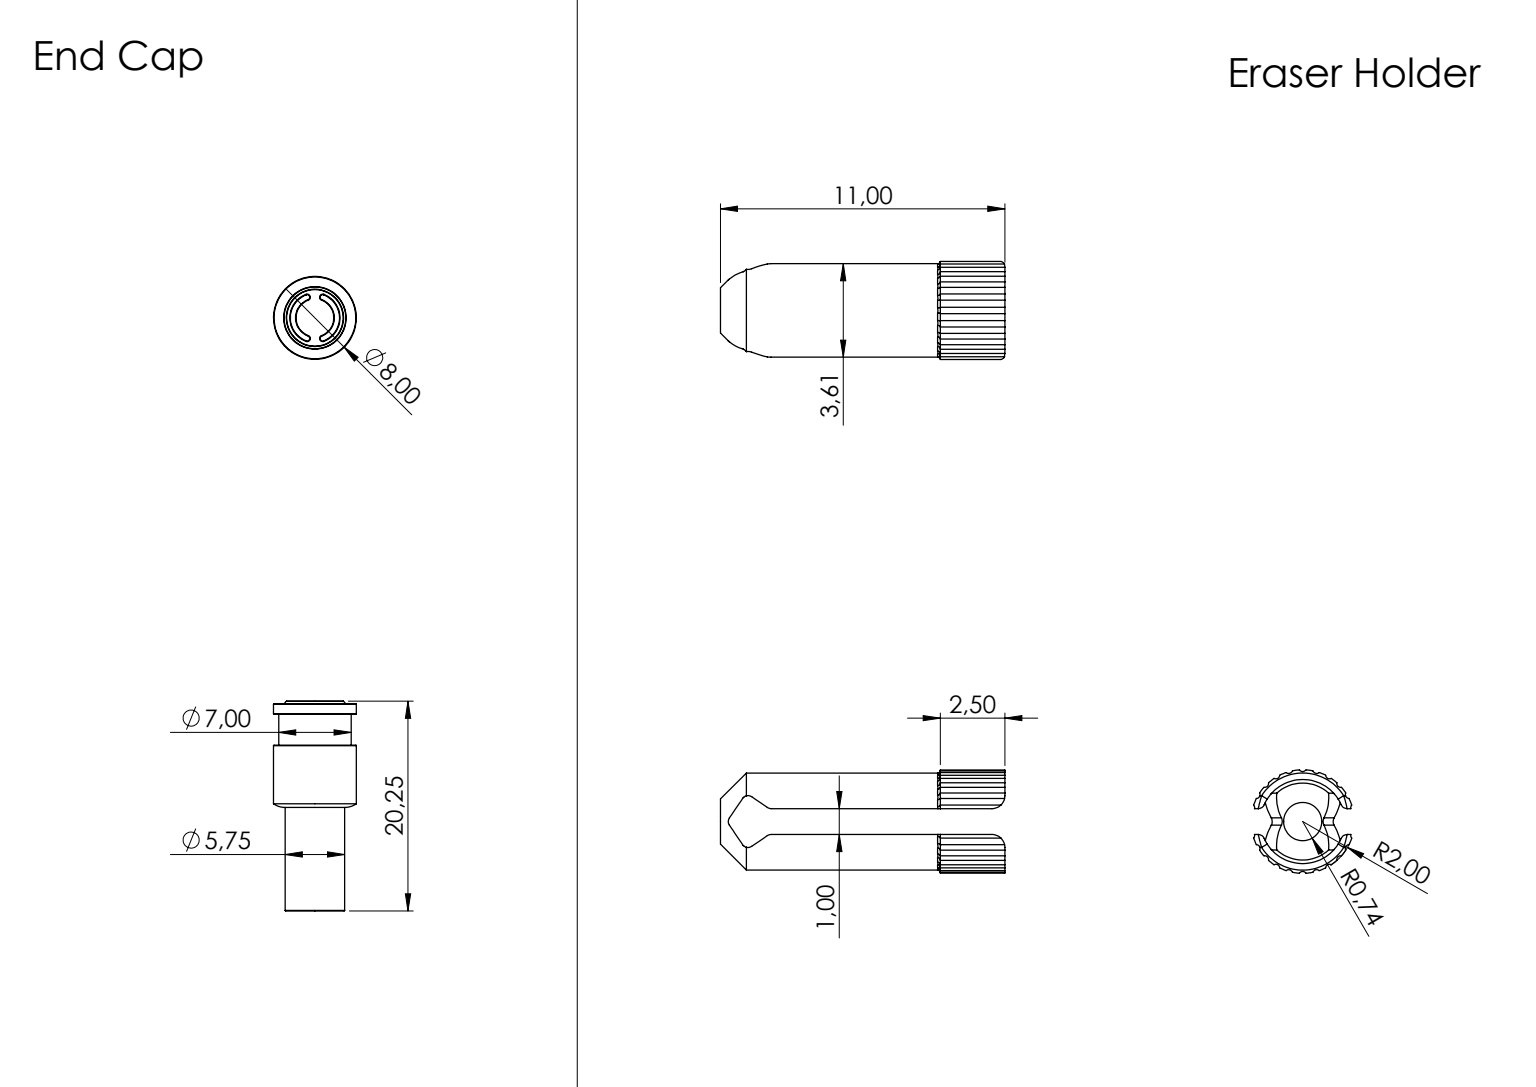
ISO-10303-21;
HEADER;
FILE_DESCRIPTION (('STEP AP214'),
    '1' );
FILE_NAME ('Eraser Holder.step',
    '2026-10-06T14:00:01',
    ( '' ),
    ( '' ),
    'SwSTEP 2.0',
    'SolidWorks 2020',
    '' );
FILE_SCHEMA (( 'AUTOMOTIVE_DESIGN' ));
ENDSEC;

DATA;
#15=CARTESIAN_POINT ( 'NONE',  ( 61.23770293223015670, -0.8897917884444476178, 1.791164585743103999 ) ) ;
#18=ORIENTED_EDGE ( 'NONE', *, *, #4179, .T. ) ;
#19=CARTESIAN_POINT ( 'NONE',  ( 58.72419296898095809, -1.822284191842195256, 0.4419487341019822102 ) ) ;
#25=ORIENTED_EDGE ( 'NONE', *, *, #30906, .F. ) ;
#36=VERTEX_POINT ( 'NONE', #5192 ) ;
#42=CARTESIAN_POINT ( 'NONE',  ( 60.81599023037216512, -0.4999999999993630651, -1.863080903343643291 ) ) ;
#52=ORIENTED_EDGE ( 'NONE', *, *, #16574, .F. ) ;
#60=DIRECTION ( 'NONE',  ( 1.000000000000000000, 1.047444401652940007E-14, -0.000000000000000000 ) ) ;
#62=EDGE_CURVE ( 'NONE', #4204, #12232, #6428, .T. ) ;
#67=VERTEX_POINT ( 'NONE', #29413 ) ;
#84=B_SPLINE_CURVE_WITH_KNOTS ( 'NONE', 3,
 ( #27085, #16988, #10017, #5408 ),
 .UNSPECIFIED., .F., .F.,
 ( 4, 4 ),
 ( 0.000000000000000000, 2.862003379465075675E-05 ),
 .UNSPECIFIED. ) ;
#90=CARTESIAN_POINT ( 'NONE',  ( 61.24891880570161362, -0.9671362613607715764, -1.669082548205986116 ) ) ;
#91=VERTEX_POINT ( 'NONE', #17714 ) ;
#93=VECTOR ( 'NONE', #18197, 1000.000000000000000 ) ;
#104=EDGE_LOOP ( 'NONE', ( #2125, #11645, #5974, #22411, #4642 ) ) ;
#118=CARTESIAN_POINT ( 'NONE',  ( 58.65817410504259044, 0.5270377936603326541, 1.799623063671935475 ) ) ;
#124=PLANE ( 'NONE',  #26575 ) ;
#126=CARTESIAN_POINT ( 'NONE',  ( 61.25000000000002132, 6.415596960124259844E-13, 3.111507638930570854E-58 ) ) ;
#136=CARTESIAN_POINT ( 'NONE',  ( 58.75000000000003553, -1.895722432252946010, 0.6373668173470157239 ) ) ;
#139=DIRECTION ( 'NONE',  ( 0.000000000000000000, 0.000000000000000000, 1.000000000000000000 ) ) ;
#145=CARTESIAN_POINT ( 'NONE',  ( 58.65000000000003411, -1.394635017527761311, -1.253243060177727131 ) ) ;
#162=CARTESIAN_POINT ( 'NONE',  ( 58.75000000000001421, 0.5933779550744251452, 1.867062706146590756 ) ) ;
#164=ORIENTED_EDGE ( 'NONE', *, *, #3455, .T. ) ;
#165=CARTESIAN_POINT ( 'NONE',  ( 58.75000018803721247, -1.882836145342761780, 0.4533061784681521322 ) ) ;
#166=LINE ( 'NONE', #7453, #15603 ) ;
#168=CARTESIAN_POINT ( 'NONE',  ( 51.64333574538936489, -0.8318165372340011743, -1.569663068107119974 ) ) ;
#173=CARTESIAN_POINT ( 'NONE',  ( 51.41326833096621129, -0.9846823677975790057, -1.426744987257088315 ) ) ;
#177=ORIENTED_EDGE ( 'NONE', *, *, #3546, .F. ) ;
#181=CARTESIAN_POINT ( 'NONE',  ( 58.74999999999980815, -1.394635017527639409, -1.253243060177863466 ) ) ;
#182=EDGE_CURVE ( 'NONE', #17885, #28405, #12945, .T. ) ;
#195=ORIENTED_EDGE ( 'NONE', *, *, #1967, .T. ) ;
#198=DIRECTION ( 'NONE',  ( 0.000000000000000000, 0.4531102586347437455, 0.8914544820235946743 ) ) ;
#203=VERTEX_POINT ( 'NONE', #8511 ) ;
#204=AXIS2_PLACEMENT_3D ( 'NONE', #12059, #22191, #17129 ) ;
#207=VERTEX_POINT ( 'NONE', #28132 ) ;
#212=B_SPLINE_CURVE_WITH_KNOTS ( 'NONE', 3,
 ( #23853, #28760, #23704, #11809, #1994, #9613, #29059, #26699, #21656, #24001, #19271, #11968, #26052 ),
 .UNSPECIFIED., .F., .F.,
 ( 4, 3, 3, 3, 4 ),
 ( 0.000000000000000000, 3.429247765843156239E-05, 6.861252194981137440E-05, 0.0001025118211733701013, 0.0001105094600589245180 ),
 .UNSPECIFIED. ) ;
#217=ADVANCED_FACE ( 'NONE', ( #691 ), #11323, .F. ) ;
#219=CIRCLE ( 'NONE', #12340, 2.000000000000000000 ) ;
#223=PLANE ( 'NONE',  #2312 ) ;
#224=CARTESIAN_POINT ( 'NONE',  ( 58.75000000000000000, 2.008165151418601191, 0.5380862305919300592 ) ) ;
#232=CARTESIAN_POINT ( 'NONE',  ( 58.66133336607628479, 1.875011749337246014, -0.03256983989501838900 ) ) ;
#233=DIRECTION ( 'NONE',  ( 1.000000000000000000, 1.047444401652940007E-14, 0.000000000000000000 ) ) ;
#238=FACE_OUTER_BOUND ( 'NONE', #13734, .T. ) ;
#243=AXIS2_PLACEMENT_3D ( 'NONE', #15272, #24917, #10208 ) ;
#245=AXIS2_PLACEMENT_3D ( 'NONE', #26689, #7358, #17036 ) ;
#249=DIRECTION ( 'NONE',  ( 1.000000000000000000, 1.047444401652940007E-14, 0.000000000000000000 ) ) ;
#262=PLANE ( 'NONE',  #2851 ) ;
#268=ORIENTED_EDGE ( 'NONE', *, *, #4535, .F. ) ;
#270=CARTESIAN_POINT ( 'NONE',  ( 51.50435016707359637, -0.9265794315402092751, -1.339215852266876672 ) ) ;
#272=VECTOR ( 'NONE', #16238, 1000.000000000000000 ) ;
#275=( BOUNDED_SURFACE ( )  B_SPLINE_SURFACE ( 3, 2, ( 
 ( #24839, #13578, #27853 ),
 ( #16132, #30851, #18355 ),
 ( #9002, #13880, #21051 ),
 ( #20886, #11544, #16291 ),
 ( #27992, #25934, #28322 ),
 ( #8822, #3767, #18511 ),
 ( #25783, #1876, #23266 ),
 ( #13729, #20588, #1550 ),
 ( #30222, #8528, #28153 ),
 ( #11213, #23111, #18831 ) ),
 .UNSPECIFIED., .F., .F., .T. ) 
 B_SPLINE_SURFACE_WITH_KNOTS ( ( 4, 2, 2, 2, 4 ),
 ( 3, 3 ),
 ( 0.0001706658715693258458, 0.0002229276920778027425, 0.0002751895125862796393, 0.0003274513330947565631, 0.0003797131536032334869 ),
 ( 0.000000000000000000, 1.000000000000000000 ),
 .UNSPECIFIED. ) 
 GEOMETRIC_REPRESENTATION_ITEM ( )  RATIONAL_B_SPLINE_SURFACE ( (
 ( 1.000000000000000000, 0.7071067811865444641, 1.000000000000000000),
 ( 1.000000000000000000, 0.7375607040701035455, 1.000000000000000000),
 ( 1.000000000000000000, 0.7730431127426561355, 1.000000000000000000),
 ( 1.000000000000000000, 0.8321012486983990764, 1.000000000000000000),
 ( 1.000000000000000000, 0.8541932017405543531, 1.000000000000000000),
 ( 1.000000000000000000, 0.8545723906055556762, 1.000000000000000000),
 ( 1.000000000000000000, 0.8327032135045047134, 1.000000000000000000),
 ( 1.000000000000000000, 0.7734559727062164658, 1.000000000000000000),
 ( 1.000000000000000000, 0.7377766653995503354, 1.000000000000000000),
 ( 1.000000000000000000, 0.7071067811865452413, 1.000000000000000000) ) ) 
 REPRESENTATION_ITEM ( '' )  SURFACE ( )  );
#276=ORIENTED_EDGE ( 'NONE', *, *, #13970, .F. ) ;
#283=DIRECTION ( 'NONE',  ( 0.000000000000000000, 0.9985773570672645816, 0.05332224631949589871 ) ) ;
#284=ADVANCED_FACE ( 'NONE', ( #30591 ), #18007, .F. ) ;
#286=CARTESIAN_POINT ( 'NONE',  ( 50.25000000000002132, 5.263408118306026973E-13, 3.111507638930570854E-58 ) ) ;
#295=CARTESIAN_POINT ( 'NONE',  ( 58.75000000000003553, -1.655311165516605509, -1.077297519404007753 ) ) ;
#297=ORIENTED_EDGE ( 'NONE', *, *, #11149, .T. ) ;
#299=AXIS2_PLACEMENT_3D ( 'NONE', #16364, #4639, #26010 ) ;
#310=CARTESIAN_POINT ( 'NONE',  ( 58.72427158855736451, -1.798991944511769470, 0.5288318043114524913 ) ) ;
#311=AXIS2_PLACEMENT_3D ( 'NONE', #27449, #5763, #15416 ) ;
#314=FACE_OUTER_BOUND ( 'NONE', #22953, .T. ) ;
#316=CARTESIAN_POINT ( 'NONE',  ( 58.74472430272383150, -0.4999999999993849364, -1.853787220596752272 ) ) ;
#321=CARTESIAN_POINT ( 'NONE',  ( 51.78416995154975666, -0.8999235898776958287, -1.360374659026170718 ) ) ;
#322=AXIS2_PLACEMENT_3D ( 'NONE', #6296, #16124, #30840 ) ;
#335=CIRCLE ( 'NONE', #10516, 1.875000000000001776 ) ;
#345=CIRCLE ( 'NONE', #29674, 0.1500000000000001887 ) ;
#346=CARTESIAN_POINT ( 'NONE',  ( 58.66133336607573057, -1.802692578418147118, 0.5167488000325648478 ) ) ;
#359=CIRCLE ( 'NONE', #3392, 1.975000000000001865 ) ;
#360=DIRECTION ( 'NONE',  ( 1.000000000000000000, 1.047444401652940007E-14, 0.000000000000000000 ) ) ;
#366=ORIENTED_EDGE ( 'NONE', *, *, #22608, .F. ) ;
#367=DIRECTION ( 'NONE',  ( 1.000000000000000000, 1.047444401652940007E-14, 0.000000000000000000 ) ) ;
#370=ADVANCED_FACE ( 'NONE', ( #29150 ), #19356, .F. ) ;
#379=AXIS2_PLACEMENT_3D ( 'NONE', #22161, #7586, #5825 ) ;
#382=ORIENTED_EDGE ( 'NONE', *, *, #29422, .T. ) ;
#383=CARTESIAN_POINT ( 'NONE',  ( 51.89360908398760586, 0.6611756245550776123, -1.497563819580874922 ) ) ;
#385=CARTESIAN_POINT ( 'NONE',  ( 58.72427158855720819, -0.9764256747734804120, -1.600821037878335185 ) ) ;
#388=CARTESIAN_POINT ( 'NONE',  ( 51.18802626461298644, 0.9696678249730820154, 1.452003249885708946 ) ) ;
#389=CIRCLE ( 'NONE', #18100, 0.1000000000000000749 ) ;
#392=CARTESIAN_POINT ( 'NONE',  ( 58.75000000000002842, -1.077297519403676906, 1.655311165517035166 ) ) ;
#394=CARTESIAN_POINT ( 'NONE',  ( 51.17290532404582137, 0.9646187004851747293, 1.462925393634774363 ) ) ;
#398=CARTESIAN_POINT ( 'NONE',  ( 61.24637336955063915, -0.9388313581414567954, -1.688008567904763835 ) ) ;
#401=ORIENTED_EDGE ( 'NONE', *, *, #30815, .F. ) ;
#406=DIRECTION ( 'NONE',  ( 1.000000000000000000, 1.047444401652940007E-14, 0.000000000000000000 ) ) ;
#408=ORIENTED_EDGE ( 'NONE', *, *, #18853, .F. ) ;
#414=CIRCLE ( 'NONE', #1347, 1.875000000000001776 ) ;
#423=CARTESIAN_POINT ( 'NONE',  ( 51.45655683570189609, 0.9591657938401617622, -1.518428463906025705 ) ) ;
#425=AXIS2_PLACEMENT_3D ( 'NONE', #10899, #22657, #18053 ) ;
#431=LINE ( 'NONE', #17079, #18420 ) ;
#436=ORIENTED_EDGE ( 'NONE', *, *, #1318, .F. ) ;
#442=CARTESIAN_POINT ( 'NONE',  ( 58.75000000000001421, 0.5380862305905714793, 2.008165151419250449 ) ) ;
#443=ADVANCED_FACE ( 'NONE', ( #24852 ), #20138, .T. ) ;
#445=DIRECTION ( 'NONE',  ( -1.000000000000000000, -1.047444401652940007E-14, -0.000000000000000000 ) ) ;
#456=CARTESIAN_POINT ( 'NONE',  ( 51.84831113588977303, -0.6920605891655385866, -1.653603923793142361 ) ) ;
#457=ORIENTED_EDGE ( 'NONE', *, *, #26462, .T. ) ;
#465=EDGE_LOOP ( 'NONE', ( #3537, #28913, #30616, #5077 ) ) ;
#466=CIRCLE ( 'NONE', #9064, 0.1499999999999998557 ) ;
#477=CARTESIAN_POINT ( 'NONE',  ( 58.75000000000002132, 6.153735859711025284E-13, 3.111507638930570854E-58 ) ) ;
#482=ORIENTED_EDGE ( 'NONE', *, *, #30906, .T. ) ;
#490=CIRCLE ( 'NONE', #22257, 2.000000000000000000 ) ;
#493=DIRECTION ( 'NONE',  ( 1.000000000000000000, 1.047444401652940007E-14, 0.000000000000000000 ) ) ;
#507=VERTEX_POINT ( 'NONE', #5861 ) ;
#511=CARTESIAN_POINT ( 'NONE',  ( 50.25000000000002842, -0.6373668173474561494, 1.895722432253304168 ) ) ;
#521=ORIENTED_EDGE ( 'NONE', *, *, #12297, .F. ) ;
#528=DIRECTION ( 'NONE',  ( 0.000000000000000000, 0.000000000000000000, 1.000000000000000000 ) ) ;
#535=CARTESIAN_POINT ( 'NONE',  ( 61.25000000000004263, -1.960427193528290424, -0.3958853607747112036 ) ) ;
#543=DIRECTION ( 'NONE',  ( 1.000000000000000000, 1.047444401652940007E-14, 0.000000000000000000 ) ) ;
#545=CARTESIAN_POINT ( 'NONE',  ( 58.72427158855708029, 1.293556822995456823, -1.357477749119827104 ) ) ;
#555=EDGE_LOOP ( 'NONE', ( #4647, #4798, #8077, #13774 ) ) ;
#574=DIRECTION ( 'NONE',  ( 0.000000000000000000, -1.154631945610163433E-14, 1.000000000000000000 ) ) ;
#575=DIRECTION ( 'NONE',  ( 1.000000000000000000, 1.047444401652940007E-14, 0.000000000000000000 ) ) ;
#585=VERTEX_POINT ( 'NONE', #11859 ) ;
#589=CARTESIAN_POINT ( 'NONE',  ( 51.23644008536124517, -1.080112125195908490, -1.214076932077872817 ) ) ;
#593=CIRCLE ( 'NONE', #14742, 0.09999999999999990841 ) ;
#595=CARTESIAN_POINT ( 'NONE',  ( 58.75000000000002132, 6.153735859711025284E-13, 3.111507638930570854E-58 ) ) ;
#599=ADVANCED_FACE ( 'NONE', ( #18369 ), #26110, .T. ) ;
#606=CARTESIAN_POINT ( 'NONE',  ( 52.06628335902946247, -0.5434431642975662280, -1.718465885608440713 ) ) ;
#620=CARTESIAN_POINT ( 'NONE',  ( 58.75000000000002132, 6.153735859711025284E-13, 3.111507638930570854E-58 ) ) ;
#624=VERTEX_POINT ( 'NONE', #28172 ) ;
#627=CYLINDRICAL_SURFACE ( 'NONE', #1476, 2.000000000000000000 ) ;
#628=ORIENTED_EDGE ( 'NONE', *, *, #25092, .T. ) ;
#631=DIRECTION ( 'NONE',  ( 0.000000000000000000, 0.000000000000000000, 1.000000000000000000 ) ) ;
#672=ORIENTED_EDGE ( 'NONE', *, *, #29291, .F. ) ;
#675=VECTOR ( 'NONE', #28976, 1000.000000000000000 ) ;
#691=FACE_OUTER_BOUND ( 'NONE', #7612, .T. ) ;
#695=CARTESIAN_POINT ( 'NONE',  ( 52.20711756518983293, 0.5000000000005468959, 1.807104036850122109 ) ) ;
#698=ORIENTED_EDGE ( 'NONE', *, *, #22851, .F. ) ;
#704=VERTEX_POINT ( 'NONE', #19468 ) ;
#716=AXIS2_PLACEMENT_3D ( 'NONE', #28481, #23120, #1884 ) ;
#719=B_SPLINE_CURVE_WITH_KNOTS ( 'NONE', 3,
 ( #22326, #2999, #17256, #24068, #2383, #12047, #21722, #16951, #26898, #14858, #7446, #7736, #15 ),
 .UNSPECIFIED., .F., .F.,
 ( 4, 3, 3, 3, 4 ),
 ( 0.000000000000000000, 4.969793434219683530E-05, 9.932084631989379544E-05, 0.0001499488332825447262, 0.0001857305951747128983 ),
 .UNSPECIFIED. ) ;
#755=CARTESIAN_POINT ( 'NONE',  ( 58.74999981404332061, 1.649595783783479375, -1.050697058760609037 ) ) ;
#756=DIRECTION ( 'NONE',  ( -0.000000000000000000, -0.000000000000000000, 1.000000000000000000 ) ) ;
#760=AXIS2_PLACEMENT_3D ( 'NONE', #23917, #2210, #11875 ) ;
#764=CARTESIAN_POINT ( 'NONE',  ( 50.25000000000001421, 0.5380862305914526633, -2.008165151417984351 ) ) ;
#771=EDGE_CURVE ( 'NONE', #11615, #8275, #12629, .T. ) ;
#773=DIRECTION ( 'NONE',  ( 0.000000000000000000, 0.000000000000000000, 1.000000000000000000 ) ) ;
#779=VERTEX_POINT ( 'NONE', #24051 ) ;
#783=VECTOR ( 'NONE', #2254, 1000.000000000000000 ) ;
#793=B_SPLINE_CURVE_WITH_KNOTS ( 'NONE', 3,
 ( #2578, #2877, #7631, #19681 ),
 .UNSPECIFIED., .F., .F.,
 ( 4, 4 ),
 ( 0.0001543670095910078732, 0.0003084486524517373977 ),
 .UNSPECIFIED. ) ;
#797=B_SPLINE_CURVE_WITH_KNOTS ( 'NONE', 3,
 ( #20697, #30322, #12903, #18305 ),
 .UNSPECIFIED., .F., .F.,
 ( 4, 4 ),
 ( 0.000000000000000000, 0.0003819718307412704175 ),
 .UNSPECIFIED. ) ;
#798=ORIENTED_EDGE ( 'NONE', *, *, #29211, .T. ) ;
#803=CIRCLE ( 'NONE', #9900, 0.1500000000000001887 ) ;
#805=DIRECTION ( 'NONE',  ( 0.000000000000000000, 1.000000000000000000, 0.000000000000000000 ) ) ;
#806=DIRECTION ( 'NONE',  ( 0.000000000000000000, 0.000000000000000000, 1.000000000000000000 ) ) ;
#810=CIRCLE ( 'NONE', #6376, 1.975000000000001865 ) ;
#822=ORIENTED_EDGE ( 'NONE', *, *, #25663, .T. ) ;
#823=CARTESIAN_POINT ( 'NONE',  ( 51.25000000000000711, 1.487500000000537836, 3.111507638930570854E-58 ) ) ;
#833=VERTEX_POINT ( 'NONE', #5999 ) ;
#835=ADVANCED_FACE ( 'NONE', ( #6144 ), #29926, .F. ) ;
#847=CIRCLE ( 'NONE', #15519, 0.1499999999999999667 ) ;
#848=CARTESIAN_POINT ( 'NONE',  ( 58.75000000000001421, 0.5811678240991637878, -1.782657835994492013 ) ) ;
#849=CYLINDRICAL_SURFACE ( 'NONE', #29409, 0.1499999999999999667 ) ;
#852=DIRECTION ( 'NONE',  ( 1.000000000000000000, 1.047444401652940007E-14, 0.000000000000000000 ) ) ;
#858=DIRECTION ( 'NONE',  ( 0.000000000000000000, 0.000000000000000000, 1.000000000000000000 ) ) ;
#861=CARTESIAN_POINT ( 'NONE',  ( 58.75000000000000711, 1.469015551797813846, -1.320082690053157037 ) ) ;
#869=CIRCLE ( 'NONE', #6936, 0.1500000000000001887 ) ;
#870=ORIENTED_EDGE ( 'NONE', *, *, #20028, .T. ) ;
#872=CIRCLE ( 'NONE', #8460, 1.975000000000001865 ) ;
#882=CARTESIAN_POINT ( 'NONE',  ( 51.59739104186226655, 1.010292945603182391, -1.272765950230260179 ) ) ;
#892=ADVANCED_FACE ( 'NONE', ( #25917 ), #30664, .F. ) ;
#906=ADVANCED_FACE ( 'NONE', ( #23399 ), #24657, .F. ) ;
#909=EDGE_CURVE ( 'NONE', #14419, #20284, #9225, .T. ) ;
#911=CARTESIAN_POINT ( 'NONE',  ( 50.56925576102500486, 0.1015751161705248512, 0.8011113709441619601 ) ) ;
#917=CARTESIAN_POINT ( 'NONE',  ( 58.75000000000001421, 0.5380862305905714793, 2.008165151419250449 ) ) ;
#919=CARTESIAN_POINT ( 'NONE',  ( 58.65000000000001990, 6.143261415694495821E-13, 3.111507638930570854E-58 ) ) ;
#923=ADVANCED_FACE ( 'NONE', ( #2011 ), #8804, .F. ) ;
#925=CARTESIAN_POINT ( 'NONE',  ( 58.65000000000001990, 6.143261415694495821E-13, 3.111507638930570854E-58 ) ) ;
#934=CARTESIAN_POINT ( 'NONE',  ( 51.64281244548085681, -0.8321733326261643304, 1.569379851958366601 ) ) ;
#935=EDGE_CURVE ( 'NONE', #17628, #18608, #7028, .T. ) ;
#939=ADVANCED_FACE ( 'NONE', ( #28303 ), #31138, .F. ) ;
#951=CARTESIAN_POINT ( 'NONE',  ( 51.12687253673781385, -0.9194130538815391551, 1.491219977510798600 ) ) ;
#954=ORIENTED_EDGE ( 'NONE', *, *, #13577, .T. ) ;
#957=MECHANICAL_DESIGN_GEOMETRIC_PRESENTATION_REPRESENTATION('',(#11070),#9033);
#967=EDGE_CURVE ( 'NONE', #12164, #18852, #27400, .T. ) ;
#978=CARTESIAN_POINT ( 'NONE',  ( 58.74999999305998699, -1.869977652031123094, -0.4744892162740728669 ) ) ;
#986=AXIS2_PLACEMENT_3D ( 'NONE', #6730, #26038, #21171 ) ;
#989=CARTESIAN_POINT ( 'NONE',  ( 58.75000000000000711, 1.039502773797200019, -1.800471618823823450 ) ) ;
#990=EDGE_LOOP ( 'NONE', ( #18643, #27738, #24622, #5621, #14527, #4921 ) ) ;
#993=CIRCLE ( 'NONE', #14134, 0.1000000000000000611 ) ;
#996=EDGE_LOOP ( 'NONE', ( #25581, #2177, #9610, #14667, #5663, #17467 ) ) ;
#997=CARTESIAN_POINT ( 'NONE',  ( 58.75000000000000711, 1.039502773796331159, 1.800471618825331355 ) ) ;
#998=CARTESIAN_POINT ( 'NONE',  ( 51.36308620441097617, 1.097739233406260118, -1.198394850649635357 ) ) ;
#1013=FACE_OUTER_BOUND ( 'NONE', #20174, .T. ) ;
#1014=CARTESIAN_POINT ( 'NONE',  ( 50.25000000000000000, 1.800471618824854181, -1.039502773795712987 ) ) ;
#1015=DIRECTION ( 'NONE',  ( 1.000000000000000000, 1.047444401652940007E-14, 0.000000000000000000 ) ) ;
#1016=CARTESIAN_POINT ( 'NONE',  ( 51.25000000000001421, 5.368152558471320595E-13, 3.111507638930570854E-58 ) ) ;
#1018=DIRECTION ( 'NONE',  ( -0.5633368246414943714, -0.8262273428075581627, 0.000000000000000000 ) ) ;
#1024=AXIS2_PLACEMENT_3D ( 'NONE', #23682, #18298, #6253 ) ;
#1030=CARTESIAN_POINT ( 'NONE',  ( 61.00000000000002132, 6.389410850082937196E-13, 3.111507638930570854E-58 ) ) ;
#1037=VERTEX_POINT ( 'NONE', #24332 ) ;
#1048=AXIS2_PLACEMENT_3D ( 'NONE', #10585, #8052, #2989 ) ;
#1050=DIRECTION ( 'NONE',  ( 1.000000000000000000, 1.047444401652940007E-14, 0.000000000000000000 ) ) ;
#1054=CARTESIAN_POINT ( 'NONE',  ( 51.25000000000001421, 5.368152558471320595E-13, 3.111507638930570854E-58 ) ) ;
#1058=CARTESIAN_POINT ( 'NONE',  ( 58.65000000000000568, 1.571497941946485177, 1.022750809562084306 ) ) ;
#1061=FACE_OUTER_BOUND ( 'NONE', #19043, .T. ) ;
#1062=ORIENTED_EDGE ( 'NONE', *, *, #27891, .F. ) ;
#1063=CARTESIAN_POINT ( 'NONE',  ( 58.75000000000000711, 1.932246131438033920, -0.4087173687832938995 ) ) ;
#1066=DIRECTION ( 'NONE',  ( -1.018631342913014973E-14, 1.000000000000000000, 0.000000000000000000 ) ) ;
#1067=DIRECTION ( 'NONE',  ( 0.000000000000000000, 0.000000000000000000, 1.000000000000000000 ) ) ;
#1072=CARTESIAN_POINT ( 'NONE',  ( 51.31572262954152563, 0.7526089581382734428, -1.996089927833914146 ) ) ;
#1075=DIRECTION ( 'NONE',  ( -0.8262273428075537218, 0.5633368246415009217, 0.000000000000000000 ) ) ;
#1079=FACE_OUTER_BOUND ( 'NONE', #31118, .T. ) ;
#1081=CARTESIAN_POINT ( 'NONE',  ( 51.84831113588978724, -0.6920605891655307040, 1.653603923793091068 ) ) ;
#1083=VERTEX_POINT ( 'NONE', #20221 ) ;
#1091=CARTESIAN_POINT ( 'NONE',  ( 58.75000000000002132, -0.4999999999991334154, 1.863080903344709549 ) ) ;
#1107=CARTESIAN_POINT ( 'NONE',  ( 58.74160516400056053, 1.017053542743361794, 1.575205926126844513 ) ) ;
#1114=ADVANCED_FACE ( 'NONE', ( #10373 ), #27630, .F. ) ;
#1121=DIRECTION ( 'NONE',  ( 1.000000000000000000, 1.047444401652940007E-14, 0.000000000000000000 ) ) ;
#1124=CARTESIAN_POINT ( 'NONE',  ( 58.75000000000003553, -1.760622601995984304, -0.8948927608036236769 ) ) ;
#1135=ORIENTED_EDGE ( 'NONE', *, *, #4031, .F. ) ;
#1138=ORIENTED_EDGE ( 'NONE', *, *, #28214, .F. ) ;
#1143=CARTESIAN_POINT ( 'NONE',  ( 58.64999999999999858, 1.671477153795419390, -0.8495817349390374362 ) ) ;
#1144=EDGE_LOOP ( 'NONE', ( #6591, #9871, #26617, #31163 ) ) ;
#1152=CARTESIAN_POINT ( 'NONE',  ( 61.20598745287978915, 0.7563774268569909420, 1.657497327209963345 ) ) ;
#1154=AXIS2_PLACEMENT_3D ( 'NONE', #9213, #7572, #17089 ) ;
#1164=ORIENTED_EDGE ( 'NONE', *, *, #8587, .T. ) ;
#1165=CARTESIAN_POINT ( 'NONE',  ( 51.98855675296391610, 0.7791495708613138671, -1.432971607104406520 ) ) ;
#1192=FACE_OUTER_BOUND ( 'NONE', #13084, .T. ) ;
#1196=DIRECTION ( 'NONE',  ( 1.000000000000000000, 1.047444401652940007E-14, 0.000000000000000000 ) ) ;
#1200=EDGE_LOOP ( 'NONE', ( #2742, #18519, #13836, #1367 ) ) ;
#1201=ADVANCED_FACE ( 'NONE', ( #11638 ), #13817, .T. ) ;
#1211=DIRECTION ( 'NONE',  ( 0.000000000000000000, 0.000000000000000000, -1.000000000000000000 ) ) ;
#1216=CARTESIAN_POINT ( 'NONE',  ( 58.73371041428912065, 1.662559130999850865, -0.8671977075788435130 ) ) ;
#1249=( BOUNDED_CURVE ( )  B_SPLINE_CURVE ( 3, ( #3855, #13504, #1165, #10822 ),
 .UNSPECIFIED., .F., .T. ) 
 B_SPLINE_CURVE_WITH_KNOTS ( ( 4, 4 ),
 ( 4.041453792691655167, 4.300872134317202722 ),
 .UNSPECIFIED. ) 
 CURVE ( )  GEOMETRIC_REPRESENTATION_ITEM ( )  RATIONAL_B_SPLINE_CURVE ( ( 1.000000000000000000, 0.9943997021150918769, 0.9943997021150918769, 1.000000000000000000 ) ) 
 REPRESENTATION_ITEM ( '' )  );
#1256=VERTEX_POINT ( 'NONE', #25406 ) ;
#1266=CARTESIAN_POINT ( 'NONE',  ( 58.64999999999999147, 1.827485639843792864, -0.4207625006677218060 ) ) ;
#1268=AXIS2_PLACEMENT_3D ( 'NONE', #6662, #6195, #11578 ) ;
#1269=ORIENTED_EDGE ( 'NONE', *, *, #8234, .T. ) ;
#1273=DIRECTION ( 'NONE',  ( 0.000000000000000000, 0.000000000000000000, 1.000000000000000000 ) ) ;
#1276=CARTESIAN_POINT ( 'NONE',  ( 61.25000000000000711, 1.499837071477986505, 1.323060376182421782 ) ) ;
#1288=CARTESIAN_POINT ( 'NONE',  ( 51.23644008536124517, -1.080112125195908490, -1.214076932077872817 ) ) ;
#1298=AXIS2_PLACEMENT_3D ( 'NONE', #4590, #28822, #21869 ) ;
#1300=CARTESIAN_POINT ( 'NONE',  ( 58.75000002382379449, 0.5510104498278126650, -1.849358057801673505 ) ) ;
#1301=CARTESIAN_POINT ( 'NONE',  ( 58.64999999999999147, 1.589751505945893095, 0.9947034709630272475 ) ) ;
#1313=CIRCLE ( 'NONE', #15983, 0.1000000000000000611 ) ;
#1316=ORIENTED_EDGE ( 'NONE', *, *, #1533, .F. ) ;
#1318=EDGE_CURVE ( 'NONE', #3662, #19841, #3554, .T. ) ;
#1320=FACE_OUTER_BOUND ( 'NONE', #25481, .T. ) ;
#1332=ORIENTED_EDGE ( 'NONE', *, *, #26822, .F. ) ;
#1333=AXIS2_PLACEMENT_3D ( 'NONE', #25103, #29529, #2954 ) ;
#1335=DIRECTION ( 'NONE',  ( 0.000000000000000000, 0.000000000000000000, 1.000000000000000000 ) ) ;
#1336=VERTEX_POINT ( 'NONE', #15758 ) ;
#1337=CARTESIAN_POINT ( 'NONE',  ( 61.09423418603945777, 0.6373668173466511266, 1.895722432253563516 ) ) ;
#1341=CARTESIAN_POINT ( 'NONE',  ( 51.89360908398611372, -0.6611756245528535025, -1.497563819582787614 ) ) ;
#1347=AXIS2_PLACEMENT_3D ( 'NONE', #24122, #26652, #2730 ) ;
#1349=CARTESIAN_POINT ( 'NONE',  ( 61.25000000000004263, -1.996089927834276301, 0.1250000000000018041 ) ) ;
#1352=CARTESIAN_POINT ( 'NONE',  ( 58.65000090395038512, -0.5493607500713694192, 1.793027323413614038 ) ) ;
#1356=AXIS2_PLACEMENT_3D ( 'NONE', #5359, #7596, #14714 ) ;
#1358=DIRECTION ( 'NONE',  ( 0.000000000000000000, 0.000000000000000000, -1.000000000000000000 ) ) ;
#1362=ORIENTED_EDGE ( 'NONE', *, *, #12297, .T. ) ;
#1364=EDGE_LOOP ( 'NONE', ( #23271, #3401, #8925, #4713 ) ) ;
#1367=ORIENTED_EDGE ( 'NONE', *, *, #7484, .F. ) ;
#1370=CARTESIAN_POINT ( 'NONE',  ( 60.87284881435256523, -0.5000000998561487942, 1.554802432719775362 ) ) ;
#1372=CIRCLE ( 'NONE', #30683, 0.1500000000000001887 ) ;
#1382=VERTEX_POINT ( 'NONE', #16713 ) ;
#1384=CARTESIAN_POINT ( 'NONE',  ( 58.75000000000000000, 1.871971993775707555, -0.6020210199447628696 ) ) ;
#1394=AXIS2_PLACEMENT_3D ( 'NONE', #286, #17550, #5511 ) ;
#1395=CIRCLE ( 'NONE', #10003, 0.1500000000000001887 ) ;
#1397=CARTESIAN_POINT ( 'NONE',  ( 61.09423418603945777, 0.6373668173466511266, 1.895722432253563516 ) ) ;
#1399=CARTESIAN_POINT ( 'NONE',  ( 58.66118217212479635, -1.874997884618849753, 0.01689491344058241529 ) ) ;
#1401=ORIENTED_EDGE ( 'NONE', *, *, #26434, .T. ) ;
#1405=CARTESIAN_POINT ( 'NONE',  ( 51.64837794009022076, -0.8283786772106969121, 1.688958810662479104 ) ) ;
#1407=CARTESIAN_POINT ( 'NONE',  ( 58.65000000000001990, 6.143261415694495821E-13, 3.111507638930570854E-58 ) ) ;
#1421=ORIENTED_EDGE ( 'NONE', *, *, #10213, .T. ) ;
#1431=CARTESIAN_POINT ( 'NONE',  ( 58.65000000000001990, 6.143261415694495821E-13, 3.111507638930570854E-58 ) ) ;
#1433=ORIENTED_EDGE ( 'NONE', *, *, #16160, .F. ) ;
#1435=CARTESIAN_POINT ( 'NONE',  ( 61.25000000000003553, -0.9999999999993586242, -1.586072192556190252 ) ) ;
#1436=( BOUNDED_SURFACE ( )  B_SPLINE_SURFACE ( 3, 2, ( 
 ( #15821, #3492, #3779 ),
 ( #13130, #1107, #22819 ),
 ( #21701, #26269, #23426 ),
 ( #18997, #4575, #30704 ),
 ( #12024, #14223, #21384 ),
 ( #26421, #16926, #31172 ),
 ( #9660, #23749, #4717 ),
 ( #14374, #23897, #30863 ),
 ( #21230, #14067, #31008 ),
 ( #19167, #7258, #2189 ) ),
 .UNSPECIFIED., .F., .F., .F. ) 
 B_SPLINE_SURFACE_WITH_KNOTS ( ( 4, 2, 2, 2, 4 ),
 ( 3, 3 ),
 ( 0.0001706658715694773631, 0.0002229276920777904640, 0.0002751895125861035648, 0.0003274513330944167199, 0.0003797131536027298208 ),
 ( 0.000000000000000000, 1.000000000000000000 ),
 .UNSPECIFIED. ) 
 GEOMETRIC_REPRESENTATION_ITEM ( )  RATIONAL_B_SPLINE_SURFACE ( (
 ( 1.000000000000000000, 0.7071067811865445751, 1.000000000000000000),
 ( 1.000000000000000000, 0.7375607040698810568, 1.000000000000000000),
 ( 1.000000000000000000, 0.7730431127426297122, 1.000000000000000000),
 ( 1.000000000000000000, 0.8321012486974134204, 1.000000000000000000),
 ( 1.000000000000000000, 0.8541932017392805943, 1.000000000000000000),
 ( 1.000000000000000000, 0.8545723906046818197, 1.000000000000000000),
 ( 1.000000000000000000, 0.8327032135036619431, 1.000000000000000000),
 ( 1.000000000000000000, 0.7734559727059460155, 1.000000000000000000),
 ( 1.000000000000000000, 0.7377766653993722556, 1.000000000000000000),
 ( 1.000000000000000000, 0.7071067811865451302, 1.000000000000000000) ) ) 
 REPRESENTATION_ITEM ( '' )  SURFACE ( )  );
#1443=CARTESIAN_POINT ( 'NONE',  ( 51.12687253673781385, -0.9194130538815391551, -1.491219977510798600 ) ) ;
#1448=ORIENTED_EDGE ( 'NONE', *, *, #2643, .F. ) ;
#1468=CIRCLE ( 'NONE', #23234, 1.975000000000001865 ) ;
#1472=CARTESIAN_POINT ( 'NONE',  ( 58.75000000000003553, -1.760622601995690983, -0.8948927608037045012 ) ) ;
#1476=AXIS2_PLACEMENT_3D ( 'NONE', #477, #10141, #11927 ) ;
#1478=VERTEX_POINT ( 'NONE', #4584 ) ;
#1480=DIRECTION ( 'NONE',  ( 0.000000000000000000, 0.000000000000000000, 1.000000000000000000 ) ) ;
#1484=CARTESIAN_POINT ( 'NONE',  ( 51.25000000000001421, 0.9938153758931693726, 1.589954715908409755 ) ) ;
#1487=CARTESIAN_POINT ( 'NONE',  ( 58.75000000000002132, 6.153735859711025284E-13, 3.111507638930570854E-58 ) ) ;
#1503=DIRECTION ( 'NONE',  ( 1.000000000000000000, 1.047444401652940007E-14, 0.000000000000000000 ) ) ;
#1505=EDGE_CURVE ( 'NONE', #16552, #4296, #28743, .T. ) ;
#1509=DIRECTION ( 'NONE',  ( 1.000000000000000000, 1.047444401652940007E-14, 0.000000000000000000 ) ) ;
#1523=CARTESIAN_POINT ( 'NONE',  ( 60.75000000000003553, -0.6499999999993626432, 1.489337100860685270 ) ) ;
#1525=ORIENTED_EDGE ( 'NONE', *, *, #13910, .F. ) ;
#1531=FACE_OUTER_BOUND ( 'NONE', #4571, .T. ) ;
#1532=CYLINDRICAL_SURFACE ( 'NONE', #17592, 0.2500000000000000000 ) ;
#1533=EDGE_CURVE ( 'NONE', #10001, #12097, #20968, .T. ) ;
#1537=CARTESIAN_POINT ( 'NONE',  ( 58.74999981404330640, 1.865327579934561664, -0.5879486190987924799 ) ) ;
#1542=PLANE ( 'NONE',  #8402 ) ;
#1550=CARTESIAN_POINT ( 'NONE',  ( 58.65266784251152643, 1.589569034372934730, 0.9945725797258593293 ) ) ;
#1551=ORIENTED_EDGE ( 'NONE', *, *, #3019, .F. ) ;
#1574=CARTESIAN_POINT ( 'NONE',  ( 61.23913277633455721, 0.8963220027434347648, -1.755758457445524279 ) ) ;
#1575=CARTESIAN_POINT ( 'NONE',  ( 61.25000000000004263, -2.008165151418346728, -0.5380862305909229759 ) ) ;
#1578=DIRECTION ( 'NONE',  ( 0.000000000000000000, 0.000000000000000000, 1.000000000000000000 ) ) ;
#1582=CARTESIAN_POINT ( 'NONE',  ( 50.25000000000004263, -1.960427193528665679, 0.3958853607747486181 ) ) ;
#1586=CARTESIAN_POINT ( 'NONE',  ( 58.65838214097832548, 1.819565423307722973, 0.4528606663879586880 ) ) ;
#1594=DIRECTION ( 'NONE',  ( 0.000000000000000000, 0.000000000000000000, 1.000000000000000000 ) ) ;
#1598=ORIENTED_EDGE ( 'NONE', *, *, #27228, .F. ) ;
#1603=ORIENTED_EDGE ( 'NONE', *, *, #30308, .T. ) ;
#1609=DIRECTION ( 'NONE',  ( 0.000000000000000000, 0.000000000000000000, 1.000000000000000000 ) ) ;
#1620=ORIENTED_EDGE ( 'NONE', *, *, #27872, .T. ) ;
#1625=ORIENTED_EDGE ( 'NONE', *, *, #27794, .F. ) ;
#1629=ORIENTED_EDGE ( 'NONE', *, *, #2077, .F. ) ;
#1633=CARTESIAN_POINT ( 'NONE',  ( 51.31943556899493331, 1.088761256244167086, -1.206353010735628395 ) ) ;
#1640=EDGE_LOOP ( 'NONE', ( #23576, #7511, #21638, #13636 ) ) ;
#1649=CARTESIAN_POINT ( 'NONE',  ( 58.73307976133193620, -0.5681412931372339381, 1.786904874453541181 ) ) ;
#1652=EDGE_CURVE ( 'NONE', #18954, #20483, #19935, .T. ) ;
#1656=DIRECTION ( 'NONE',  ( 1.000000000000000000, 1.047444401652940007E-14, 0.000000000000000000 ) ) ;
#1657=AXIS2_PLACEMENT_3D ( 'NONE', #30446, #11286, #18439 ) ;
#1660=ORIENTED_EDGE ( 'NONE', *, *, #10869, .F. ) ;
#1662=DIRECTION ( 'NONE',  ( 1.000000000000000000, 1.047444401652940007E-14, 0.000000000000000000 ) ) ;
#1663=EDGE_LOOP ( 'NONE', ( #16263, #15937, #26989, #11465 ) ) ;
#1667=CARTESIAN_POINT ( 'NONE',  ( 61.16418558922029547, -0.6863720863828340901, 1.477277441814885073 ) ) ;
#1671=ORIENTED_EDGE ( 'NONE', *, *, #20492, .F. ) ;
#1681=CARTESIAN_POINT ( 'NONE',  ( 51.21569492700663062, -0.9844681138054331981, -1.555342057744142359 ) ) ;
#1682=FACE_OUTER_BOUND ( 'NONE', #29942, .T. ) ;
#1685=CIRCLE ( 'NONE', #9284, 0.09999999999999997780 ) ;
#1686=DIRECTION ( 'NONE',  ( 0.000000000000000000, 0.000000000000000000, 1.000000000000000000 ) ) ;
#1701=CARTESIAN_POINT ( 'NONE',  ( 58.75000000000004263, -1.394635017527501075, 1.253243060178017121 ) ) ;
#1718=ORIENTED_EDGE ( 'NONE', *, *, #12779, .F. ) ;
#1722=DIRECTION ( 'NONE',  ( 0.000000000000000000, 0.000000000000000000, 1.000000000000000000 ) ) ;
#1725=ADVANCED_FACE ( 'NONE', ( #25449 ), #4036, .T. ) ;
#1726=EDGE_CURVE ( 'NONE', #25442, #19414, #7799, .T. ) ;
#1737=CARTESIAN_POINT ( 'NONE',  ( 58.74999981196283017, 1.865248186430322752, 0.5877861523419425360 ) ) ;
#1751=CYLINDRICAL_SURFACE ( 'NONE', #7892, 0.5000000000000000000 ) ;
#1763=FACE_OUTER_BOUND ( 'NONE', #1200, .T. ) ;
#1765=CARTESIAN_POINT ( 'NONE',  ( 60.88446240048056524, 0.5000000000006363798, 1.718465885608440491 ) ) ;
#1767=CARTESIAN_POINT ( 'NONE',  ( 51.25000000000001421, 5.368152558471320595E-13, 3.111507638930570854E-58 ) ) ;
#1773=CARTESIAN_POINT ( 'NONE',  ( 58.75000000694009827, -1.658042653848017300, -0.9860766835992956780 ) ) ;
#1781=ORIENTED_EDGE ( 'NONE', *, *, #7380, .T. ) ;
#1786=AXIS2_PLACEMENT_3D ( 'NONE', #8044, #17551, #27356 ) ;
#1792=CARTESIAN_POINT ( 'NONE',  ( 58.75000000000003553, -1.655311165516861083, 1.077297519403202175 ) ) ;
#1794=ORIENTED_EDGE ( 'NONE', *, *, #13176, .T. ) ;
#1795=CARTESIAN_POINT ( 'NONE',  ( 52.20711756518983293, 0.5000000000005468959, -1.996089927833914146 ) ) ;
#1801=ORIENTED_EDGE ( 'NONE', *, *, #3505, .F. ) ;
#1805=( BOUNDED_CURVE ( )  B_SPLINE_CURVE ( 3, ( #14575, #3006, #7288, #19798 ),
 .UNSPECIFIED., .F., .T. ) 
 B_SPLINE_CURVE_WITH_KNOTS ( ( 4, 4 ),
 ( 1.033802687944702203, 1.276740478505648868 ),
 .UNSPECIFIED. ) 
 CURVE ( )  GEOMETRIC_REPRESENTATION_ITEM ( )  RATIONAL_B_SPLINE_CURVE ( ( 1.000000000000000000, 0.9950878134350369386, 0.9950878134350369386, 1.000000000000000000 ) ) 
 REPRESENTATION_ITEM ( '' )  );
#1806=DIRECTION ( 'NONE',  ( 0.000000000000000000, 0.000000000000000000, 1.000000000000000000 ) ) ;
#1815=CARTESIAN_POINT ( 'NONE',  ( 58.75000000000003553, -1.323060376181095732, -1.499837071478052453 ) ) ;
#1816=CARTESIAN_POINT ( 'NONE',  ( 58.66118217212468267, -0.9228675180754075669, 1.632243256842505819 ) ) ;
#1818=AXIS2_PLACEMENT_3D ( 'NONE', #29013, #4951, #3037 ) ;
#1822=CIRCLE ( 'NONE', #12942, 0.1500000000000001887 ) ;
#1826=CIRCLE ( 'NONE', #7431, 0.1499999999999999667 ) ;
#1841=EDGE_LOOP ( 'NONE', ( #628, #26422, #5505, #21184 ) ) ;
#1847=EDGE_CURVE ( 'NONE', #27521, #23889, #26879, .T. ) ;
#1849=CARTESIAN_POINT ( 'NONE',  ( 58.72200624034154259, 1.816790722508793365, -0.4641018782086855921 ) ) ;
#1858=EDGE_CURVE ( 'NONE', #19651, #21772, #2734, .T. ) ;
#1875=EDGE_CURVE ( 'NONE', #10792, #18525, #6890, .T. ) ;
#1876=CARTESIAN_POINT ( 'NONE',  ( 58.72419296898070940, 1.601054456121395964, 0.9760445624818194776 ) ) ;
#1877=CIRCLE ( 'NONE', #6952, 0.1499999999999999667 ) ;
#1881=CARTESIAN_POINT ( 'NONE',  ( 58.74999981196286569, -1.441661833134154636, 1.321459237641457563 ) ) ;
#1882=VERTEX_POINT ( 'NONE', #15903 ) ;
#1883=ORIENTED_EDGE ( 'NONE', *, *, #21252, .T. ) ;
#1884=DIRECTION ( 'NONE',  ( 0.000000000000000000, 0.000000000000000000, 1.000000000000000000 ) ) ;
#1889=CIRCLE ( 'NONE', #379, 1.875000000000001776 ) ;
#1895=DIRECTION ( 'NONE',  ( 1.000000000000000000, 1.047444401652940007E-14, 0.000000000000000000 ) ) ;
#1897=EDGE_CURVE ( 'NONE', #17885, #10721, #16797, .T. ) ;
#1900=VERTEX_POINT ( 'NONE', #31101 ) ;
#1901=AXIS2_PLACEMENT_3D ( 'NONE', #24169, #2478, #12132 ) ;
#1906=DIRECTION ( 'NONE',  ( 1.000000000000000000, 1.047444401652940007E-14, 0.000000000000000000 ) ) ;
#1908=ADVANCED_FACE ( 'NONE', ( #12113 ), #20053, .F. ) ;
#1910=CARTESIAN_POINT ( 'NONE',  ( 58.75000000000002132, 6.153735859711025284E-13, 3.111507638930570854E-58 ) ) ;
#1915=CARTESIAN_POINT ( 'NONE',  ( 51.25000000000002842, -1.099999999999462963, -1.996089927833914146 ) ) ;
#1917=VECTOR ( 'NONE', #16680, 1000.000000000000000 ) ;
#1920=DIRECTION ( 'NONE',  ( -0.000000000000000000, -0.000000000000000000, -1.000000000000000000 ) ) ;
#1922=ORIENTED_EDGE ( 'NONE', *, *, #24349, .F. ) ;
#1926=AXIS2_PLACEMENT_3D ( 'NONE', #4634, #4487, #24276 ) ;
#1931=CARTESIAN_POINT ( 'NONE',  ( 58.75000000000000000, 1.972190280208565571, -0.1053114364790996016 ) ) ;
#1932=ORIENTED_EDGE ( 'NONE', *, *, #14326, .F. ) ;
#1937=EDGE_CURVE ( 'NONE', #28767, #12009, #26394, .T. ) ;
#1939=VERTEX_POINT ( 'NONE', #14316 ) ;
#1943=CARTESIAN_POINT ( 'NONE',  ( 58.75000000000003553, -1.800471618824714071, 1.039502773796719959 ) ) ;
#1952=CARTESIAN_POINT ( 'NONE',  ( 58.65000038048068376, -1.663933463835848059, -0.8644232797864647155 ) ) ;
#1958=FACE_OUTER_BOUND ( 'NONE', #27770, .T. ) ;
#1961=CARTESIAN_POINT ( 'NONE',  ( 60.75000000000001421, 0.6500000000006350698, -1.489337100860685048 ) ) ;
#1965=DIRECTION ( 'NONE',  ( 0.000000000000000000, 0.000000000000000000, 1.000000000000000000 ) ) ;
#1967=EDGE_CURVE ( 'NONE', #31291, #24125, #14030, .T. ) ;
#1968=CARTESIAN_POINT ( 'NONE',  ( 58.65266784251147669, -1.656109637134997703, 0.8793208749736606267 ) ) ;
#1974=CARTESIAN_POINT ( 'NONE',  ( 58.65000000000004121, -1.872332544500605378, 0.09997921184723741750 ) ) ;
#1985=ADVANCED_FACE ( 'NONE', ( #25225 ), #849, .F. ) ;
#1992=CARTESIAN_POINT ( 'NONE',  ( 51.25000000000001421, 5.368159983410797313E-13, 3.111507638930570854E-58 ) ) ;
#1994=CARTESIAN_POINT ( 'NONE',  ( 58.72153194576635826, 0.5000000000006150636, -1.827449685318863093 ) ) ;
#1998=DIRECTION ( 'NONE',  ( 1.000000000000000000, 0.000000000000000000, -0.000000000000000000 ) ) ;
#2011=FACE_OUTER_BOUND ( 'NONE', #28396, .T. ) ;
#2021=CARTESIAN_POINT ( 'NONE',  ( 58.75000000000000711, 1.932246131437593162, 0.4087173687853762338 ) ) ;
#2023=CARTESIAN_POINT ( 'NONE',  ( 61.23770293222972327, 0.8897917884438596436, 1.791164585743606041 ) ) ;
#2033=CARTESIAN_POINT ( 'NONE',  ( 58.74999999305997989, -1.345908541131179081, 1.382203543031325088 ) ) ;
#2034=VERTEX_POINT ( 'NONE', #8131 ) ;
#2035=EDGE_LOOP ( 'NONE', ( #12776, #23464, #28372, #21264 ) ) ;
#2038=EDGE_CURVE ( 'NONE', #2740, #15300, #22545, .T. ) ;
#2040=DIRECTION ( 'NONE',  ( 0.000000000000000000, 0.000000000000000000, 1.000000000000000000 ) ) ;
#2045=CARTESIAN_POINT ( 'NONE',  ( 61.25000000000001421, 1.000000000000641709, 1.546164609606623053 ) ) ;
#2047=CARTESIAN_POINT ( 'NONE',  ( 58.75000000000002132, 6.153735859711025284E-13, 3.111507638930570854E-58 ) ) ;
#2062=EDGE_CURVE ( 'NONE', #20216, #21772, #20343, .T. ) ;
#2067=CARTESIAN_POINT ( 'NONE',  ( 58.75000000000004263, -1.922112613533886405, 0.4146634982040790507 ) ) ;
#2075=ORIENTED_EDGE ( 'NONE', *, *, #28271, .T. ) ;
#2077=EDGE_CURVE ( 'NONE', #507, #20216, #12900, .T. ) ;
#2078=CARTESIAN_POINT ( 'NONE',  ( 58.68279620299848176, 0.5000000000006146195, 1.809045707182517004 ) ) ;
#2081=CARTESIAN_POINT ( 'NONE',  ( 58.75000018595667939, 1.936190688449842767, -0.04992417795777597672 ) ) ;
#2085=EDGE_LOOP ( 'NONE', ( #4934, #25212, #8117, #15158, #24252, #16329 ) ) ;
#2090=CARTESIAN_POINT ( 'NONE',  ( 51.49472959044967268, -1.070956530527746420, -1.224612562803250038 ) ) ;
#2092=CARTESIAN_POINT ( 'NONE',  ( 61.00000000000002132, 6.389410850082937196E-13, 3.111507638930570854E-58 ) ) ;
#2093=AXIS2_PLACEMENT_3D ( 'NONE', #6612, #10880, #6146 ) ;
#2115=EDGE_CURVE ( 'NONE', #19132, #7871, #593, .T. ) ;
#2117=ORIENTED_EDGE ( 'NONE', *, *, #14849, .F. ) ;
#2125=ORIENTED_EDGE ( 'NONE', *, *, #2514, .T. ) ;
#2126=VERTEX_POINT ( 'NONE', #535 ) ;
#2127=( BOUNDED_SURFACE ( )  B_SPLINE_SURFACE ( 3, 2, ( 
 ( #30225, #8531, #18217 ),
 ( #6167, #25465, #2181 ),
 ( #2348, #9172, #19159 ),
 ( #16770, #12014, #4411 ),
 ( #21696, #31161, #7415 ),
 ( #21222, #28798, #31320 ),
 ( #18835, #7110, #4243 ),
 ( #9496, #14540, #11546 ),
 ( #26414, #9787, #11847 ),
 ( #19455, #28639, #14060 ) ),
 .UNSPECIFIED., .F., .F., .F. ) 
 B_SPLINE_SURFACE_WITH_KNOTS ( ( 4, 2, 2, 2, 4 ),
 ( 3, 3 ),
 ( 0.0001706658715691171911, 0.0002229276920778207674, 0.0002751895125865243437, 0.0003274513330952279200, 0.0003797131536039315505 ),
 ( 0.000000000000000000, 1.000000000000000000 ),
 .UNSPECIFIED. ) 
 GEOMETRIC_REPRESENTATION_ITEM ( )  RATIONAL_B_SPLINE_SURFACE ( (
 ( 1.000000000000000000, 0.7071067811865445751, 1.000000000000000000),
 ( 1.000000000000000000, 0.7375607040702577555, 1.000000000000000000),
 ( 1.000000000000000000, 0.7730431127429812088, 1.000000000000000000),
 ( 1.000000000000000000, 0.8321012486994131541, 1.000000000000000000),
 ( 1.000000000000000000, 0.8541932017417729339, 1.000000000000000000),
 ( 1.000000000000000000, 0.8545723906072647535, 1.000000000000000000),
 ( 1.000000000000000000, 0.8327032135058914930, 1.000000000000000000),
 ( 1.000000000000000000, 0.7734559727064781454, 1.000000000000000000),
 ( 1.000000000000000000, 0.7377766653997793744, 1.000000000000000000),
 ( 1.000000000000000000, 0.7071067811865466846, 1.000000000000000000) ) ) 
 REPRESENTATION_ITEM ( '' )  SURFACE ( )  );
#2130=CARTESIAN_POINT ( 'NONE',  ( 58.75000000000002842, -0.8948927608030053937, -1.760622601996600922 ) ) ;
#2134=DIRECTION ( 'NONE',  ( -0.000000000000000000, -0.000000000000000000, -1.000000000000000000 ) ) ;
#2138=CARTESIAN_POINT ( 'NONE',  ( 51.47729133425610115, 0.9526829978902818796, 1.321356857234310178 ) ) ;
#2139=ADVANCED_FACE ( 'NONE', ( #29657 ), #17646, .F. ) ;
#2142=ADVANCED_FACE ( 'NONE', ( #18740 ), #25522, .F. ) ;
#2150=CARTESIAN_POINT ( 'NONE',  ( 58.75000000000002842, -1.039502773796102897, -1.800471618824325493 ) ) ;
#2156=DIRECTION ( 'NONE',  ( 1.000000000000000000, 1.047444401652940007E-14, 0.000000000000000000 ) ) ;
#2164=CARTESIAN_POINT ( 'NONE',  ( 51.14630318392394770, 0.9364487020639118420, -1.503522130792751987 ) ) ;
#2170=CARTESIAN_POINT ( 'NONE',  ( 51.31572262954153985, -0.7526089581371979698, -1.996089927833914146 ) ) ;
#2177=ORIENTED_EDGE ( 'NONE', *, *, #6013, .T. ) ;
#2181=CARTESIAN_POINT ( 'NONE',  ( 58.65000038048047060, 0.8644232797865400997, -1.663933463836744231 ) ) ;
#2182=CARTESIAN_POINT ( 'NONE',  ( 58.72200624034191208, -1.341335979946730816, 1.310319377727102497 ) ) ;
#2184=EDGE_LOOP ( 'NONE', ( #27777, #22817, #4422, #9131, #26467 ) ) ;
#2188=CARTESIAN_POINT ( 'NONE',  ( 58.65815574817776223, -0.5272471384221183444, 1.799565140951959963 ) ) ;
#2189=CARTESIAN_POINT ( 'NONE',  ( 58.65000000000000568, 0.8495817349399593654, 1.671477153794648896 ) ) ;
#2204=CARTESIAN_POINT ( 'NONE',  ( 58.75000000000000000, 2.079005547593415937, 1.004182178118534636E-12 ) ) ;
#2210=DIRECTION ( 'NONE',  ( 1.000000000000000000, 1.047444401652940007E-14, 0.000000000000000000 ) ) ;
#2212=EDGE_CURVE ( 'NONE', #29156, #28572, #6857, .T. ) ;
#2214=DIRECTION ( 'NONE',  ( -0.000000000000000000, -0.000000000000000000, -1.000000000000000000 ) ) ;
#2218=CARTESIAN_POINT ( 'NONE',  ( 51.25000000000002842, -1.099999999999462963, 1.196087371390569087 ) ) ;
#2223=ORIENTED_EDGE ( 'NONE', *, *, #30510, .T. ) ;
#2224=CARTESIAN_POINT ( 'NONE',  ( 51.35647303904148231, -1.001029238032807633, -1.398203054920482025 ) ) ;
#2225=EDGE_CURVE ( 'NONE', #29589, #67, #17282, .T. ) ;
#2228=CARTESIAN_POINT ( 'NONE',  ( 58.67159525762672700, 0.5000000000007230883, 1.807104036850089468 ) ) ;
#2230=LINE ( 'NONE', #11895, #29634 ) ;
#2231=EDGE_LOOP ( 'NONE', ( #12494, #26433, #20885, #23045, #6777, #24843 ) ) ;
#2236=ORIENTED_EDGE ( 'NONE', *, *, #11052, .T. ) ;
#2249=CIRCLE ( 'NONE', #12863, 1.625000000000000222 ) ;
#2254=DIRECTION ( 'NONE',  ( 1.000000000000000000, 1.047444401652940007E-14, 0.000000000000000000 ) ) ;
#2264=CARTESIAN_POINT ( 'NONE',  ( 58.65000000000001279, 0.6121634413844184719, -1.877732920580865272 ) ) ;
#2274=ORIENTED_EDGE ( 'NONE', *, *, #29608, .F. ) ;
#2276=( BOUNDED_SURFACE ( )  B_SPLINE_SURFACE ( 3, 2, ( 
 ( #1792, #16224, #18611 ),
 ( #30610, #11469, #13519 ),
 ( #6712, #30307, #21312 ),
 ( #18920, #16374, #8617 ),
 ( #18293, #13983, #13347 ),
 ( #8757, #23040, #4026 ),
 ( #8924, #16067, #28409 ),
 ( #25719, #28561, #1968 ),
 ( #27933, #11633, #21152 ),
 ( #28254, #30941, #6564 ) ),
 .UNSPECIFIED., .F., .F., .F. ) 
 B_SPLINE_SURFACE_WITH_KNOTS ( ( 4, 2, 2, 2, 4 ),
 ( 3, 3 ),
 ( 0.0001706658715701343896, 0.0002229276920781098699, 0.0002751895125860853502, 0.0003274513330940608848, 0.0003797131536020363651 ),
 ( 0.000000000000000000, 1.000000000000000000 ),
 .UNSPECIFIED. ) 
 GEOMETRIC_REPRESENTATION_ITEM ( )  RATIONAL_B_SPLINE_SURFACE ( (
 ( 1.000000000000000000, 0.7071067811873458231, 1.000000000000000000),
 ( 1.000000000000000000, 0.7375607040708066497, 1.000000000000000000),
 ( 1.000000000000000000, 0.7730431127427257465, 1.000000000000000000),
 ( 1.000000000000000000, 0.8321012486970551514, 1.000000000000000000),
 ( 1.000000000000000000, 0.8541932017381971276, 1.000000000000000000),
 ( 1.000000000000000000, 0.8545723906028362959, 1.000000000000000000),
 ( 1.000000000000000000, 0.8327032135022484072, 1.000000000000000000),
 ( 1.000000000000000000, 0.7734559727053097467, 1.000000000000000000),
 ( 1.000000000000000000, 0.7377766653992025025, 1.000000000000000000),
 ( 1.000000000000000000, 0.7071067811865759944, 1.000000000000000000) ) ) 
 REPRESENTATION_ITEM ( '' )  SURFACE ( )  );
#2277=CARTESIAN_POINT ( 'NONE',  ( 51.23644008536124517, -1.080112125195908046, 1.214076932077873039 ) ) ;
#2279=AXIS2_PLACEMENT_3D ( 'NONE', #9892, #19568, #29213 ) ;
#2285=CIRCLE ( 'NONE', #15922, 0.1000000000000001027 ) ;
#2289=PLANE ( 'NONE',  #13484 ) ;
#2293=EDGE_CURVE ( 'NONE', #23458, #29895, #18212, .T. ) ;
#2295=CARTESIAN_POINT ( 'NONE',  ( 51.02976068049071756, 1.019450805965458340, 1.268081568884036114 ) ) ;
#2297=DIRECTION ( 'NONE',  ( 1.000000000000000000, 1.047444401652940007E-14, 0.000000000000000000 ) ) ;
#2299=CIRCLE ( 'NONE', #12395, 0.1500000000000001887 ) ;
#2308=ORIENTED_EDGE ( 'NONE', *, *, #28100, .T. ) ;
#2311=ORIENTED_EDGE ( 'NONE', *, *, #21252, .F. ) ;
#2312=AXIS2_PLACEMENT_3D ( 'NONE', #26682, #22092, #22247 ) ;
#2316=CARTESIAN_POINT ( 'NONE',  ( 58.65000000000004121, -1.590093208332549413, 0.9941784314378853127 ) ) ;
#2342=CARTESIAN_POINT ( 'NONE',  ( 51.25000000000001421, 5.368152558471320595E-13, 3.111507638930570854E-58 ) ) ;
#2344=CIRCLE ( 'NONE', #20057, 1.487500000000000933 ) ;
#2348=CARTESIAN_POINT ( 'NONE',  ( 58.74999981404332772, 0.9032433253516619631, -1.734728236459875728 ) ) ;
#2349=CARTESIAN_POINT ( 'NONE',  ( 58.75000000000002132, 6.153735859711025284E-13, 3.111507638930570854E-58 ) ) ;
#2352=DIRECTION ( 'NONE',  ( 0.000000000000000000, 0.000000000000000000, 1.000000000000000000 ) ) ;
#2355=CARTESIAN_POINT ( 'NONE',  ( 58.75000000000004263, -2.079005547593188119, 1.932245437381540134E-15 ) ) ;
#2359=CARTESIAN_POINT ( 'NONE',  ( 61.25000000000001421, 1.000000000000641709, 1.655766640118845112 ) ) ;
#2364=EDGE_CURVE ( 'NONE', #28412, #17938, #22756, .T. ) ;
#2365=CIRCLE ( 'NONE', #17529, 1.875000000000001776 ) ;
#2366=CARTESIAN_POINT ( 'NONE',  ( 58.64999999999999858, 1.655311165516931471, 1.077297519405395310 ) ) ;
#2370=EDGE_LOOP ( 'NONE', ( #6560, #30304, #10944, #27026 ) ) ;
#2371=DIRECTION ( 'NONE',  ( 0.000000000000000000, 0.000000000000000000, 1.000000000000000000 ) ) ;
#2379=EDGE_CURVE ( 'NONE', #27051, #15300, #11016, .T. ) ;
#2380=VECTOR ( 'NONE', #19019, 1000.000000000000000 ) ;
#2383=CARTESIAN_POINT ( 'NONE',  ( 61.24672990992804245, -0.9412912739128637130, 1.685898893893857053 ) ) ;
#2387=VERTEX_POINT ( 'NONE', #4770 ) ;
#2389=VECTOR ( 'NONE', #3649, 1000.000000000000000 ) ;
#2391=CARTESIAN_POINT ( 'NONE',  ( 51.45655683570191741, -0.9591657938390835136, -1.468576096419531574 ) ) ;
#2393=CARTESIAN_POINT ( 'NONE',  ( 52.20711756518982583, 0.7500000000005468959, 1.718465885608440269 ) ) ;
#2397=ORIENTED_EDGE ( 'NONE', *, *, #22347, .T. ) ;
#2401=ORIENTED_EDGE ( 'NONE', *, *, #21227, .T. ) ;
#2407=AXIS2_PLACEMENT_3D ( 'NONE', #17777, #15847, #13010 ) ;
#2410=CIRCLE ( 'NONE', #20121, 1.875000000000001776 ) ;
#2412=VECTOR ( 'NONE', #11803, 1000.000000000000000 ) ;
#2417=DIRECTION ( 'NONE',  ( 1.000000000000000000, 1.047444401652940007E-14, 0.000000000000000000 ) ) ;
#2419=CARTESIAN_POINT ( 'NONE',  ( 58.65000000000000568, 1.077297519403822568, 1.655311165517741490 ) ) ;
#2426=CARTESIAN_POINT ( 'NONE',  ( 61.25000000000004263, -1.895722432251839562, -0.6373668173467583742 ) ) ;
#2436=DIRECTION ( 'NONE',  ( 0.000000000000000000, 0.000000000000000000, 1.000000000000000000 ) ) ;
#2437=ORIENTED_EDGE ( 'NONE', *, *, #25376, .F. ) ;
#2444=CARTESIAN_POINT ( 'NONE',  ( 58.65000000000003411, -1.394635017527501297, 1.253243060178016455 ) ) ;
#2447=ORIENTED_EDGE ( 'NONE', *, *, #29611, .F. ) ;
#2450=CARTESIAN_POINT ( 'NONE',  ( 51.59739104186229497, -1.010292945602101256, 1.272765950230260623 ) ) ;
#2453=ORIENTED_EDGE ( 'NONE', *, *, #23414, .T. ) ;
#2454=AXIS2_PLACEMENT_3D ( 'NONE', #10410, #19925, #8195 ) ;
#2455=CARTESIAN_POINT ( 'NONE',  ( 52.15659655364832048, -0.4999999999994547695, -1.807104036850121886 ) ) ;
#2456=CARTESIAN_POINT ( 'NONE',  ( 52.06628335902946247, -0.5434431642975677823, 1.718465885608439603 ) ) ;
#2458=DIRECTION ( 'NONE',  ( 0.000000000000000000, 0.000000000000000000, 1.000000000000000000 ) ) ;
#2462=CARTESIAN_POINT ( 'NONE',  ( 58.73379417893118415, -0.8670685180651961366, 1.662624490945991740 ) ) ;
#2466=DIRECTION ( 'NONE',  ( 0.000000000000000000, 0.000000000000000000, 1.000000000000000000 ) ) ;
#2471=ORIENTED_EDGE ( 'NONE', *, *, #9703, .T. ) ;
#2474=EDGE_LOOP ( 'NONE', ( #6328, #2570, #20144, #14080, #18366, #17961 ) ) ;
#2475=( BOUNDED_SURFACE ( )  B_SPLINE_SURFACE ( 3, 2, ( 
 ( #15199, #19807, #14145 ),
 ( #29440, #26341, #11626 ),
 ( #29592, #7752, #10289 ),
 ( #24536, #4644, #17418 ) ),
 .UNSPECIFIED., .F., .F., .F. ) 
 B_SPLINE_SURFACE_WITH_KNOTS ( ( 4, 4 ),
 ( 3, 3 ),
 ( 4.041453792691653391, 4.300872134317200945 ),
 ( 0.000000000000000000, 1.000000000000000000 ),
 .UNSPECIFIED. ) 
 GEOMETRIC_REPRESENTATION_ITEM ( )  RATIONAL_B_SPLINE_SURFACE ( (
 ( 1.000000000000000000, 0.8699658093904929501, 1.000000000000000000),
 ( 1.000000000000000000, 0.8538860448759273414, 1.000000000000000000),
 ( 1.000000000000000000, 0.8356979842195431107, 1.000000000000000000),
 ( 1.000000000000000000, 0.8156258140602941076, 1.000000000000000000) ) ) 
 REPRESENTATION_ITEM ( '' )  SURFACE ( )  );
#2476=CARTESIAN_POINT ( 'NONE',  ( 61.25000000000003553, -1.106298139389941149, 1.666164585742037296 ) ) ;
#2478=DIRECTION ( 'NONE',  ( 1.000000000000000000, 1.047444401652940007E-14, -0.000000000000000000 ) ) ;
#2483=ORIENTED_EDGE ( 'NONE', *, *, #13665, .F. ) ;
#2502=ORIENTED_EDGE ( 'NONE', *, *, #8643, .T. ) ;
#2503=ADVANCED_FACE ( 'NONE', ( #20149 ), #19971, .F. ) ;
#2508=EDGE_CURVE ( 'NONE', #21159, #28946, #14385, .T. ) ;
#2513=ORIENTED_EDGE ( 'NONE', *, *, #29211, .F. ) ;
#2514=EDGE_CURVE ( 'NONE', #1336, #2034, #12622, .T. ) ;
#2526=VERTEX_POINT ( 'NONE', #13752 ) ;
#2528=CARTESIAN_POINT ( 'NONE',  ( 61.24012582333622845, 0.9011229182324727027, 1.742583661752045820 ) ) ;
#2529=LINE ( 'NONE', #2045, #8954 ) ;
#2532=B_SPLINE_CURVE_WITH_KNOTS ( 'NONE', 3,
 ( #14574, #19486, #19194, #16656, #24238, #17121 ),
 .UNSPECIFIED., .F., .F.,
 ( 4, 2, 4 ),
 ( 0.000000000000000000, 0.0001000270069610660921, 0.0002000540139221321841 ),
 .UNSPECIFIED. ) ;
#2533=DIRECTION ( 'NONE',  ( -7.145967004358956819E-15, 0.5454670984331110306, -0.8381322357044637128 ) ) ;
#2544=EDGE_CURVE ( 'NONE', #19199, #2126, #16698, .T. ) ;
#2551=CARTESIAN_POINT ( 'NONE',  ( 58.65000000000004121, -1.782657835994441387, 0.5811678240968194409 ) ) ;
#2557=ORIENTED_EDGE ( 'NONE', *, *, #18563, .T. ) ;
#2559=ORIENTED_EDGE ( 'NONE', *, *, #30590, .F. ) ;
#2570=ORIENTED_EDGE ( 'NONE', *, *, #9386, .T. ) ;
#2571=ORIENTED_EDGE ( 'NONE', *, *, #23479, .F. ) ;
#2574=CARTESIAN_POINT ( 'NONE',  ( 58.75000000000003553, -1.800471618824714071, 1.039502773796719959 ) ) ;
#2578=CARTESIAN_POINT ( 'NONE',  ( 50.55258015808398397, 5.293720379222080095E-13, -1.177580158083963546 ) ) ;
#2583=CARTESIAN_POINT ( 'NONE',  ( 61.25000000000001421, 1.106298139389969348, 1.666164585743605375 ) ) ;
#2585=ORIENTED_EDGE ( 'NONE', *, *, #9944, .T. ) ;
#2586=CARTESIAN_POINT ( 'NONE',  ( 58.65000000000003411, -1.394635017527761311, -1.253243060177727131 ) ) ;
#2593=CARTESIAN_POINT ( 'NONE',  ( 51.41639946534622396, 0.9865458190826668083, 1.594793944595433111 ) ) ;
#2603=VERTEX_POINT ( 'NONE', #20614 ) ;
#2604=CARTESIAN_POINT ( 'NONE',  ( 61.21683709729278888, -0.7974544867251196489, -1.837034727152028424 ) ) ;
#2605=CARTESIAN_POINT ( 'NONE',  ( 50.25000000000004263, -1.800471618824301734, -1.039502773796582069 ) ) ;
#2608=CIRCLE ( 'NONE', #6060, 0.1499999999999999667 ) ;
#2616=CARTESIAN_POINT ( 'NONE',  ( 51.36283714269074352, 1.001673184508090397, 1.284520656909115877 ) ) ;
#2618=EDGE_CURVE ( 'NONE', #24348, #28516, #29867, .T. ) ;
#2622=ORIENTED_EDGE ( 'NONE', *, *, #20452, .F. ) ;
#2638=CARTESIAN_POINT ( 'NONE',  ( 51.13996726386385916, -0.9386186536664237190, 1.439073407537155180 ) ) ;
#2639=DIRECTION ( 'NONE',  ( 1.000000000000000000, 1.047444401652940007E-14, 0.000000000000000000 ) ) ;
#2643=EDGE_CURVE ( 'NONE', #19132, #30566, #10273, .T. ) ;
#2649=ADVANCED_FACE ( 'NONE', ( #10922 ), #8550, .F. ) ;
#2656=DIRECTION ( 'NONE',  ( 1.000000000000000000, 1.047444401652940007E-14, 0.000000000000000000 ) ) ;
#2657=CARTESIAN_POINT ( 'NONE',  ( 51.55144386500332132, -1.037443573994098811, -1.251214392908860829 ) ) ;
#2686=DIRECTION ( 'NONE',  ( -0.000000000000000000, -0.000000000000000000, -1.000000000000000000 ) ) ;
#2693=CARTESIAN_POINT ( 'NONE',  ( 58.73379417893125520, -1.788763080991752963, 0.5625430232375976392 ) ) ;
#2697=DIRECTION ( 'NONE',  ( -1.000000000000000000, -1.047444401652940007E-14, -0.000000000000000000 ) ) ;
#2707=ORIENTED_EDGE ( 'NONE', *, *, #15872, .F. ) ;
#2725=CARTESIAN_POINT ( 'NONE',  ( 52.13000000000003098, -0.4999999999994542144, -1.718465885608440269 ) ) ;
#2730=DIRECTION ( 'NONE',  ( 0.000000000000000000, 0.000000000000000000, 1.000000000000000000 ) ) ;
#2731=CARTESIAN_POINT ( 'NONE',  ( 58.75000000000000711, 1.877732920581273390, 0.6121634413844396772 ) ) ;
#2734=B_SPLINE_CURVE_WITH_KNOTS ( 'NONE', 3,
 ( #23364, #11303, #16555, #25884, #23509, #25562 ),
 .UNSPECIFIED., .F., .F.,
 ( 4, 2, 4 ),
 ( 0.000000000000000000, 0.0003974125641964907241, 0.0007948251283929814483 ),
 .UNSPECIFIED. ) ;
#2739=ORIENTED_EDGE ( 'NONE', *, *, #19326, .F. ) ;
#2740=VERTEX_POINT ( 'NONE', #17519 ) ;
#2741=CARTESIAN_POINT ( 'NONE',  ( 58.66054497608038076, -0.4999999999994944599, -1.807104036850091688 ) ) ;
#2742=ORIENTED_EDGE ( 'NONE', *, *, #13315, .T. ) ;
#2751=ORIENTED_EDGE ( 'NONE', *, *, #7123, .T. ) ;
#2754=CARTESIAN_POINT ( 'NONE',  ( 58.74999981196286569, -0.9033020670124441986, -1.734557215428337296 ) ) ;
#2758=CIRCLE ( 'NONE', #20475, 1.875000000000001776 ) ;
#2768=DIRECTION ( 'NONE',  ( 0.000000000000000000, 0.000000000000000000, 1.000000000000000000 ) ) ;
#2769=DIRECTION ( 'NONE',  ( 1.000000000000000000, 1.047444401652940007E-14, 0.000000000000000000 ) ) ;
#2775=ORIENTED_EDGE ( 'NONE', *, *, #3509, .F. ) ;
#2777=ORIENTED_EDGE ( 'NONE', *, *, #2818, .F. ) ;
#2782=EDGE_CURVE ( 'NONE', #22168, #5779, #5526, .T. ) ;
#2784=AXIS2_PLACEMENT_3D ( 'NONE', #23788, #21417, #631 ) ;
#2787=LINE ( 'NONE', #423, #11966 ) ;
#2793=VERTEX_POINT ( 'NONE', #21245 ) ;
#2800=ORIENTED_EDGE ( 'NONE', *, *, #26083, .T. ) ;
#2804=CARTESIAN_POINT ( 'NONE',  ( 58.65000000000000568, 0.8794134543724719810, 1.656314228059073912 ) ) ;
#2809=CARTESIAN_POINT ( 'NONE',  ( 58.75000000000000000, 1.972190280208565571, -0.1053114364790996849 ) ) ;
#2818=EDGE_CURVE ( 'NONE', #14302, #28844, #1468, .T. ) ;
#2819=CARTESIAN_POINT ( 'NONE',  ( 50.25000000000004263, -1.996089927834391764, 0.1250000000000018041 ) ) ;
#2823=EDGE_CURVE ( 'NONE', #30150, #12308, #9108, .T. ) ;
#2824=VERTEX_POINT ( 'NONE', #30166 ) ;
#2825=AXIS2_PLACEMENT_3D ( 'NONE', #21286, #4301, #7017 ) ;
#2826=CIRCLE ( 'NONE', #7384, 0.1500000000000001887 ) ;
#2832=FACE_OUTER_BOUND ( 'NONE', #17196, .T. ) ;
#2833=CIRCLE ( 'NONE', #3341, 2.000000000000000000 ) ;
#2839=CIRCLE ( 'NONE', #20569, 0.1500000000000001887 ) ;
#2840=ORIENTED_EDGE ( 'NONE', *, *, #7061, .T. ) ;
#2842=CARTESIAN_POINT ( 'NONE',  ( 61.00000000000001421, 1.000000000000639044, 1.586072192556190252 ) ) ;
#2849=ORIENTED_EDGE ( 'NONE', *, *, #10793, .T. ) ;
#2851=AXIS2_PLACEMENT_3D ( 'NONE', #29246, #7559, #17219 ) ;
#2857=CARTESIAN_POINT ( 'NONE',  ( 60.75000000000001421, 0.7500000000006363798, -1.718465885608440047 ) ) ;
#2863=AXIS2_PLACEMENT_3D ( 'NONE', #26528, #4836, #7540 ) ;
#2875=CYLINDRICAL_SURFACE ( 'NONE', #30172, 2.000000000000000000 ) ;
#2877=CARTESIAN_POINT ( 'NONE',  ( 50.55258015808398397, -0.05176326469654482509, -1.177580158083963324 ) ) ;
#2880=DIRECTION ( 'NONE',  ( 1.000000000000000000, 1.047444401652940007E-14, 0.000000000000000000 ) ) ;
#2892=AXIS2_PLACEMENT_3D ( 'NONE', #5034, #24660, #17090 ) ;
#2894=CONICAL_SURFACE ( 'NONE', #25675, 1.487500000000000933, 0.7853981633974481680 ) ;
#2899=ORIENTED_EDGE ( 'NONE', *, *, #16827, .F. ) ;
#2910=B_SPLINE_CURVE_WITH_KNOTS ( 'NONE', 3,
 ( #24331, #2638, #20054, #12280, #14809, #17211 ),
 .UNSPECIFIED., .F., .F.,
 ( 4, 2, 4 ),
 ( 0.000000000000000000, 0.0001701207528151775234, 0.0003402415056303550469 ),
 .UNSPECIFIED. ) ;
#2915=FACE_OUTER_BOUND ( 'NONE', #2370, .T. ) ;
#2920=CIRCLE ( 'NONE', #28712, 1.975000000000001865 ) ;
#2923=DIRECTION ( 'NONE',  ( 1.000000000000000000, 1.047444401652940007E-14, 0.000000000000000000 ) ) ;
#2924=CARTESIAN_POINT ( 'NONE',  ( 58.66595318830262329, -0.4999999999993857136, 1.807217177072697245 ) ) ;
#2931=VERTEX_POINT ( 'NONE', #1349 ) ;
#2933=EDGE_CURVE ( 'NONE', #22181, #14808, #797, .T. ) ;
#2934=DIRECTION ( 'NONE',  ( 1.000000000000000000, 1.047444401652940007E-14, 0.000000000000000000 ) ) ;
#2942=ORIENTED_EDGE ( 'NONE', *, *, #3426, .F. ) ;
#2954=DIRECTION ( 'NONE',  ( 0.000000000000000000, 0.000000000000000000, 1.000000000000000000 ) ) ;
#2955=DIRECTION ( 'NONE',  ( 5.167928589571388008E-15, -0.4531102586341528293, -0.8914544820238951006 ) ) ;
#2961=CARTESIAN_POINT ( 'NONE',  ( 51.19148447764912646, -0.9872860527319672341, 1.295557643792433433 ) ) ;
#2962=ORIENTED_EDGE ( 'NONE', *, *, #25304, .T. ) ;
#2964=CARTESIAN_POINT ( 'NONE',  ( 51.59739104186229497, -1.010292945602101256, -1.272765950230260623 ) ) ;
#2971=DIRECTION ( 'NONE',  ( 1.000000000000000000, 1.047444401652940007E-14, 0.000000000000000000 ) ) ;
#2977=B_SPLINE_CURVE_WITH_KNOTS ( 'NONE', 3,
 ( #12007, #7245, #4867, #12160, #21842, #19447 ),
 .UNSPECIFIED., .F., .F.,
 ( 4, 2, 4 ),
 ( 0.000000000000000000, 0.0001000270069610858788, 0.0002000540139221717575 ),
 .UNSPECIFIED. ) ;
#2978=CARTESIAN_POINT ( 'NONE',  ( 60.88861521483879358, -0.6775725165974680886, -1.477731239195208879 ) ) ;
#2989=DIRECTION ( 'NONE',  ( 0.000000000000000000, 0.000000000000000000, 1.000000000000000000 ) ) ;
#2996=CARTESIAN_POINT ( 'NONE',  ( 52.20711756518982583, 0.7500000000005468959, -1.718465885608440269 ) ) ;
#2999=CARTESIAN_POINT ( 'NONE',  ( 61.25000000000003553, -0.9840188032644283656, 1.660129320693359167 ) ) ;
#3003=EDGE_CURVE ( 'NONE', #833, #28572, #20711, .T. ) ;
#3006=CARTESIAN_POINT ( 'NONE',  ( 51.64837794009021366, -0.8283786772106966900, -1.688958810662479104 ) ) ;
#3019=EDGE_CURVE ( 'NONE', #20216, #10008, #6581, .T. ) ;
#3023=AXIS2_PLACEMENT_3D ( 'NONE', #1575, #1906, #30541 ) ;
#3030=AXIS2_PLACEMENT_3D ( 'NONE', #29194, #4499, #7509 ) ;
#3034=CARTESIAN_POINT ( 'NONE',  ( 51.17957687186119387, 0.9671124184268959922, -1.523623459118158552 ) ) ;
#3037=DIRECTION ( 'NONE',  ( 0.000000000000000000, 0.000000000000000000, 1.000000000000000000 ) ) ;
#3048=VERTEX_POINT ( 'NONE', #28268 ) ;
#3053=ORIENTED_EDGE ( 'NONE', *, *, #30454, .F. ) ;
#3070=CARTESIAN_POINT ( 'NONE',  ( 51.16540481435728793, 0.9540520100826064276, 1.477289350867987405 ) ) ;
#3073=FACE_OUTER_BOUND ( 'NONE', #29067, .T. ) ;
#3075=CARTESIAN_POINT ( 'NONE',  ( 51.34441612831281532, 1.002608958138276440, 1.395204572094387085 ) ) ;
#3077=CARTESIAN_POINT ( 'NONE',  ( 58.72419296898062413, 1.357170036000971081, -1.293880926823457456 ) ) ;
#3080=CARTESIAN_POINT ( 'NONE',  ( 51.45655683570191741, -0.9591657938390835136, 1.468576096419531574 ) ) ;
#3088=ORIENTED_EDGE ( 'NONE', *, *, #25651, .T. ) ;
#3090=ORIENTED_EDGE ( 'NONE', *, *, #19574, .T. ) ;
#3091=CARTESIAN_POINT ( 'NONE',  ( 51.44193764627932808, 0.9752197701250188144, -1.304631266258923006 ) ) ;
#3105=FACE_OUTER_BOUND ( 'NONE', #9254, .T. ) ;
#3112=B_SPLINE_CURVE_WITH_KNOTS ( 'NONE', 3,
 ( #19978, #15222, #3034, #22054 ),
 .UNSPECIFIED., .F., .F.,
 ( 4, 4 ),
 ( 2.168404344971008868E-19, 0.0001476506082772737762 ),
 .UNSPECIFIED. ) ;
#3122=CARTESIAN_POINT ( 'NONE',  ( 51.25000000000001421, 5.368152558471320595E-13, 3.111507638930570854E-58 ) ) ;
#3124=CARTESIAN_POINT ( 'NONE',  ( 58.65000000000000568, 1.394635017528131904, 1.253243060178682144 ) ) ;
#3126=ORIENTED_EDGE ( 'NONE', *, *, #29024, .F. ) ;
#3143=DIRECTION ( 'NONE',  ( 1.000000000000000000, 0.000000000000000000, -0.000000000000000000 ) ) ;
#3153=EDGE_CURVE ( 'NONE', #28946, #22153, #13621, .T. ) ;
#3154=PLANE ( 'NONE',  #15838 ) ;
#3155=ORIENTED_EDGE ( 'NONE', *, *, #26129, .T. ) ;
#3157=FACE_OUTER_BOUND ( 'NONE', #26227, .T. ) ;
#3158=DIRECTION ( 'NONE',  ( 0.000000000000000000, 0.000000000000000000, 1.000000000000000000 ) ) ;
#3159=CARTESIAN_POINT ( 'NONE',  ( 58.75000000000002132, -0.4999999999991823207, -1.863080903343696137 ) ) ;
#3164=ORIENTED_EDGE ( 'NONE', *, *, #4179, .F. ) ;
#3174=EDGE_CURVE ( 'NONE', #16870, #31166, #2344, .T. ) ;
#3183=CYLINDRICAL_SURFACE ( 'NONE', #23527, 0.1500000000000001887 ) ;
#3184=VECTOR ( 'NONE', #14103, 1000.000000000000000 ) ;
#3187=DIRECTION ( 'NONE',  ( -1.000000000000000000, -1.047444401652940007E-14, -0.000000000000000000 ) ) ;
#3193=DIRECTION ( 'NONE',  ( 1.000000000000000000, 1.047444401652940007E-14, 0.000000000000000000 ) ) ;
#3202=ORIENTED_EDGE ( 'NONE', *, *, #25541, .T. ) ;
#3205=( NAMED_UNIT ( * ) PLANE_ANGLE_UNIT ( ) SI_UNIT ( $, .RADIAN. ) );
#3216=EDGE_CURVE ( 'NONE', #23636, #23889, #18934, .T. ) ;
#3219=EDGE_CURVE ( 'NONE', #6099, #11926, #15951, .T. ) ;
#3220=CARTESIAN_POINT ( 'NONE',  ( 58.75000000000001421, 0.6121634413844194711, -1.877732920580865050 ) ) ;
#3225=DIRECTION ( 'NONE',  ( 0.000000000000000000, 0.000000000000000000, 1.000000000000000000 ) ) ;
#3233=ORIENTED_EDGE ( 'NONE', *, *, #28271, .F. ) ;
#3247=CARTESIAN_POINT ( 'NONE',  ( 51.38214458811555829, 1.084857585946179315, -1.209959298770756808 ) ) ;
#3251=CARTESIAN_POINT ( 'NONE',  ( 50.75360625943719839, 0.3719558471750604722, -1.344678919698701014 ) ) ;
#3252=CARTESIAN_POINT ( 'NONE',  ( 51.31572262954153985, -0.7526089581371979698, -1.996089927833914146 ) ) ;
#3253=VECTOR ( 'NONE', #9511, 1000.000000000000000 ) ;
#3258=FACE_OUTER_BOUND ( 'NONE', #23705, .T. ) ;
#3260=CARTESIAN_POINT ( 'NONE',  ( 58.64999999999999147, 1.793030239489902478, 0.5493518053835514392 ) ) ;
#3262=CARTESIAN_POINT ( 'NONE',  ( 58.75000000000000711, 0.8948927608033926395, 1.760622601997029912 ) ) ;
#3263=DIRECTION ( 'NONE',  ( 0.000000000000000000, 0.000000000000000000, 1.000000000000000000 ) ) ;
#3283=CARTESIAN_POINT ( 'NONE',  ( 60.75000000000002132, -0.4999999999993638977, -1.718465885608440047 ) ) ;
#3284=ADVANCED_FACE ( 'NONE', ( #9371 ), #19229, .F. ) ;
#3285=DIRECTION ( 'NONE',  ( 0.000000000000000000, 0.000000000000000000, 1.000000000000000000 ) ) ;
#3286=ORIENTED_EDGE ( 'NONE', *, *, #1652, .T. ) ;
#3290=ADVANCED_FACE ( 'NONE', ( #7008 ), #1751, .T. ) ;
#3293=CARTESIAN_POINT ( 'NONE',  ( 50.59602332238209499, -0.1408342061598474859, 1.212874140286674285 ) ) ;
#3314=CARTESIAN_POINT ( 'NONE',  ( 58.74160516400043264, -1.258299259018153204, 1.390091577293904423 ) ) ;
#3320=EDGE_CURVE ( 'NONE', #1882, #9827, #2230, .T. ) ;
#3321=CIRCLE ( 'NONE', #4304, 0.1499999999999999667 ) ;
#3325=CARTESIAN_POINT ( 'NONE',  ( 51.25000000000001421, 1.100000000000537215, -1.196087371390568643 ) ) ;
#3326=CARTESIAN_POINT ( 'NONE',  ( 52.20711756518982583, 0.7500000000005468959, -1.996089927833914146 ) ) ;
#3341=AXIS2_PLACEMENT_3D ( 'NONE', #22217, #9855, #5248 ) ;
#3342=CIRCLE ( 'NONE', #15485, 0.1500000000000001887 ) ;
#3346=CARTESIAN_POINT ( 'NONE',  ( 58.66118217212486741, -1.815481606354510724, -0.4689659288411509031 ) ) ;
#3348=CARTESIAN_POINT ( 'NONE',  ( 58.75000000000002132, 6.153735859711025284E-13, 3.111507638930570854E-58 ) ) ;
#3351=CARTESIAN_POINT ( 'NONE',  ( 50.50000000000002132, 5.291762632692320630E-13, 3.111507638930570854E-58 ) ) ;
#3353=EDGE_LOOP ( 'NONE', ( #29832, #4972, #15380, #12265 ) ) ;
#3355=AXIS2_PLACEMENT_3D ( 'NONE', #15910, #20841, #25418 ) ;
#3359=ORIENTED_EDGE ( 'NONE', *, *, #29768, .T. ) ;
#3362=EDGE_CURVE ( 'NONE', #11262, #1256, #1313, .T. ) ;
#3379=AXIS2_PLACEMENT_3D ( 'NONE', #21214, #25929, #6046 ) ;
#3381=ORIENTED_EDGE ( 'NONE', *, *, #30108, .T. ) ;
#3385=CIRCLE ( 'NONE', #26136, 0.2500000000000000000 ) ;
#3386=CARTESIAN_POINT ( 'NONE',  ( 58.66122331388464772, 0.5173534011644945751, -1.802520131073004128 ) ) ;
#3392=AXIS2_PLACEMENT_3D ( 'NONE', #1487, #24248, #4922 ) ;
#3394=AXIS2_PLACEMENT_3D ( 'NONE', #26527, #30818, #28442 ) ;
#3398=CARTESIAN_POINT ( 'NONE',  ( 58.64999999999999858, 1.394635017529600951, -1.253243060177047452 ) ) ;
#3401=ORIENTED_EDGE ( 'NONE', *, *, #5205, .T. ) ;
#3403=DIRECTION ( 'NONE',  ( 0.000000000000000000, -0.8381322357052107819, 0.5454670984319629490 ) ) ;
#3409=VECTOR ( 'NONE', #11236, 1000.000000000000000 ) ;
#3426=EDGE_CURVE ( 'NONE', #17938, #27064, #28745, .T. ) ;
#3439=EDGE_LOOP ( 'NONE', ( #9222, #4212, #12728, #14863 ) ) ;
#3445=EDGE_CURVE ( 'NONE', #29950, #14808, #22443, .T. ) ;
#3455=EDGE_CURVE ( 'NONE', #12058, #12009, #19040, .T. ) ;
#3456=ORIENTED_EDGE ( 'NONE', *, *, #21208, .T. ) ;
#3464=CARTESIAN_POINT ( 'NONE',  ( 58.75000000000000711, 1.652371589363942794, -1.066009655021259883 ) ) ;
#3466=CARTESIAN_POINT ( 'NONE',  ( 51.78364358464227024, -0.9002346248696042608, 1.360127766454835685 ) ) ;
#3468=ORIENTED_EDGE ( 'NONE', *, *, #15966, .T. ) ;
#3475=CARTESIAN_POINT ( 'NONE',  ( 58.72204580543430552, -1.874996463825583826, 0.02257357450724356909 ) ) ;
#3482=CARTESIAN_POINT ( 'NONE',  ( 61.25000000000002132, 6.415596960124259844E-13, 3.111507638930570854E-58 ) ) ;
#3486=DIRECTION ( 'NONE',  ( 0.000000000000000000, 0.000000000000000000, 1.000000000000000000 ) ) ;
#3487=( GEOMETRIC_REPRESENTATION_CONTEXT ( 3 ) GLOBAL_UNCERTAINTY_ASSIGNED_CONTEXT ( ( #19948 ) ) GLOBAL_UNIT_ASSIGNED_CONTEXT ( ( #5741, #3205, #13168 ) ) REPRESENTATION_CONTEXT ( 'NONE', 'WORKASPACE' ) );
#3492=CARTESIAN_POINT ( 'NONE',  ( 58.75000000000000711, 1.022750809560622143, 1.571497941947222365 ) ) ;
#3505=EDGE_CURVE ( 'NONE', #3662, #19199, #24031, .T. ) ;
#3507=CIRCLE ( 'NONE', #16677, 0.09999999999999983902 ) ;
#3509=EDGE_CURVE ( 'NONE', #20749, #22845, #219, .T. ) ;
#3512=CARTESIAN_POINT ( 'NONE',  ( 58.75000000000002132, -0.4999999999991823207, -1.863080903343696137 ) ) ;
#3523=EDGE_CURVE ( 'NONE', #27109, #7871, #8782, .T. ) ;
#3524=( BOUNDED_CURVE ( )  B_SPLINE_CURVE ( 3, ( #10140, #17268, #321, #9689 ),
 .UNSPECIFIED., .F., .T. ) 
 B_SPLINE_CURVE_WITH_KNOTS ( ( 4, 4 ),
 ( 1.982313172862383510, 2.241731514487931065 ),
 .UNSPECIFIED. ) 
 CURVE ( )  GEOMETRIC_REPRESENTATION_ITEM ( )  RATIONAL_B_SPLINE_CURVE ( ( 1.000000000000000000, 0.9943997021150918769, 0.9943997021150918769, 1.000000000000000000 ) ) 
 REPRESENTATION_ITEM ( '' )  );
#3527=DIRECTION ( 'NONE',  ( 0.000000000000000000, 0.000000000000000000, 1.000000000000000000 ) ) ;
#3537=ORIENTED_EDGE ( 'NONE', *, *, #6553, .T. ) ;
#3546=EDGE_CURVE ( 'NONE', #3048, #28401, #4252, .T. ) ;
#3552=CARTESIAN_POINT ( 'NONE',  ( 58.75000000000000711, 1.394635017529601617, -1.253243060177046564 ) ) ;
#3553=LINE ( 'NONE', #30130, #21611 ) ;
#3554=CIRCLE ( 'NONE', #1024, 2.000000000000000000 ) ;
#3561=EDGE_CURVE ( 'NONE', #4172, #28052, #431, .T. ) ;
#3563=LINE ( 'NONE', #19876, #12364 ) ;
#3569=CARTESIAN_POINT ( 'NONE',  ( 58.64999999999999858, 1.877732920581272058, 0.6121634413844395661 ) ) ;
#3570=ORIENTED_EDGE ( 'NONE', *, *, #10028, .T. ) ;
#3573=CARTESIAN_POINT ( 'NONE',  ( 60.81468257897371643, 0.5000000000006363798, 1.863080903344385586 ) ) ;
#3579=CARTESIAN_POINT ( 'NONE',  ( 58.65000038048046349, 1.383507098107668476, 1.265626441016067805 ) ) ;
#3584=DIRECTION ( 'NONE',  ( 1.000000000000000000, 1.047444401652940007E-14, -0.000000000000000000 ) ) ;
#3593=ORIENTED_EDGE ( 'NONE', *, *, #14187, .T. ) ;
#3595=CYLINDRICAL_SURFACE ( 'NONE', #8231, 0.1500000000000001887 ) ;
#3598=VERTEX_POINT ( 'NONE', #24198 ) ;
#3605=EDGE_LOOP ( 'NONE', ( #28850, #1164, #16168, #20608, #16024, #7000, #4024, #15605, #10838, #27110, #3468, #15958, #18199, #1781, #6627, #26607, #3570, #20339, #27784, #23267, #6999, #2962, #26412, #22336, #26949, #4513, #20403, #28216, #3090, #10562 ) ) ;
#3608=CARTESIAN_POINT ( 'NONE',  ( 58.75000000000000711, 1.655311165517640459, -1.077297519404307957 ) ) ;
#3611=CARTESIAN_POINT ( 'NONE',  ( 51.89360908398616345, -0.6611756245529596399, 1.497563819582714340 ) ) ;
#3622=CARTESIAN_POINT ( 'NONE',  ( 58.74160516400041843, -1.872695119588361212, 0.09319124196129820181 ) ) ;
#3624=ORIENTED_EDGE ( 'NONE', *, *, #18111, .F. ) ;
#3630=ORIENTED_EDGE ( 'NONE', *, *, #23122, .F. ) ;
#3634=LINE ( 'NONE', #18223, #6547 ) ;
#3638=EDGE_CURVE ( 'NONE', #4925, #7153, #27006, .T. ) ;
#3645=DIRECTION ( 'NONE',  ( 1.000000000000000000, 1.047444401652940007E-14, 0.000000000000000000 ) ) ;
#3647=EDGE_CURVE ( 'NONE', #8649, #19299, #20456, .T. ) ;
#3649=DIRECTION ( 'NONE',  ( 1.000000000000000000, 1.047444401652940007E-14, 0.000000000000000000 ) ) ;
#3650=CARTESIAN_POINT ( 'NONE',  ( 58.65000000000004121, -1.834410884275005094, -0.3880228184670952429 ) ) ;
#3652=LINE ( 'NONE', #10480, #21571 ) ;
#3659=CARTESIAN_POINT ( 'NONE',  ( 58.74160516400053211, 1.833004249033624022, 0.3946733352257345007 ) ) ;
#3661=CARTESIAN_POINT ( 'NONE',  ( 61.25000000000003553, -0.9999999999993586242, -1.586072192556190252 ) ) ;
#3662=VERTEX_POINT ( 'NONE', #25703 ) ;
#3665=ORIENTED_EDGE ( 'NONE', *, *, #21632, .T. ) ;
#3668=ADVANCED_FACE ( 'NONE', ( #23025 ), #6795, .F. ) ;
#3675=ORIENTED_EDGE ( 'NONE', *, *, #11181, .F. ) ;
#3676=EDGE_CURVE ( 'NONE', #29895, #7647, #26502, .T. ) ;
#3679=CARTESIAN_POINT ( 'NONE',  ( 58.66120520918180858, 0.4851952615770047106, -1.811135157337470991 ) ) ;
#3681=AXIS2_PLACEMENT_3D ( 'NONE', #11928, #26491, #30935 ) ;
#3685=DIRECTION ( 'NONE',  ( 0.000000000000000000, 0.000000000000000000, 1.000000000000000000 ) ) ;
#3688=CARTESIAN_POINT ( 'NONE',  ( 51.12687253673779253, 0.9194130538826106314, 1.491219977510798156 ) ) ;
#3689=DIRECTION ( 'NONE',  ( 1.000000000000000000, 1.047444401652940007E-14, 0.000000000000000000 ) ) ;
#3690=CARTESIAN_POINT ( 'NONE',  ( 58.65838214097816206, -1.640356269755633534, -0.9083679987359125629 ) ) ;
#3691=DIRECTION ( 'NONE',  ( 0.000000000000000000, 0.000000000000000000, 1.000000000000000000 ) ) ;
#3695=CARTESIAN_POINT ( 'NONE',  ( 58.65000000000003411, -1.022750809560422747, 1.571497941946552457 ) ) ;
#3698=AXIS2_PLACEMENT_3D ( 'NONE', #5324, #17852, #27489 ) ;
#3699=CARTESIAN_POINT ( 'NONE',  ( 61.22030551133023835, 0.7785732690203674977, -1.430137637026578146 ) ) ;
#3702=ORIENTED_EDGE ( 'NONE', *, *, #28456, .F. ) ;
#3708=DIRECTION ( 'NONE',  ( 1.000000000000000000, 1.047444401652940007E-14, 0.000000000000000000 ) ) ;
#3717=CARTESIAN_POINT ( 'NONE',  ( 58.72200624034169891, 1.310319377727330536, 1.341335979947728241 ) ) ;
#3721=CARTESIAN_POINT ( 'NONE',  ( 51.13989201884552926, -0.9305404255924549783, 1.499649012356545130 ) ) ;
#3727=DIRECTION ( 'NONE',  ( 0.000000000000000000, 0.000000000000000000, 1.000000000000000000 ) ) ;
#3732=ORIENTED_EDGE ( 'NONE', *, *, #2379, .T. ) ;
#3737=ORIENTED_EDGE ( 'NONE', *, *, #10619, .F. ) ;
#3750=CARTESIAN_POINT ( 'NONE',  ( 58.75000000000000000, 1.571497941947157972, -1.022750809561051133 ) ) ;
#3762=EDGE_CURVE ( 'NONE', #23733, #27840, #7293, .T. ) ;
#3763=DIRECTION ( 'NONE',  ( 1.000000000000000000, 1.047444401652940007E-14, 0.000000000000000000 ) ) ;
#3765=DIRECTION ( 'NONE',  ( 0.000000000000000000, 0.000000000000000000, 1.000000000000000000 ) ) ;
#3767=CARTESIAN_POINT ( 'NONE',  ( 58.72200624034164207, 1.612834625125591614, 0.9564954546397232971 ) ) ;
#3769=CARTESIAN_POINT ( 'NONE',  ( 51.45655683570191741, -0.9591657938390834026, 1.611094652690528095 ) ) ;
#3771=PLANE ( 'NONE',  #6068 ) ;
#3773=ORIENTED_EDGE ( 'NONE', *, *, #24286, .T. ) ;
#3779=CARTESIAN_POINT ( 'NONE',  ( 58.65000000000000568, 1.022750809560621699, 1.571497941947222587 ) ) ;
#3787=DIRECTION ( 'NONE',  ( 1.000000000000000000, 1.047444401652940007E-14, 0.000000000000000000 ) ) ;
#3802=CARTESIAN_POINT ( 'NONE',  ( 61.25000000000002132, 6.415596960124259844E-13, 3.111507638930570854E-58 ) ) ;
#3815=CARTESIAN_POINT ( 'NONE',  ( 50.25000000000000000, 1.499837071478580919, -1.323060376180706710 ) ) ;
#3816=CIRCLE ( 'NONE', #21546, 0.1500000000000001887 ) ;
#3821=ORIENTED_EDGE ( 'NONE', *, *, #13783, .F. ) ;
#3829=ORIENTED_EDGE ( 'NONE', *, *, #25537, .F. ) ;
#3834=CARTESIAN_POINT ( 'NONE',  ( 58.65000090395037802, 0.5493607500728427961, -1.793027323413543650 ) ) ;
#3837=CARTESIAN_POINT ( 'NONE',  ( 51.25000000000002842, -1.487499999999465361, 1.821662113731690703E-16 ) ) ;
#3849=CARTESIAN_POINT ( 'NONE',  ( 58.73371041428932671, -1.582294810366662308, -1.006219588948326304 ) ) ;
#3852=EDGE_CURVE ( 'NONE', #207, #15867, #9041, .T. ) ;
#3855=CARTESIAN_POINT ( 'NONE',  ( 51.59739104186227365, 1.010292945603182169, -1.272765950230260401 ) ) ;
#3858=CIRCLE ( 'NONE', #311, 0.1500000000000001887 ) ;
#3870=CARTESIAN_POINT ( 'NONE',  ( 51.13585994975460380, 0.9262448312174480503, -1.518514878530177192 ) ) ;
#3875=EDGE_LOOP ( 'NONE', ( #1794, #15851, #2274, #3593 ) ) ;
#3877=CARTESIAN_POINT ( 'NONE',  ( 50.25000000000004263, -1.960427193528405887, -0.3958853607747112036 ) ) ;
#3882=CARTESIAN_POINT ( 'NONE',  ( 58.75000000000001421, 1.253243060177670509, 1.394635017528978560 ) ) ;
#3885=VECTOR ( 'NONE', #2214, 1000.000000000000000 ) ;
#3886=DIRECTION ( 'NONE',  ( 0.000000000000000000, 0.000000000000000000, 1.000000000000000000 ) ) ;
#3894=CARTESIAN_POINT ( 'NONE',  ( 50.25000000000002842, -1.106298139390672564, 1.666164585743104443 ) ) ;
#3906=ORIENTED_EDGE ( 'NONE', *, *, #18111, .T. ) ;
#3909=CIRCLE ( 'NONE', #18569, 0.1500000000000000777 ) ;
#3912=AXIS2_PLACEMENT_3D ( 'NONE', #16435, #13878, #18982 ) ;
#3913=ORIENTED_EDGE ( 'NONE', *, *, #9715, .F. ) ;
#3915=DIRECTION ( 'NONE',  ( 1.000000000000000000, 1.047444401652940007E-14, 0.000000000000000000 ) ) ;
#3919=DIRECTION ( 'NONE',  ( 0.5633368246415176861, -0.8262273428075422865, 0.000000000000000000 ) ) ;
#3922=CARTESIAN_POINT ( 'NONE',  ( 52.20711756518982583, 0.7500000000005468959, -1.718465885608440269 ) ) ;
#3923=AXIS2_PLACEMENT_3D ( 'NONE', #2419, #9709, #7317 ) ;
#3933=CARTESIAN_POINT ( 'NONE',  ( 51.24099374247644789, 1.086790822299315895, 1.208135181987621598 ) ) ;
#3936=ORIENTED_EDGE ( 'NONE', *, *, #5923, .F. ) ;
#3942=ORIENTED_EDGE ( 'NONE', *, *, #19332, .F. ) ;
#3944=EDGE_CURVE ( 'NONE', #22261, #10512, #26962, .T. ) ;
#3958=CARTESIAN_POINT ( 'NONE',  ( 50.25000000000004263, -2.079005547593277381, 1.932245437381540134E-15 ) ) ;
#3962=CARTESIAN_POINT ( 'NONE',  ( 58.65000045311414567, -1.787855644601539451, -0.5652242121843152889 ) ) ;
#3968=DIRECTION ( 'NONE',  ( 0.000000000000000000, 0.000000000000000000, 1.000000000000000000 ) ) ;
#3970=( BOUNDED_SURFACE ( )  B_SPLINE_SURFACE ( 3, 2, ( 
 ( #8463, #18141, #27780 ),
 ( #25395, #3699, #23031 ),
 ( #10995, #25542, #13512 ),
 ( #16854, #7503, #4322 ),
 ( #21306, #19239, #28555 ),
 ( #1961, #9578, #26661 ) ),
 .UNSPECIFIED., .F., .F., .F. ) 
 B_SPLINE_SURFACE_WITH_KNOTS ( ( 4, 2, 4 ),
 ( 3, 3 ),
 ( 5.963111948670274387E-19, 0.0002090583013612447186, 0.0004181166027224888409 ),
 ( 0.000000000000000000, 1.000000000000000000 ),
 .UNSPECIFIED. ) 
 GEOMETRIC_REPRESENTATION_ITEM ( )  RATIONAL_B_SPLINE_SURFACE ( (
 ( 1.000000000000000000, 0.7071067811865358044, 1.000000000000000000),
 ( 1.000000000000000000, 0.7521684882082442236, 1.000000000000000000),
 ( 1.000000000000000000, 0.7851308282770599334, 1.000000000000000000),
 ( 1.000000000000000000, 0.8276934144745562438, 1.000000000000000000),
 ( 1.000000000000000000, 0.8364441017664440148, 1.000000000000000000),
 ( 1.000000000000000000, 0.8366600265340728981, 1.000000000000000000) ) ) 
 REPRESENTATION_ITEM ( '' )  SURFACE ( )  );
#3973=CARTESIAN_POINT ( 'NONE',  ( 58.65263613458532888, 1.827305695291647547, 0.4205413283056451679 ) ) ;
#3980=ORIENTED_EDGE ( 'NONE', *, *, #10979, .T. ) ;
#4002=DIRECTION ( 'NONE',  ( 1.000000000000000000, 1.047444401652940007E-14, 0.000000000000000000 ) ) ;
#4008=CARTESIAN_POINT ( 'NONE',  ( 58.65000000000004121, -1.671477153793431647, -0.8495817349405304642 ) ) ;
#4024=ORIENTED_EDGE ( 'NONE', *, *, #30577, .T. ) ;
#4025=AXIS2_PLACEMENT_3D ( 'NONE', #13563, #15794, #28134 ) ;
#4026=CARTESIAN_POINT ( 'NONE',  ( 58.66122797211809825, -1.632010475557796214, 0.9232791089888466862 ) ) ;
#4027=PLANE ( 'NONE',  #23546 ) ;
#4031=EDGE_CURVE ( 'NONE', #22261, #28405, #29006, .T. ) ;
#4033=ORIENTED_EDGE ( 'NONE', *, *, #4819, .T. ) ;
#4036=( BOUNDED_SURFACE ( )  B_SPLINE_SURFACE ( 3, 2, ( 
 ( #6147, #15488, #25146 ),
 ( #12944, #3611, #1081 ),
 ( #3466, #30207, #934 ),
 ( #22638, #10731, #10586 ) ),
 .UNSPECIFIED., .F., .F., .F. ) 
 B_SPLINE_SURFACE_WITH_KNOTS ( ( 4, 4 ),
 ( 3, 3 ),
 ( 1.982313172862383066, 2.241731514487931065 ),
 ( 0.000000000000000000, 1.000000000000000000 ),
 .UNSPECIFIED. ) 
 GEOMETRIC_REPRESENTATION_ITEM ( )  RATIONAL_B_SPLINE_SURFACE ( (
 ( 1.000000000000000000, 0.8156258140602881124, 1.000000000000000000),
 ( 1.000000000000000000, 0.8356979842195455532, 1.000000000000000000),
 ( 1.000000000000000000, 0.8538860448759181265, 1.000000000000000000),
 ( 1.000000000000000000, 0.8699658093904938383, 1.000000000000000000) ) ) 
 REPRESENTATION_ITEM ( '' )  SURFACE ( )  );
#4037=CARTESIAN_POINT ( 'NONE',  ( 51.45655683570191741, -0.9591657938390827365, -1.468576096419532018 ) ) ;
#4052=CARTESIAN_POINT ( 'NONE',  ( 51.39880079787599243, -0.9985449105385801882, 1.587650281084739712 ) ) ;
#4055=FACE_OUTER_BOUND ( 'NONE', #31072, .T. ) ;
#4061=ORIENTED_EDGE ( 'NONE', *, *, #28959, .T. ) ;
#4062=ORIENTED_EDGE ( 'NONE', *, *, #9263, .T. ) ;
#4069=CARTESIAN_POINT ( 'NONE',  ( 58.75000000000002132, 6.153735859711025284E-13, 3.111507638930570854E-58 ) ) ;
#4070=ORIENTED_EDGE ( 'NONE', *, *, #8587, .F. ) ;
#4073=CARTESIAN_POINT ( 'NONE',  ( 58.65000045311409593, 1.830940512617971194, -0.4044292957139257183 ) ) ;
#4083=CARTESIAN_POINT ( 'NONE',  ( 61.00000000000001421, 1.000000000000639044, -1.586072192556190474 ) ) ;
#4084=AXIS2_PLACEMENT_3D ( 'NONE', #24707, #26781, #4926 ) ;
#4089=VERTEX_POINT ( 'NONE', #13293 ) ;
#4094=DIRECTION ( 'NONE',  ( 0.000000000000000000, 0.9783524716138816135, -0.2069455031814148027 ) ) ;
#4095=CARTESIAN_POINT ( 'NONE',  ( 58.65263613458535019, -1.277852321299179916, 1.372222488448882727 ) ) ;
#4106=EDGE_CURVE ( 'NONE', #26655, #23063, #26472, .T. ) ;
#4112=CARTESIAN_POINT ( 'NONE',  ( 61.23770293222991512, 0.8897917884447287262, -1.791164585742097914 ) ) ;
#4126=DIRECTION ( 'NONE',  ( 0.000000000000000000, 0.000000000000000000, 1.000000000000000000 ) ) ;
#4131=EDGE_CURVE ( 'NONE', #30566, #16027, #1685, .T. ) ;
#4134=CARTESIAN_POINT ( 'NONE',  ( 52.06628335902946247, -0.5434431642975677823, -1.996089927833914146 ) ) ;
#4138=DIRECTION ( 'NONE',  ( 2.616380615828677096E-15, -0.2069455031823360380, -0.9783524716136868804 ) ) ;
#4151=FACE_OUTER_BOUND ( 'NONE', #15246, .T. ) ;
#4165=CARTESIAN_POINT ( 'NONE',  ( 51.45655683570191741, -0.9591657938390835136, -1.468576096419531574 ) ) ;
#4169=ORIENTED_EDGE ( 'NONE', *, *, #22608, .T. ) ;
#4171=FACE_OUTER_BOUND ( 'NONE', #19072, .T. ) ;
#4172=VERTEX_POINT ( 'NONE', #27415 ) ;
#4173=CARTESIAN_POINT ( 'NONE',  ( 51.13858604272871133, 1.070913481529462086, -1.222302725805713308 ) ) ;
#4179=EDGE_CURVE ( 'NONE', #7044, #17335, #18893, .T. ) ;
#4193=CARTESIAN_POINT ( 'NONE',  ( 58.74999999305997278, -0.9423072185570646742, 1.683452862813170636 ) ) ;
#4195=DIRECTION ( 'NONE',  ( 0.000000000000000000, 0.000000000000000000, 1.000000000000000000 ) ) ;
#4201=EDGE_LOOP ( 'NONE', ( #3773, #1603, #18562, #21804 ) ) ;
#4204=VERTEX_POINT ( 'NONE', #28201 ) ;
#4210=ORIENTED_EDGE ( 'NONE', *, *, #23209, .T. ) ;
#4212=ORIENTED_EDGE ( 'NONE', *, *, #29857, .F. ) ;
#4214=ORIENTED_EDGE ( 'NONE', *, *, #17708, .T. ) ;
#4221=CARTESIAN_POINT ( 'NONE',  ( 58.75000018803716273, 1.882836145343370404, -0.4533061784665026739 ) ) ;
#4224=VECTOR ( 'NONE', #16333, 1000.000000000000000 ) ;
#4227=CARTESIAN_POINT ( 'NONE',  ( 50.59602332238209499, 0.1408342061609074158, -1.212874140286673841 ) ) ;
#4237=EDGE_CURVE ( 'NONE', #10792, #4826, #31036, .T. ) ;
#4240=ORIENTED_EDGE ( 'NONE', *, *, #31187, .F. ) ;
#4243=CARTESIAN_POINT ( 'NONE',  ( 58.65844932252372246, 0.9660788770032745498, -1.607045716458365581 ) ) ;
#4247=DIRECTION ( 'NONE',  ( 2.475188721679744024E-12, -0.7438053426811914726, -0.6683962987621305807 ) ) ;
#4248=DIRECTION ( 'NONE',  ( 0.000000000000000000, 0.000000000000000000, 1.000000000000000000 ) ) ;
#4249=CARTESIAN_POINT ( 'NONE',  ( 61.05455829109366306, 0.5997039666881081033, -1.862468256791881327 ) ) ;
#4252=CIRCLE ( 'NONE', #14870, 0.1500000000000001887 ) ;
#4265=DIRECTION ( 'NONE',  ( 0.000000000000000000, -1.000000000000000000, 0.000000000000000000 ) ) ;
#4268=CARTESIAN_POINT ( 'NONE',  ( 58.73371041428929118, -1.788808215311387118, -0.5624054559931295216 ) ) ;
#4273=VERTEX_POINT ( 'NONE', #4599 ) ;
#4280=AXIS2_PLACEMENT_3D ( 'NONE', #9088, #28402, #28073 ) ;
#4289=CARTESIAN_POINT ( 'NONE',  ( 60.75000000000001421, 1.000000000000636380, -1.996089927833914146 ) ) ;
#4296=VERTEX_POINT ( 'NONE', #2218 ) ;
#4301=DIRECTION ( 'NONE',  ( 1.000000000000000000, 1.047444401652940007E-14, 0.000000000000000000 ) ) ;
#4304=AXIS2_PLACEMENT_3D ( 'NONE', #12089, #10484, #10314 ) ;
#4312=CARTESIAN_POINT ( 'NONE',  ( 58.72427158855725793, -1.646019958200114486, -0.8981388483283767599 ) ) ;
#4316=ORIENTED_EDGE ( 'NONE', *, *, #29166, .T. ) ;
#4322=CARTESIAN_POINT ( 'NONE',  ( 61.02708519082499095, 0.5631634571416959112, -1.705199831323242821 ) ) ;
#4324=ORIENTED_EDGE ( 'NONE', *, *, #23356, .T. ) ;
#4330=CARTESIAN_POINT ( 'NONE',  ( 51.31802667458094902, 1.005866567097610575, -1.281163073955430720 ) ) ;
#4338=VERTEX_POINT ( 'NONE', #20924 ) ;
#4346=LINE ( 'NONE', #28577, #272 ) ;
#4347=CARTESIAN_POINT ( 'NONE',  ( 58.65000000000002700, -0.6121634413827002907, 1.877732920581024700 ) ) ;
#4348=DIRECTION ( 'NONE',  ( -1.000000000000000000, -1.047444401652940007E-14, -0.000000000000000000 ) ) ;
#4350=CARTESIAN_POINT ( 'NONE',  ( 58.75000000000002132, -0.5933363752205416120, 1.867039175319914923 ) ) ;
#4351=CARTESIAN_POINT ( 'NONE',  ( 58.65000000000002700, -0.8495817349410276220, 1.671477153793481163 ) ) ;
#4359=EDGE_CURVE ( 'NONE', #22738, #8786, #4638, .T. ) ;
#4361=CIRCLE ( 'NONE', #25107, 0.1500000000000002720 ) ;
#4362=AXIS2_PLACEMENT_3D ( 'NONE', #4779, #9073, #14440 ) ;
#4365=AXIS2_PLACEMENT_3D ( 'NONE', #15295, #30004, #18307 ) ;
#4375=EDGE_CURVE ( 'NONE', #5258, #36, #1805, .T. ) ;
#4383=DIRECTION ( 'NONE',  ( 0.000000000000000000, 0.000000000000000000, 1.000000000000000000 ) ) ;
#4387=DIRECTION ( 'NONE',  ( 1.000000000000000000, 1.047444401652940007E-14, 0.000000000000000000 ) ) ;
#4389=CIRCLE ( 'NONE', #22596, 1.875000000000001776 ) ;
#4393=TOROIDAL_SURFACE ( 'NONE', #29169, 1.975000000000001865, 0.1000000000000000056 ) ;
#4397=EDGE_CURVE ( 'NONE', #7031, #22738, #16121, .T. ) ;
#4402=EDGE_CURVE ( 'NONE', #27109, #8262, #166, .T. ) ;
#4404=CIRCLE ( 'NONE', #2892, 0.1500000000000001887 ) ;
#4406=DIRECTION ( 'NONE',  ( 1.000000000000000000, 1.047444401652940007E-14, 0.000000000000000000 ) ) ;
#4411=CARTESIAN_POINT ( 'NONE',  ( 58.65838214097848891, 0.9083679987363961761, -1.640356269756322094 ) ) ;
#4419=SPHERICAL_SURFACE ( 'NONE', #25150, 0.2500000000000000000 ) ;
#4422=ORIENTED_EDGE ( 'NONE', *, *, #1967, .F. ) ;
#4429=EDGE_CURVE ( 'NONE', #14364, #23034, #5489, .T. ) ;
#4433=AXIS2_PLACEMENT_3D ( 'NONE', #7560, #29530, #9929 ) ;
#4452=VERTEX_POINT ( 'NONE', #24386 ) ;
#4455=VECTOR ( 'NONE', #27653, 1000.000000000000000 ) ;
#4457=CARTESIAN_POINT ( 'NONE',  ( 58.72219294808260770, 0.5000000000006150636, 1.828782891498946350 ) ) ;
#4458=ORIENTED_EDGE ( 'NONE', *, *, #20222, .F. ) ;
#4465=B_SPLINE_CURVE_WITH_KNOTS ( 'NONE', 3,
 ( #18842, #4249, #13893, #11554 ),
 .UNSPECIFIED., .F., .F.,
 ( 4, 4 ),
 ( 0.000000000000000000, 0.0001886355468578361809 ),
 .UNSPECIFIED. ) ;
#4487=DIRECTION ( 'NONE',  ( 1.000000000000000000, 1.047444401652940007E-14, 0.000000000000000000 ) ) ;
#4488=CARTESIAN_POINT ( 'NONE',  ( 58.75000000000002132, 6.153735859711025284E-13, 3.111507638930570854E-58 ) ) ;
#4490=DIRECTION ( 'NONE',  ( -9.958586508671106819E-15, 0.9507508458640636650, -0.3099561728515299319 ) ) ;
#4499=DIRECTION ( 'NONE',  ( -9.994490842163784987E-15, 0.7438053426821212843, -0.6683962987610958528 ) ) ;
#4500=CIRCLE ( 'NONE', #16123, 0.2499999999999986955 ) ;
#4502=ORIENTED_EDGE ( 'NONE', *, *, #15891, .T. ) ;
#4507=ORIENTED_EDGE ( 'NONE', *, *, #19286, .T. ) ;
#4508=ADVANCED_FACE ( 'NONE', ( #314 ), #24693, .F. ) ;
#4509=CARTESIAN_POINT ( 'NONE',  ( 50.25000000000000711, 1.106298139390723190, -1.666164585742097914 ) ) ;
#4513=ORIENTED_EDGE ( 'NONE', *, *, #7852, .T. ) ;
#4516=DIRECTION ( 'NONE',  ( 0.000000000000000000, 0.000000000000000000, 1.000000000000000000 ) ) ;
#4520=CARTESIAN_POINT ( 'NONE',  ( 58.65000000000005542, -1.827356000909702294, -0.4213753797513699051 ) ) ;
#4521=CARTESIAN_POINT ( 'NONE',  ( 58.75000000000002132, -0.4999999999991334154, 1.863080903344709549 ) ) ;
#4525=CARTESIAN_POINT ( 'NONE',  ( 61.25000000000002132, 6.415596960124259844E-13, 3.111507638930570854E-58 ) ) ;
#4528=ORIENTED_EDGE ( 'NONE', *, *, #3455, .F. ) ;
#4535=EDGE_CURVE ( 'NONE', #4273, #4826, #11537, .T. ) ;
#4541=CARTESIAN_POINT ( 'NONE',  ( 61.25000000000004263, -1.470078920827193825, -1.320078920827526758 ) ) ;
#4543=VERTEX_POINT ( 'NONE', #23114 ) ;
#4546=AXIS2_PLACEMENT_3D ( 'NONE', #31003, #9324, #18989 ) ;
#4558=AXIS2_PLACEMENT_3D ( 'NONE', #3252, #29850, #17676 ) ;
#4569=CARTESIAN_POINT ( 'NONE',  ( 58.65000000000003411, -1.394635017527501297, 1.253243060178016899 ) ) ;
#4571=EDGE_LOOP ( 'NONE', ( #27306, #2557, #12420 ) ) ;
#4572=AXIS2_PLACEMENT_3D ( 'NONE', #20687, #5956, #20524 ) ;
#4574=CARTESIAN_POINT ( 'NONE',  ( 58.65000000000002700, -0.5811678240974692544, 1.782657835994643447 ) ) ;
#4575=CARTESIAN_POINT ( 'NONE',  ( 58.72427158855730767, 0.9764256747737051212, 1.600821037878903619 ) ) ;
#4581=EDGE_CURVE ( 'NONE', #7044, #8649, #8072, .T. ) ;
#4584=CARTESIAN_POINT ( 'NONE',  ( 61.25000000000003553, -1.323060376180724029, -1.499837071477706729 ) ) ;
#4585=ADVANCED_FACE ( 'NONE', ( #3157 ), #12078, .F. ) ;
#4586=VERTEX_POINT ( 'NONE', #951 ) ;
#4590=CARTESIAN_POINT ( 'NONE',  ( 61.25000000000002132, 6.415596960124259844E-13, 3.111507638930570854E-58 ) ) ;
#4592=CARTESIAN_POINT ( 'NONE',  ( 51.23644008536122385, 1.080112125196981854, 1.214076932077872817 ) ) ;
#4596=CARTESIAN_POINT ( 'NONE',  ( 60.81561938753820584, -0.6499999999993623101, 1.489337100860648633 ) ) ;
#4599=CARTESIAN_POINT ( 'NONE',  ( 52.06628335902946247, -0.5434431642975682264, 1.794517909405659806 ) ) ;
#4610=CARTESIAN_POINT ( 'NONE',  ( 58.74840439586692753, 0.5000000000006153966, 1.859896009349663037 ) ) ;
#4614=CARTESIAN_POINT ( 'NONE',  ( 58.75000000000002132, -0.5380862305903428844, -2.008165151418244143 ) ) ;
#4617=EDGE_CURVE ( 'NONE', #28052, #22181, #26217, .T. ) ;
#4618=ORIENTED_EDGE ( 'NONE', *, *, #29522, .T. ) ;
#4632=CARTESIAN_POINT ( 'NONE',  ( 58.66133336607604321, -1.348863877412392664, -1.302803168107730114 ) ) ;
#4633=CARTESIAN_POINT ( 'NONE',  ( 60.81472790383496374, -0.4999999999993504640, 1.863080903340958328 ) ) ;
#4634=CARTESIAN_POINT ( 'NONE',  ( 61.25000000000004263, -1.800471618824186493, -1.039502773796582069 ) ) ;
#4638=B_SPLINE_CURVE_WITH_KNOTS ( 'NONE', 3,
 ( #17409, #26770, #4745, #17123, #29432, #21879 ),
 .UNSPECIFIED., .F., .F.,
 ( 4, 2, 4 ),
 ( 0.000000000000000000, 0.0001939776071359005987, 0.0003879552142718011975 ),
 .UNSPECIFIED. ) ;
#4639=DIRECTION ( 'NONE',  ( 1.000000000000000000, 1.047444401652940007E-14, 0.000000000000000000 ) ) ;
#4642=ORIENTED_EDGE ( 'NONE', *, *, #5312, .F. ) ;
#4643=ADVANCED_FACE ( 'NONE', ( #18674 ), #26260, .T. ) ;
#4644=CARTESIAN_POINT ( 'NONE',  ( 52.10126625705170511, 0.5195911883743922210, 1.546252172343136388 ) ) ;
#4647=ORIENTED_EDGE ( 'NONE', *, *, #1847, .T. ) ;
#4648=VERTEX_POINT ( 'NONE', #28156 ) ;
#4653=VECTOR ( 'NONE', #28419, 1000.000000000000000 ) ;
#4657=CYLINDRICAL_SURFACE ( 'NONE', #19757, 0.1499999999999999667 ) ;
#4663=CARTESIAN_POINT ( 'NONE',  ( 58.65000045311413146, -0.8645309767535818146, -1.663878723407328897 ) ) ;
#4671=DIRECTION ( 'NONE',  ( 0.000000000000000000, 0.000000000000000000, 1.000000000000000000 ) ) ;
#4672=ORIENTED_EDGE ( 'NONE', *, *, #10728, .F. ) ;
#4676=( BOUNDED_CURVE ( )  B_SPLINE_CURVE ( 3, ( #3688, #20662, #25529, #10671 ),
 .UNSPECIFIED., .F., .T. ) 
 B_SPLINE_CURVE_WITH_KNOTS ( ( 4, 4 ),
 ( 1.817784745758538767, 2.232964403949253107 ),
 .UNSPECIFIED. ) 
 CURVE ( )  GEOMETRIC_REPRESENTATION_ITEM ( )  RATIONAL_B_SPLINE_CURVE ( ( 1.000000000000000000, 0.9856869983806465507, 0.9856869983806465507, 1.000000000000000000 ) ) 
 REPRESENTATION_ITEM ( '' )  );
#4687=VERTEX_POINT ( 'NONE', #15959 ) ;
#4690=B_SPLINE_CURVE_WITH_KNOTS ( 'NONE', 3,
 ( #27638, #3260, #27172, #12598, #7842, #21713 ),
 .UNSPECIFIED., .F., .F.,
 ( 4, 2, 4 ),
 ( 0.000000000000000000, 0.0001000270069607746585, 0.0002000540139215493170 ),
 .UNSPECIFIED. ) ;
#4699=AXIS2_PLACEMENT_3D ( 'NONE', #7963, #367, #27273 ) ;
#4705=DIRECTION ( 'NONE',  ( 0.000000000000000000, 0.000000000000000000, 1.000000000000000000 ) ) ;
#4713=ORIENTED_EDGE ( 'NONE', *, *, #62, .F. ) ;
#4714=CARTESIAN_POINT ( 'NONE',  ( 51.01608411450973080, -0.7569233679470204201, 1.030722644926826748 ) ) ;
#4716=CARTESIAN_POINT ( 'NONE',  ( 58.64999999999991331, -0.8948927608045756932, 1.760622601995819325 ) ) ;
#4717=CARTESIAN_POINT ( 'NONE',  ( 58.65844932252329613, 0.9087029769946789459, 1.640171707773312004 ) ) ;
#4735=DIRECTION ( 'NONE',  ( 0.5633368246414943714, 0.8262273428075581627, 0.000000000000000000 ) ) ;
#4736=AXIS2_PLACEMENT_3D ( 'NONE', #28115, #25898, #13840 ) ;
#4742=FACE_OUTER_BOUND ( 'NONE', #29851, .T. ) ;
#4745=CARTESIAN_POINT ( 'NONE',  ( 60.97363240180332156, 0.7541976959284683035, 1.440084173506624321 ) ) ;
#4751=AXIS2_PLACEMENT_3D ( 'NONE', #29252, #9485, #26407 ) ;
#4753=CARTESIAN_POINT ( 'NONE',  ( 61.25000000000001421, 1.000000000000641709, -1.655766640117574795 ) ) ;
#4766=AXIS2_PLACEMENT_3D ( 'NONE', #20893, #30523, #13736 ) ;
#4770=CARTESIAN_POINT ( 'NONE',  ( 58.75000000000000711, 1.760622601997809955, -0.8948927608024527247 ) ) ;
#4779=CARTESIAN_POINT ( 'NONE',  ( 58.75000000000002132, 6.153735859711025284E-13, 3.111507638930570854E-58 ) ) ;
#4780=CARTESIAN_POINT ( 'NONE',  ( 58.75000000000002842, -1.039502773796102897, -1.800471618824325493 ) ) ;
#4784=CARTESIAN_POINT ( 'NONE',  ( 60.75000000000001421, 0.5000000000006363798, -1.863080903343375061 ) ) ;
#4790=DIRECTION ( 'NONE',  ( 0.000000000000000000, -0.7438053426816512159, -0.6683962987616188789 ) ) ;
#4791=EDGE_CURVE ( 'NONE', #585, #8786, #7151, .T. ) ;
#4792=ORIENTED_EDGE ( 'NONE', *, *, #20393, .T. ) ;
#4798=ORIENTED_EDGE ( 'NONE', *, *, #3216, .F. ) ;
#4807=AXIS2_PLACEMENT_3D ( 'NONE', #9235, #23954, #20953 ) ;
#4810=B_SPLINE_CURVE_WITH_KNOTS ( 'NONE', 3,
 ( #14608, #17156, #24274, #4632, #14902, #2586 ),
 .UNSPECIFIED., .F., .F.,
 ( 4, 2, 4 ),
 ( 0.000000000000000000, 0.0001000270069604664605, 0.0002000540139209329210 ),
 .UNSPECIFIED. ) ;
#4814=CARTESIAN_POINT ( 'NONE',  ( 50.59602332238209499, 0.1408342061609076379, -0.8215393206232032286 ) ) ;
#4817=EDGE_CURVE ( 'NONE', #11068, #29981, #8929, .T. ) ;
#4819=EDGE_CURVE ( 'NONE', #17369, #4543, #28891, .T. ) ;
#4826=VERTEX_POINT ( 'NONE', #17540 ) ;
#4829=AXIS2_PLACEMENT_3D ( 'NONE', #28719, #26482, #21604 ) ;
#4836=DIRECTION ( 'NONE',  ( 1.000000000000000000, 1.047444401652940007E-14, 0.000000000000000000 ) ) ;
#4837=ORIENTED_EDGE ( 'NONE', *, *, #9226, .F. ) ;
#4838=CIRCLE ( 'NONE', #16483, 0.2500000000000000000 ) ;
#4841=VERTEX_POINT ( 'NONE', #1063 ) ;
#4842=CIRCLE ( 'NONE', #5836, 0.2500000000000000000 ) ;
#4852=CARTESIAN_POINT ( 'NONE',  ( 58.75000000000003553, -1.791164585742486937, -0.8897917884440847969 ) ) ;
#4853=ADVANCED_FACE ( 'NONE', ( #20396 ), #23325, .F. ) ;
#4854=CIRCLE ( 'NONE', #10903, 0.1500000000000001887 ) ;
#4865=ORIENTED_EDGE ( 'NONE', *, *, #26519, .F. ) ;
#4866=DIRECTION ( 'NONE',  ( 0.000000000000000000, 0.000000000000000000, 1.000000000000000000 ) ) ;
#4867=CARTESIAN_POINT ( 'NONE',  ( 58.66107449606997193, 1.349793924523127187, -1.301839550767805331 ) ) ;
#4876=LINE ( 'NONE', #14541, #9630 ) ;
#4882=CARTESIAN_POINT ( 'NONE',  ( 58.75000000000002132, 6.153735859711025284E-13, 3.111507638930570854E-58 ) ) ;
#4888=AXIS2_PLACEMENT_3D ( 'NONE', #9852, #26644, #14752 ) ;
#4892=TOROIDAL_SURFACE ( 'NONE', #14524, 1.975000000000001865, 0.1000000000000000056 ) ;
#4894=ORIENTED_EDGE ( 'NONE', *, *, #13577, .F. ) ;
#4896=DIRECTION ( 'NONE',  ( 1.000000000000000000, 1.047444401652940007E-14, 0.000000000000000000 ) ) ;
#4900=CIRCLE ( 'NONE', #27665, 1.975000000000001865 ) ;
#4911=ADVANCED_FACE ( 'NONE', ( #238 ), #19273, .F. ) ;
#4912=CARTESIAN_POINT ( 'NONE',  ( 58.72200624034184102, -1.816790722507359179, 0.4641018782093048189 ) ) ;
#4916=CARTESIAN_POINT ( 'NONE',  ( 58.68279620299891519, -0.4999999999993856026, -1.809045707182514118 ) ) ;
#4921=ORIENTED_EDGE ( 'NONE', *, *, #909, .F. ) ;
#4922=DIRECTION ( 'NONE',  ( 0.000000000000000000, 0.000000000000000000, 1.000000000000000000 ) ) ;
#4925=VERTEX_POINT ( 'NONE', #2476 ) ;
#4926=DIRECTION ( 'NONE',  ( 0.000000000000000000, 0.000000000000000000, 1.000000000000000000 ) ) ;
#4930=DIRECTION ( 'NONE',  ( 0.000000000000000000, 0.000000000000000000, 1.000000000000000000 ) ) ;
#4931=VERTEX_POINT ( 'NONE', #31286 ) ;
#4934=ORIENTED_EDGE ( 'NONE', *, *, #8258, .F. ) ;
#4944=CARTESIAN_POINT ( 'NONE',  ( 61.23770293222972327, 0.8897917884438596436, 1.791164585743606041 ) ) ;
#4951=DIRECTION ( 'NONE',  ( 1.000000000000000000, 1.047444401652940007E-14, 0.000000000000000000 ) ) ;
#4969=ORIENTED_EDGE ( 'NONE', *, *, #26248, .F. ) ;
#4972=ORIENTED_EDGE ( 'NONE', *, *, #5136, .F. ) ;
#4975=B_SPLINE_CURVE_WITH_KNOTS ( 'NONE', 3,
 ( #21127, #2090, #30759, #30914 ),
 .UNSPECIFIED., .F., .F.,
 ( 4, 4 ),
 ( 0.000000000000000000, 0.0003819718307412712306 ),
 .UNSPECIFIED. ) ;
#4983=CARTESIAN_POINT ( 'NONE',  ( 50.56925576102500486, -0.1015751161694646437, -0.8011113709441625153 ) ) ;
#4988=LINE ( 'NONE', #14643, #5804 ) ;
#4995=ORIENTED_EDGE ( 'NONE', *, *, #29706, .T. ) ;
#4999=CARTESIAN_POINT ( 'NONE',  ( 58.75000000000002842, -0.8897917884436052915, -1.791164585742600179 ) ) ;
#5002=VERTEX_POINT ( 'NONE', #25242 ) ;
#5015=EDGE_CURVE ( 'NONE', #1037, #27051, #3563, .T. ) ;
#5018=FACE_OUTER_BOUND ( 'NONE', #19394, .T. ) ;
#5030=AXIS2_PLACEMENT_3D ( 'NONE', #11374, #4247, #11552 ) ;
#5034=CARTESIAN_POINT ( 'NONE',  ( 58.75000000000000711, 1.470078920827434965, 1.470078920828533420 ) ) ;
#5037=ADVANCED_FACE ( 'NONE', ( #29680 ), #15116, .F. ) ;
#5040=EDGE_CURVE ( 'NONE', #21318, #17938, #2249, .T. ) ;
#5044=DIRECTION ( 'NONE',  ( 2.477824476393711885E-12, -0.8914544820231923294, -0.4531102586355355011 ) ) ;
#5047=EDGE_LOOP ( 'NONE', ( #2585, #2401, #15070, #27283, #20892, #13162, #26022, #2447, #9939, #12246, #25982, #22277, #30857, #28564, #21150, #18575, #25722, #1671, #16223, #177, #14264, #25322 ) ) ;
#5049=CARTESIAN_POINT ( 'NONE',  ( 61.23770293223015670, -0.8897917884444476178, 1.791164585743103999 ) ) ;
#5050=CARTESIAN_POINT ( 'NONE',  ( 52.20711756518983293, 0.5000000000005468959, -1.807104036850122109 ) ) ;
#5062=AXIS2_PLACEMENT_3D ( 'NONE', #29065, #2769, #24320 ) ;
#5067=CYLINDRICAL_SURFACE ( 'NONE', #25621, 1.875000000000001776 ) ;
#5069=ORIENTED_EDGE ( 'NONE', *, *, #8145, .F. ) ;
#5076=LINE ( 'NONE', #9685, #9520 ) ;
#5077=ORIENTED_EDGE ( 'NONE', *, *, #2293, .F. ) ;
#5078=ORIENTED_EDGE ( 'NONE', *, *, #16650, .F. ) ;
#5082=CARTESIAN_POINT ( 'NONE',  ( 58.75000000000002842, -1.039502773796971091, 1.800471618824829756 ) ) ;
#5088=CARTESIAN_POINT ( 'NONE',  ( 58.65000000000003411, -1.253243060177393620, -1.394635017528123688 ) ) ;
#5095=DIRECTION ( 'NONE',  ( 8.860386339788722010E-15, -0.8459051693633015123, 0.5333333333333332149 ) ) ;
#5098=DIRECTION ( 'NONE',  ( 1.000000000000000000, 1.047444401652940007E-14, 0.000000000000000000 ) ) ;
#5102=CARTESIAN_POINT ( 'NONE',  ( 50.25000000000000000, 1.960427193528456069, 0.3958853607757182314 ) ) ;
#5106=CARTESIAN_POINT ( 'NONE',  ( 58.75000000000003553, -1.960427193528576639, 0.3958853607747486181 ) ) ;
#5113=CARTESIAN_POINT ( 'NONE',  ( 61.25000000000003553, -0.9999999999993586242, 1.586072192556190252 ) ) ;
#5120=ORIENTED_EDGE ( 'NONE', *, *, #8315, .F. ) ;
#5130=CARTESIAN_POINT ( 'NONE',  ( 51.45655683570189609, 0.9591657938401632055, -1.468576096419530463 ) ) ;
#5132=DIRECTION ( 'NONE',  ( 1.000000000000000000, 1.047444401652940007E-14, 0.000000000000000000 ) ) ;
#5136=EDGE_CURVE ( 'NONE', #28516, #16439, #10691, .T. ) ;
#5137=CARTESIAN_POINT ( 'NONE',  ( 51.11922224408084503, 0.9310536428531250852, 1.338077479438640971 ) ) ;
#5142=B_SPLINE_CURVE_WITH_KNOTS ( 'NONE', 3,
 ( #26375, #6741, #14331, #16401 ),
 .UNSPECIFIED., .F., .F.,
 ( 4, 4 ),
 ( 0.000000000000000000, 2.862003379465107863E-05 ),
 .UNSPECIFIED. ) ;
#5156=ORIENTED_EDGE ( 'NONE', *, *, #27593, .T. ) ;
#5159=CARTESIAN_POINT ( 'NONE',  ( 50.93312545610842790, 0.6352506689595297518, -1.438808137080895611 ) ) ;
#5161=EDGE_CURVE ( 'NONE', #14419, #21148, #10855, .T. ) ;
#5164=AXIS2_PLACEMENT_3D ( 'NONE', #11989, #2639, #19432 ) ;
#5170=( BOUNDED_SURFACE ( )  B_SPLINE_SURFACE ( 3, 2, ( 
 ( #27659, #27493, #15924 ),
 ( #13552, #18010, #17856 ),
 ( #27823, #1667, #25585 ),
 ( #30185, #23074, #5987 ),
 ( #23384, #1370, #23235 ),
 ( #1523, #11326, #20398 ) ),
 .UNSPECIFIED., .F., .F., .T. ) 
 B_SPLINE_SURFACE_WITH_KNOTS ( ( 4, 2, 4 ),
 ( 3, 3 ),
 ( 9.486769009248163798E-19, 0.0002090583013612445288, 0.0004181166027224881361 ),
 ( 0.000000000000000000, 1.000000000000000000 ),
 .UNSPECIFIED. ) 
 GEOMETRIC_REPRESENTATION_ITEM ( )  RATIONAL_B_SPLINE_SURFACE ( (
 ( 1.000000000000000000, 0.7071067811865492381, 1.000000000000000000),
 ( 1.000000000000000000, 0.7521684882082728674, 1.000000000000000000),
 ( 1.000000000000000000, 0.7851308282770136371, 1.000000000000000000),
 ( 1.000000000000000000, 0.8276934144745947686, 1.000000000000000000),
 ( 1.000000000000000000, 0.8364441017664203670, 1.000000000000000000),
 ( 1.000000000000000000, 0.8366600265340731202, 1.000000000000000000) ) ) 
 REPRESENTATION_ITEM ( '' )  SURFACE ( )  );
#5184=DIRECTION ( 'NONE',  ( 1.000000000000000000, 1.047444401652940007E-14, 0.000000000000000000 ) ) ;
#5188=DIRECTION ( 'NONE',  ( 0.000000000000000000, 0.4531102586345838179, -0.8914544820236760536 ) ) ;
#5192=CARTESIAN_POINT ( 'NONE',  ( 52.06628335902946247, -0.5434431642975682264, -1.794517909405659806 ) ) ;
#5198=CARTESIAN_POINT ( 'NONE',  ( 52.20711756518984714, -0.7499999999994533262, -1.996089927833914146 ) ) ;
#5199=CIRCLE ( 'NONE', #3681, 0.1500000000000001887 ) ;
#5205=EDGE_CURVE ( 'NONE', #25278, #10205, #22491, .T. ) ;
#5209=EDGE_CURVE ( 'NONE', #2740, #27829, #2608, .T. ) ;
#5211=CARTESIAN_POINT ( 'NONE',  ( 58.75000006180458456, 0.5511536957114213653, 1.849318015439010532 ) ) ;
#5213=ORIENTED_EDGE ( 'NONE', *, *, #771, .F. ) ;
#5214=CARTESIAN_POINT ( 'NONE',  ( 58.65266784251144827, -1.827264058874260133, 0.4207260278637539597 ) ) ;
#5219=DIRECTION ( 'NONE',  ( -2.167639087557276846E-15, 0.2069455031824688485, -0.9783524716136586807 ) ) ;
#5221=AXIS2_PLACEMENT_3D ( 'NONE', #13155, #8254, #1273 ) ;
#5222=ORIENTED_EDGE ( 'NONE', *, *, #29707, .F. ) ;
#5223=ORIENTED_EDGE ( 'NONE', *, *, #20813, .F. ) ;
#5225=DIRECTION ( 'NONE',  ( 1.093889549751081128E-14, -0.9507508458637282667, -0.3099561728525587756 ) ) ;
#5239=CIRCLE ( 'NONE', #8209, 1.487500000000000933 ) ;
#5246=DIRECTION ( 'NONE',  ( 0.000000000000000000, 0.000000000000000000, 1.000000000000000000 ) ) ;
#5247=DIRECTION ( 'NONE',  ( 0.000000000000000000, 0.000000000000000000, 1.000000000000000000 ) ) ;
#5248=DIRECTION ( 'NONE',  ( 0.000000000000000000, 0.000000000000000000, 1.000000000000000000 ) ) ;
#5254=DIRECTION ( 'NONE',  ( 0.8023336663629093701, 0.5470456816110859100, -0.2387503090077881251 ) ) ;
#5258=VERTEX_POINT ( 'NONE', #22339 ) ;
#5259=CIRCLE ( 'NONE', #22970, 0.1000000000000000611 ) ;
#5260=CARTESIAN_POINT ( 'NONE',  ( 51.31572262954149011, 1.002608958138273554, -1.395204572094392637 ) ) ;
#5263=CARTESIAN_POINT ( 'NONE',  ( 58.65000000000002700, -0.5539202450379242526, -1.791540873397694966 ) ) ;
#5264=B_SPLINE_CURVE_WITH_KNOTS ( 'NONE', 3,
 ( #26635, #1765, #9069, #18743, #6689, #28535 ),
 .UNSPECIFIED., .F., .F.,
 ( 4, 2, 4 ),
 ( 0.000000000000000000, 0.0003982002662752217367, 0.0007964005325504434733 ),
 .UNSPECIFIED. ) ;
#5268=ORIENTED_EDGE ( 'NONE', *, *, #3523, .T. ) ;
#5271=AXIS2_PLACEMENT_3D ( 'NONE', #7854, #15146, #20076 ) ;
#5276=CARTESIAN_POINT ( 'NONE',  ( 58.75000000000002842, -1.077297519403688009, -1.655311165516759608 ) ) ;
#5281=DIRECTION ( 'NONE',  ( 0.000000000000000000, 0.000000000000000000, 1.000000000000000000 ) ) ;
#5285=AXIS2_PLACEMENT_3D ( 'NONE', #20934, #6355, #18564 ) ;
#5287=ORIENTED_EDGE ( 'NONE', *, *, #11983, .T. ) ;
#5288=ADVANCED_FACE ( 'NONE', ( #26914 ), #627, .T. ) ;
#5292=CARTESIAN_POINT ( 'NONE',  ( 60.75000000000003553, -0.9999999999993638422, -1.996089927833914146 ) ) ;
#5293=DIRECTION ( 'NONE',  ( 0.000000000000000000, 0.000000000000000000, 1.000000000000000000 ) ) ;
#5309=ADVANCED_FACE ( 'NONE', ( #22030 ), #2475, .T. ) ;
#5311=FACE_OUTER_BOUND ( 'NONE', #23467, .T. ) ;
#5312=EDGE_CURVE ( 'NONE', #1336, #2824, #993, .T. ) ;
#5316=CARTESIAN_POINT ( 'NONE',  ( 51.34893360928146677, -1.002183861492330630, 1.396106892655424980 ) ) ;
#5319=CARTESIAN_POINT ( 'NONE',  ( 61.09423418604154676, -0.6373668173473425735, 1.895722432253304168 ) ) ;
#5321=TOROIDAL_SURFACE ( 'NONE', #9391, 1.875000000000000222, 0.2500000000000000000 ) ;
#5324=CARTESIAN_POINT ( 'NONE',  ( 58.64999999999992752, -1.877732920580853948, 0.6121634413819996290 ) ) ;
#5337=ORIENTED_EDGE ( 'NONE', *, *, #3505, .T. ) ;
#5350=CIRCLE ( 'NONE', #15460, 0.2500000000000000000 ) ;
#5353=( BOUNDED_CURVE ( )  B_SPLINE_CURVE ( 3, ( #23769, #8699, #28502, #16467 ),
 .UNSPECIFIED., .F., .T. ) 
 B_SPLINE_CURVE_WITH_KNOTS ( ( 4, 4 ),
 ( 1.982313172862383732, 2.241731514487931065 ),
 .UNSPECIFIED. ) 
 CURVE ( )  GEOMETRIC_REPRESENTATION_ITEM ( )  RATIONAL_B_SPLINE_CURVE ( ( 1.000000000000000000, 0.9943997021150919879, 0.9943997021150919879, 1.000000000000000000 ) ) 
 REPRESENTATION_ITEM ( '' )  );
#5359=CARTESIAN_POINT ( 'NONE',  ( 58.65000000000003411, -1.320082690053553387, -1.469015551796290397 ) ) ;
#5360=AXIS2_PLACEMENT_3D ( 'NONE', #28470, #3763, #6772 ) ;
#5361=DIRECTION ( 'NONE',  ( 1.000000000000000000, 1.047444401652940007E-14, 0.000000000000000000 ) ) ;
#5380=AXIS2_PLACEMENT_3D ( 'NONE', #27947, #23054, #8773 ) ;
#5383=EDGE_LOOP ( 'NONE', ( #25715, #24167, #6740, #26466 ) ) ;
#5389=EDGE_LOOP ( 'NONE', ( #9825, #30740, #7516, #9625, #22269 ) ) ;
#5391=CARTESIAN_POINT ( 'NONE',  ( 58.75000000000003553, -1.320165430233233295, -1.457266603153496876 ) ) ;
#5393=EDGE_CURVE ( 'NONE', #28012, #6477, #3634, .T. ) ;
#5395=AXIS2_PLACEMENT_3D ( 'NONE', #14719, #19794, #17404 ) ;
#5396=ORIENTED_EDGE ( 'NONE', *, *, #23794, .T. ) ;
#5408=CARTESIAN_POINT ( 'NONE',  ( 51.14630318392407560, -0.9364487020629673752, -1.503522130792586564 ) ) ;
#5423=CARTESIAN_POINT ( 'NONE',  ( 60.88479802533564111, -0.4999999999993592348, 1.718465885608769117 ) ) ;
#5447=CARTESIAN_POINT ( 'NONE',  ( 51.98914612709257455, 0.7788013043310292316, -1.433123603079363484 ) ) ;
#5449=DIRECTION ( 'NONE',  ( 1.000000000000000000, 1.047444401652940007E-14, 0.000000000000000000 ) ) ;
#5450=CIRCLE ( 'NONE', #7464, 0.09999999999999979738 ) ;
#5451=DIRECTION ( 'NONE',  ( 1.000000000000000000, 1.047444401652940007E-14, 0.000000000000000000 ) ) ;
#5455=AXIS2_PLACEMENT_3D ( 'NONE', #25705, #30928, #17849 ) ;
#5457=DIRECTION ( 'NONE',  ( 1.000000000000000000, 1.047444401652940007E-14, 0.000000000000000000 ) ) ;
#5464=ORIENTED_EDGE ( 'NONE', *, *, #23542, .F. ) ;
#5474=ORIENTED_EDGE ( 'NONE', *, *, #25732, .F. ) ;
#5475=ADVANCED_FACE ( 'NONE', ( #17893 ), #27529, .T. ) ;
#5476=CARTESIAN_POINT ( 'NONE',  ( 58.75000000000002132, 6.153735859711025284E-13, 3.111507638930570854E-58 ) ) ;
#5477=ORIENTED_EDGE ( 'NONE', *, *, #30308, .F. ) ;
#5487=CYLINDRICAL_SURFACE ( 'NONE', #14977, 0.5000000000000000000 ) ;
#5489=CIRCLE ( 'NONE', #12554, 0.1499999999999999667 ) ;
#5492=CARTESIAN_POINT ( 'NONE',  ( 51.08379317338048509, -0.8723108729827115937, 1.374656996893404148 ) ) ;
#5503=CARTESIAN_POINT ( 'NONE',  ( 58.66133336607590820, 0.9657121834149602346, 1.607522887372458076 ) ) ;
#5505=ORIENTED_EDGE ( 'NONE', *, *, #3362, .F. ) ;
#5511=DIRECTION ( 'NONE',  ( 0.000000000000000000, 0.000000000000000000, 1.000000000000000000 ) ) ;
#5515=CARTESIAN_POINT ( 'NONE',  ( 58.72200624034153549, 1.634766674885311133, -0.9185080301418440119 ) ) ;
#5524=EDGE_CURVE ( 'NONE', #29235, #10512, #19723, .T. ) ;
#5526=CIRCLE ( 'NONE', #24249, 0.1500000000000001887 ) ;
#5532=DIRECTION ( 'NONE',  ( 0.000000000000000000, 0.9985773570673159849, -0.05332224631853133001 ) ) ;
#5540=CARTESIAN_POINT ( 'NONE',  ( 60.75000000000002842, -0.7499999999993639532, -1.718465885608440269 ) ) ;
#5544=CARTESIAN_POINT ( 'NONE',  ( 51.17957687186121518, -0.9671124184258252932, 1.523623459118159440 ) ) ;
#5547=DIRECTION ( 'NONE',  ( 0.000000000000000000, 0.000000000000000000, 1.000000000000000000 ) ) ;
#5554=CARTESIAN_POINT ( 'NONE',  ( 58.75000000000002132, 6.153735859711025284E-13, 3.111507638930570854E-58 ) ) ;
#5556=CARTESIAN_POINT ( 'NONE',  ( 58.75000000694009827, -1.346330794793457519, -1.381609951798280500 ) ) ;
#5568=DIRECTION ( 'NONE',  ( 0.000000000000000000, 0.000000000000000000, 1.000000000000000000 ) ) ;
#5570=DIRECTION ( 'NONE',  ( 0.000000000000000000, -0.5454670984325209471, -0.8381322357048476279 ) ) ;
#5572=CYLINDRICAL_SURFACE ( 'NONE', #24612, 0.1500000000000001887 ) ;
#5579=EDGE_CURVE ( 'NONE', #4338, #29960, #23424, .T. ) ;
#5584=ORIENTED_EDGE ( 'NONE', *, *, #23141, .F. ) ;
#5594=VERTEX_POINT ( 'NONE', #23895 ) ;
#5595=( NAMED_UNIT ( * ) PLANE_ANGLE_UNIT ( ) SI_UNIT ( $, .RADIAN. ) );
#5599=EDGE_LOOP ( 'NONE', ( #21634, #20050, #23505, #9460 ) ) ;
#5604=CARTESIAN_POINT ( 'NONE',  ( 52.10126625705171222, 0.5195911883743921100, -1.546252172343136611 ) ) ;
#5605=CARTESIAN_POINT ( 'NONE',  ( 60.75000000000001421, 0.6500000000006364020, 1.489337100860647967 ) ) ;
#5606=DIRECTION ( 'NONE',  ( 1.000000000000000000, 1.047444401652940007E-14, 0.000000000000000000 ) ) ;
#5608=CARTESIAN_POINT ( 'NONE',  ( 51.27853981583098886, 1.002608958138269113, 1.395204572094398854 ) ) ;
#5609=CARTESIAN_POINT ( 'NONE',  ( 58.75000000000001421, 0.5380862305915415922, -2.008165151417984351 ) ) ;
#5610=FACE_OUTER_BOUND ( 'NONE', #21742, .T. ) ;
#5617=EDGE_CURVE ( 'NONE', #7928, #31291, #9967, .T. ) ;
#5621=ORIENTED_EDGE ( 'NONE', *, *, #21170, .F. ) ;
#5624=DIRECTION ( 'NONE',  ( 1.387778780781445676E-14, -1.000000000000000000, 0.000000000000000000 ) ) ;
#5627=EDGE_LOOP ( 'NONE', ( #14550, #13842, #4792, #28700 ) ) ;
#5630=CARTESIAN_POINT ( 'NONE',  ( 51.43355796162960303, 0.9748468443439985975, -1.443681521171340520 ) ) ;
#5645=CIRCLE ( 'NONE', #29914, 0.2500000000000000000 ) ;
#5653=EDGE_LOOP ( 'NONE', ( #30909, #22533, #28717, #3942 ) ) ;
#5654=CARTESIAN_POINT ( 'NONE',  ( 52.20711756518984714, -0.6499999999994533484, 1.489337100860647967 ) ) ;
#5657=DIRECTION ( 'NONE',  ( 1.000000000000000000, 1.047444401652940007E-14, 0.000000000000000000 ) ) ;
#5663=ORIENTED_EDGE ( 'NONE', *, *, #15418, .F. ) ;
#5669=CARTESIAN_POINT ( 'NONE',  ( 58.65000038048046349, 1.580579251836441435, -1.008797009996411642 ) ) ;
#5685=EDGE_LOOP ( 'NONE', ( #25079, #457, #23739, #268 ) ) ;
#5687=ORIENTED_EDGE ( 'NONE', *, *, #21865, .F. ) ;
#5691=CARTESIAN_POINT ( 'NONE',  ( 58.65000000000003411, -1.253243060178391932, 1.394635017527226628 ) ) ;
#5692=ORIENTED_EDGE ( 'NONE', *, *, #9215, .T. ) ;
#5693=ORIENTED_EDGE ( 'NONE', *, *, #17110, .F. ) ;
#5697=EDGE_LOOP ( 'NONE', ( #17193, #25746, #19664, #3732 ) ) ;
#5700=( BOUNDED_CURVE ( )  B_SPLINE_CURVE ( 3, ( #24137, #28884, #7343, #14306 ),
 .UNSPECIFIED., .F., .T. ) 
 B_SPLINE_CURVE_WITH_KNOTS ( ( 4, 4 ),
 ( 1.454199501120267524, 2.189070931013918031 ),
 .UNSPECIFIED. ) 
 CURVE ( )  GEOMETRIC_REPRESENTATION_ITEM ( )  RATIONAL_B_SPLINE_CURVE ( ( 1.000000000000000000, 0.9555010429016485007, 0.9555010429016485007, 1.000000000000000000 ) ) 
 REPRESENTATION_ITEM ( '' )  );
#5702=CIRCLE ( 'NONE', #21407, 2.000000000000000000 ) ;
#5707=ORIENTED_EDGE ( 'NONE', *, *, #21609, .T. ) ;
#5723=EDGE_LOOP ( 'NONE', ( #17170, #9498, #24346, #6791 ) ) ;
#5729=ORIENTED_EDGE ( 'NONE', *, *, #2818, .T. ) ;
#5730=CARTESIAN_POINT ( 'NONE',  ( 61.01502350126983742, -0.5557829358550897547, 1.706838207573794453 ) ) ;
#5737=VERTEX_POINT ( 'NONE', #29408 ) ;
#5740=ORIENTED_EDGE ( 'NONE', *, *, #22553, .F. ) ;
#5741=( LENGTH_UNIT ( ) NAMED_UNIT ( * ) SI_UNIT ( .MILLI., .METRE. ) );
#5742=CARTESIAN_POINT ( 'NONE',  ( 51.37201957452462153, 0.9974676312069150619, -1.404527551348820680 ) ) ;
#5753=DIRECTION ( 'NONE',  ( 0.000000000000000000, 0.000000000000000000, 1.000000000000000000 ) ) ;
#5763=DIRECTION ( 'NONE',  ( 1.000000000000000000, 1.047444401652940007E-14, 0.000000000000000000 ) ) ;
#5764=CARTESIAN_POINT ( 'NONE',  ( 58.74154451056411830, 1.390058629629814968, -1.258335925859399351 ) ) ;
#5767=ORIENTED_EDGE ( 'NONE', *, *, #30368, .F. ) ;
#5770=ORIENTED_EDGE ( 'NONE', *, *, #3647, .T. ) ;
#5779=VERTEX_POINT ( 'NONE', #2809 ) ;
#5782=DIRECTION ( 'NONE',  ( 0.000000000000000000, 0.000000000000000000, 1.000000000000000000 ) ) ;
#5788=EDGE_CURVE ( 'NONE', #24125, #16052, #26328, .T. ) ;
#5800=DIRECTION ( 'NONE',  ( 0.5633368246415176861, -0.8262273428075422865, 0.000000000000000000 ) ) ;
#5801=CARTESIAN_POINT ( 'NONE',  ( 51.17290532404553716, -0.9646187004837835088, 1.462925393634369353 ) ) ;
#5802=ORIENTED_EDGE ( 'NONE', *, *, #29021, .T. ) ;
#5804=VECTOR ( 'NONE', #26833, 1000.000000000000000 ) ;
#5805=CARTESIAN_POINT ( 'NONE',  ( 51.36283714269054457, -1.001673184507024805, -1.284520656909109659 ) ) ;
#5807=ORIENTED_EDGE ( 'NONE', *, *, #29744, .T. ) ;
#5808=FACE_OUTER_BOUND ( 'NONE', #5697, .T. ) ;
#5810=CARTESIAN_POINT ( 'NONE',  ( 51.59739104186229497, -1.010292945602101256, 1.272765950230260623 ) ) ;
#5811=VECTOR ( 'NONE', #18645, 1000.000000000000000 ) ;
#5815=EDGE_LOOP ( 'NONE', ( #28935, #24975, #22465, #19658 ) ) ;
#5820=FACE_OUTER_BOUND ( 'NONE', #1144, .T. ) ;
#5825=DIRECTION ( 'NONE',  ( 0.000000000000000000, 8.881784197001054122E-16, 1.000000000000000000 ) ) ;
#5827=CARTESIAN_POINT ( 'NONE',  ( 58.74999999305995146, 1.657788420845899724, -0.9867593359914171858 ) ) ;
#5833=AXIS2_PLACEMENT_3D ( 'NONE', #25351, #25023, #15703 ) ;
#5836=AXIS2_PLACEMENT_3D ( 'NONE', #30795, #9106, #18774 ) ;
#5841=CARTESIAN_POINT ( 'NONE',  ( 58.74999981196287280, -1.953821646384657384, -0.08499607038929953007 ) ) ;
#5850=ORIENTED_EDGE ( 'NONE', *, *, #15111, .T. ) ;
#5856=ORIENTED_EDGE ( 'NONE', *, *, #26317, .F. ) ;
#5860=AXIS2_PLACEMENT_3D ( 'NONE', #22291, #575, #12603 ) ;
#5861=CARTESIAN_POINT ( 'NONE',  ( 60.94140446608462014, 0.5380862305989584371, -1.858165151370887669 ) ) ;
#5881=DIRECTION ( 'NONE',  ( 0.000000000000000000, 0.000000000000000000, 1.000000000000000000 ) ) ;
#5888=AXIS2_PLACEMENT_3D ( 'NONE', #9402, #6703, #14297 ) ;
#5898=APPLICATION_CONTEXT ( 'automotive_design' ) ;
#5907=CARTESIAN_POINT ( 'NONE',  ( 51.45655683570189609, 0.9591657938401617622, -1.468576096419531352 ) ) ;
#5913=AXIS2_PLACEMENT_3D ( 'NONE', #25193, #10775, #20457 ) ;
#5919=CARTESIAN_POINT ( 'NONE',  ( 58.75000000000001421, 0.5933363752225945253, -1.867039175319659572 ) ) ;
#5923=EDGE_CURVE ( 'NONE', #15962, #2931, #12492, .T. ) ;
#5926=AXIS2_PLACEMENT_3D ( 'NONE', #2150, #28911, #28598 ) ;
#5928=CARTESIAN_POINT ( 'NONE',  ( 58.75000000000000000, 2.008165151418861427, -0.5380862305899540843 ) ) ;
#5930=CARTESIAN_POINT ( 'NONE',  ( 58.65000045311410304, 1.383426348888211699, -1.265716300431776631 ) ) ;
#5936=CYLINDRICAL_SURFACE ( 'NONE', #12921, 1.625000000000000222 ) ;
#5946=VERTEX_POINT ( 'NONE', #25437 ) ;
#5949=ORIENTED_EDGE ( 'NONE', *, *, #12259, .T. ) ;
#5956=DIRECTION ( 'NONE',  ( 1.000000000000000000, 1.047444401652940007E-14, 0.000000000000000000 ) ) ;
#5965=CARTESIAN_POINT ( 'NONE',  ( 58.73371041428917039, 1.267950628961455939, 1.381461519774026536 ) ) ;
#5966=AXIS2_PLACEMENT_3D ( 'NONE', #21961, #249, #9913 ) ;
#5968=DIRECTION ( 'NONE',  ( 1.387778780781445676E-14, -1.000000000000000000, 0.000000000000000000 ) ) ;
#5970=FACE_OUTER_BOUND ( 'NONE', #26813, .T. ) ;
#5972=DIRECTION ( 'NONE',  ( 1.000000000000000000, 1.047444401652940007E-14, -0.000000000000000000 ) ) ;
#5974=ORIENTED_EDGE ( 'NONE', *, *, #21270, .T. ) ;
#5984=EDGE_CURVE ( 'NONE', #585, #779, #15314, .T. ) ;
#5987=CARTESIAN_POINT ( 'NONE',  ( 61.02708519082507621, -0.5631634571404888767, 1.705199831323249038 ) ) ;
#5988=CARTESIAN_POINT ( 'NONE',  ( 51.31572262954149721, 1.002608958138273554, 1.395204572094392192 ) ) ;
#5998=EDGE_CURVE ( 'NONE', #4089, #24848, #2410, .T. ) ;
#5999=CARTESIAN_POINT ( 'NONE',  ( 58.75000000000000711, 1.760622601996782777, 0.8948927608044729975 ) ) ;
#6000=DIRECTION ( 'NONE',  ( 1.000000000000000000, 1.047444401652940007E-14, 0.000000000000000000 ) ) ;
#6002=AXIS2_PLACEMENT_3D ( 'NONE', #620, #10280, #29294 ) ;
#6003=ORIENTED_EDGE ( 'NONE', *, *, #16141, .F. ) ;
#6010=B_SPLINE_CURVE_WITH_KNOTS ( 'NONE', 3,
 ( #21688, #12876, #29672, #695 ),
 .UNSPECIFIED., .F., .F.,
 ( 4, 4 ),
 ( 0.000000000000000000, 0.0001494103359351912257 ),
 .UNSPECIFIED. ) ;
#6011=CARTESIAN_POINT ( 'NONE',  ( 58.65000038048068376, -1.873220289782048686, 0.08335421200007571418 ) ) ;
#6013=EDGE_CURVE ( 'NONE', #704, #10186, #11819, .T. ) ;
#6020=FACE_OUTER_BOUND ( 'NONE', #11820, .T. ) ;
#6026=CIRCLE ( 'NONE', #13584, 1.975000000000001865 ) ;
#6035=VECTOR ( 'NONE', #4348, 1000.000000000000000 ) ;
#6045=CARTESIAN_POINT ( 'NONE',  ( 58.64999999999992042, -1.077297519403624060, -1.655311165517087568 ) ) ;
#6046=DIRECTION ( 'NONE',  ( 0.000000000000000000, 0.000000000000000000, 1.000000000000000000 ) ) ;
#6050=EDGE_CURVE ( 'NONE', #23458, #10001, #30701, .T. ) ;
#6051=ORIENTED_EDGE ( 'NONE', *, *, #11746, .F. ) ;
#6060=AXIS2_PLACEMENT_3D ( 'NONE', #21305, #14299, #5547 ) ;
#6061=ORIENTED_EDGE ( 'NONE', *, *, #2115, .T. ) ;
#6068=AXIS2_PLACEMENT_3D ( 'NONE', #3482, #18055, #25321 ) ;
#6076=CARTESIAN_POINT ( 'NONE',  ( 60.89136863770590224, 0.5000000000006363798, 1.718465794862841678 ) ) ;
#6077=CARTESIAN_POINT ( 'NONE',  ( 58.65000000000003411, -1.655311165516606398, -1.077297519404007309 ) ) ;
#6080=DIRECTION ( 'NONE',  ( 1.000000000000000000, 1.047444401652940007E-14, 0.000000000000000000 ) ) ;
#6085=CARTESIAN_POINT ( 'NONE',  ( 58.66122797211835405, -1.615588400946606162, -0.9517229765811223707 ) ) ;
#6094=CARTESIAN_POINT ( 'NONE',  ( 58.75000000000002132, 6.153735859711025284E-13, 3.111507638930570854E-58 ) ) ;
#6099=VERTEX_POINT ( 'NONE', #26066 ) ;
#6101=ORIENTED_EDGE ( 'NONE', *, *, #15418, .T. ) ;
#6102=DIRECTION ( 'NONE',  ( 6.600692696441737066E-15, -0.6683962987610915230, -0.7438053426821252812 ) ) ;
#6114=CARTESIAN_POINT ( 'NONE',  ( 58.72204580543407815, 1.341784641882211693, 1.309860786662967680 ) ) ;
#6117=CARTESIAN_POINT ( 'NONE',  ( 58.75000000000000711, 1.039502773797213120, -1.650471618823823539 ) ) ;
#6127=VERTEX_POINT ( 'NONE', #26231 ) ;
#6128=DIRECTION ( 'NONE',  ( 0.000000000000000000, 0.000000000000000000, 1.000000000000000000 ) ) ;
#6132=CARTESIAN_POINT ( 'NONE',  ( 51.25000000000001421, 1.100000000000537215, 1.196087371390568643 ) ) ;
#6136=DIRECTION ( 'NONE',  ( 0.000000000000000000, 0.000000000000000000, 1.000000000000000000 ) ) ;
#6144=FACE_OUTER_BOUND ( 'NONE', #555, .T. ) ;
#6146=DIRECTION ( 'NONE',  ( 0.000000000000000000, -8.881784197000848032E-16, 1.000000000000000000 ) ) ;
#6147=CARTESIAN_POINT ( 'NONE',  ( 52.20711756518984714, -0.6499999999994510169, 1.489337100860649077 ) ) ;
#6155=FACE_OUTER_BOUND ( 'NONE', #6528, .T. ) ;
#6157=EDGE_CURVE ( 'NONE', #15867, #10721, #30490, .T. ) ;
#6163=AXIS2_PLACEMENT_3D ( 'NONE', #27290, #5606, #1609 ) ;
#6167=CARTESIAN_POINT ( 'NONE',  ( 58.75000000000000711, 0.8979909453699834732, -1.749377236609715780 ) ) ;
#6187=DIRECTION ( 'NONE',  ( 1.047444401652940007E-14, -1.000000000000000000, 0.000000000000000000 ) ) ;
#6195=DIRECTION ( 'NONE',  ( 1.000000000000000000, 1.047444401652940007E-14, 0.000000000000000000 ) ) ;
#6206=ORIENTED_EDGE ( 'NONE', *, *, #2618, .T. ) ;
#6207=CARTESIAN_POINT ( 'NONE',  ( 58.75000000000000711, 0.8948927608039202175, -1.760622601996761460 ) ) ;
#6209=VERTEX_POINT ( 'NONE', #24626 ) ;
#6215=ADVANCED_FACE ( 'NONE', ( #19745 ), #21493, .T. ) ;
#6220=CARTESIAN_POINT ( 'NONE',  ( 61.25000000000004263, -1.800471618824687869, 1.039502773796719959 ) ) ;
#6221=DIRECTION ( 'NONE',  ( 1.000000000000000000, 1.047444401652940007E-14, -0.000000000000000000 ) ) ;
#6222=CONICAL_SURFACE ( 'NONE', #27953, 1.875000000000001776, 0.7853981633974510546 ) ;
#6230=EDGE_CURVE ( 'NONE', #6099, #7928, #29376, .T. ) ;
#6231=CARTESIAN_POINT ( 'NONE',  ( 58.75000018595672913, -1.701752411746506821, -0.9248597378502191324 ) ) ;
#6235=CYLINDRICAL_SURFACE ( 'NONE', #25222, 2.000000000000000000 ) ;
#6247=LINE ( 'NONE', #28251, #30070 ) ;
#6253=DIRECTION ( 'NONE',  ( 0.000000000000000000, 0.000000000000000000, 1.000000000000000000 ) ) ;
#6254=ORIENTED_EDGE ( 'NONE', *, *, #1875, .F. ) ;
#6258=CARTESIAN_POINT ( 'NONE',  ( 51.14630318392396902, -0.9364487020628400327, 1.503522130792752209 ) ) ;
#6263=DIRECTION ( 'NONE',  ( 1.000000000000000000, 1.047444401652940007E-14, 0.000000000000000000 ) ) ;
#6269=CARTESIAN_POINT ( 'NONE',  ( 61.25000000000004263, -1.960427193527463086, 0.3958853607744572956 ) ) ;
#6274=VERTEX_POINT ( 'NONE', #7229 ) ;
#6281=CARTESIAN_POINT ( 'NONE',  ( 52.13000000000003098, -0.4999999999994542144, 1.718465885608440491 ) ) ;
#6287=CIRCLE ( 'NONE', #24473, 0.1000000000000001027 ) ;
#6289=CARTESIAN_POINT ( 'NONE',  ( 58.74160516400052501, 1.784764912520735214, -0.5747049900151632862 ) ) ;
#6291=DIRECTION ( 'NONE',  ( 0.000000000000000000, 0.000000000000000000, 1.000000000000000000 ) ) ;
#6296=CARTESIAN_POINT ( 'NONE',  ( 58.75000000000002842, -1.039502773796102897, -1.800471618824325493 ) ) ;
#6309=DIRECTION ( 'NONE',  ( 1.000000000000000000, 1.047444401652940007E-14, 0.000000000000000000 ) ) ;
#6311=FACE_OUTER_BOUND ( 'NONE', #10214, .T. ) ;
#6312=EDGE_CURVE ( 'NONE', #9733, #10218, #15567, .T. ) ;
#6313=ORIENTED_EDGE ( 'NONE', *, *, #19533, .F. ) ;
#6317=DIRECTION ( 'NONE',  ( 1.000000000000000000, 1.047444401652940007E-14, 0.000000000000000000 ) ) ;
#6324=EDGE_CURVE ( 'NONE', #7871, #27840, #26185, .T. ) ;
#6328=ORIENTED_EDGE ( 'NONE', *, *, #19699, .T. ) ;
#6331=CARTESIAN_POINT ( 'NONE',  ( 61.25000000000001421, 0.9840188032656856931, -1.660129320691967614 ) ) ;
#6333=CARTESIAN_POINT ( 'NONE',  ( 58.75000000000000711, 1.791164585742715198, 0.8897917884450912140 ) ) ;
#6337=AXIS2_PLACEMENT_3D ( 'NONE', #30395, #15539, #18239 ) ;
#6343=CARTESIAN_POINT ( 'NONE',  ( 60.75000000000002842, -0.4999999999993638977, -1.718465885608440047 ) ) ;
#6345=CARTESIAN_POINT ( 'NONE',  ( 58.75000000000000000, 1.834410884276219234, 0.3880228184671279945 ) ) ;
#6355=DIRECTION ( 'NONE',  ( 1.000000000000000000, 1.047444401652940007E-14, 0.000000000000000000 ) ) ;
#6367=VERTEX_POINT ( 'NONE', #15433 ) ;
#6372=AXIS2_PLACEMENT_3D ( 'NONE', #4069, #8799, #11338 ) ;
#6374=CIRCLE ( 'NONE', #18501, 0.1500000000000001887 ) ;
#6376=AXIS2_PLACEMENT_3D ( 'NONE', #19403, #21942, #26968 ) ;
#6401=EDGE_LOOP ( 'NONE', ( #21385, #1269, #7225, #17277 ) ) ;
#6406=DIRECTION ( 'NONE',  ( 0.000000000000000000, -7.105427357601001859E-15, 1.000000000000000000 ) ) ;
#6415=ADVANCED_FACE ( 'NONE', ( #8306 ), #17440, .T. ) ;
#6417=CARTESIAN_POINT ( 'NONE',  ( 51.59739104186229497, -1.010292945602100367, -1.272765950230261067 ) ) ;
#6418=CARTESIAN_POINT ( 'NONE',  ( 51.41321594800584194, -0.9846907464474132787, 1.426729742943413148 ) ) ;
#6425=CARTESIAN_POINT ( 'NONE',  ( 61.25000000000002132, 6.415596960124259844E-13, 3.111507638930570854E-58 ) ) ;
#6428=CIRCLE ( 'NONE', #1786, 2.000000000000000000 ) ;
#6431=FACE_OUTER_BOUND ( 'NONE', #29309, .T. ) ;
#6433=AXIS2_PLACEMENT_3D ( 'NONE', #25572, #1358, #15455 ) ;
#6438=EDGE_CURVE ( 'NONE', #29220, #11262, #18709, .T. ) ;
#6439=CYLINDRICAL_SURFACE ( 'NONE', #18911, 2.000000000000000000 ) ;
#6452=CARTESIAN_POINT ( 'NONE',  ( 50.25000000000002842, -1.039502773797060131, 1.800471618824829756 ) ) ;
#6455=ORIENTED_EDGE ( 'NONE', *, *, #22698, .T. ) ;
#6457=CARTESIAN_POINT ( 'NONE',  ( 58.72204580543391472, 1.805265037612412860, -0.5070891929463556824 ) ) ;
#6462=AXIS2_PLACEMENT_3D ( 'NONE', #24159, #28901, #4195 ) ;
#6463=VECTOR ( 'NONE', #29007, 1000.000000000000000 ) ;
#6475=ADVANCED_FACE ( 'NONE', ( #15892 ), #2276, .F. ) ;
#6477=VERTEX_POINT ( 'NONE', #18446 ) ;
#6482=CARTESIAN_POINT ( 'NONE',  ( 51.25000000000002842, -1.099999999999459410, -1.001327244211406953 ) ) ;
#6489=ADVANCED_FACE ( 'NONE', ( #20824 ), #16542, .F. ) ;
#6495=ORIENTED_EDGE ( 'NONE', *, *, #13708, .F. ) ;
#6496=CARTESIAN_POINT ( 'NONE',  ( 61.25000000000001421, 1.000000000000641709, -1.655766640117574795 ) ) ;
#6510=DIRECTION ( 'NONE',  ( 0.7071067811865455743, 7.406550393246774337E-15, 0.7071067811865493491 ) ) ;
#6511=EDGE_CURVE ( 'NONE', #21983, #12582, #5700, .T. ) ;
#6514=CARTESIAN_POINT ( 'NONE',  ( 58.75000000000004263, -2.008165151418633165, 0.5380862305909606125 ) ) ;
#6515=CARTESIAN_POINT ( 'NONE',  ( 51.29335235176148444, 1.002608958138273554, -1.584424273060082378 ) ) ;
#6528=EDGE_LOOP ( 'NONE', ( #12930, #12887, #23737, #23974, #21927 ) ) ;
#6547=VECTOR ( 'NONE', #10908, 1000.000000000000000 ) ;
#6551=CARTESIAN_POINT ( 'NONE',  ( 51.13858604272873976, -1.070913481528389166, -1.222302725805714640 ) ) ;
#6552=DIRECTION ( 'NONE',  ( 1.000000000000000000, 1.047444401652940007E-14, 0.000000000000000000 ) ) ;
#6553=EDGE_CURVE ( 'NONE', #23458, #16137, #16707, .T. ) ;
#6559=VERTEX_POINT ( 'NONE', #2444 ) ;
#6560=ORIENTED_EDGE ( 'NONE', *, *, #3561, .T. ) ;
#6564=CARTESIAN_POINT ( 'NONE',  ( 58.65000000000004121, -1.671477153793470727, 0.8495817349404540808 ) ) ;
#6568=CARTESIAN_POINT ( 'NONE',  ( 58.65000000000003411, -1.874116925334127881, -0.06656272211242116044 ) ) ;
#6570=ORIENTED_EDGE ( 'NONE', *, *, #5788, .F. ) ;
#6576=CARTESIAN_POINT ( 'NONE',  ( 58.65000000000001279, 0.5811678240972328879, 1.782657835995121287 ) ) ;
#6581=LINE ( 'NONE', #25887, #6035 ) ;
#6584=CARTESIAN_POINT ( 'NONE',  ( 58.66122389686788807, -0.5174758696799709456, -1.802487374212213167 ) ) ;
#6585=CARTESIAN_POINT ( 'NONE',  ( 58.72427158855742135, -0.8981388483288218483, 1.646019958200248157 ) ) ;
#6590=LINE ( 'NONE', #3894, #26627 ) ;
#6591=ORIENTED_EDGE ( 'NONE', *, *, #25600, .F. ) ;
#6598=CARTESIAN_POINT ( 'NONE',  ( 52.20711756518984714, -0.6499999999994533484, 1.489337100860647967 ) ) ;
#6604=VERTEX_POINT ( 'NONE', #15244 ) ;
#6609=CARTESIAN_POINT ( 'NONE',  ( 58.74999999999999289, 1.834410884276637566, -0.3880228184651508538 ) ) ;
#6611=DIRECTION ( 'NONE',  ( 0.000000000000000000, 0.000000000000000000, 1.000000000000000000 ) ) ;
#6612=CARTESIAN_POINT ( 'NONE',  ( 50.25000000000002132, 5.263408118306026973E-13, 3.111507638930570854E-58 ) ) ;
#6622=ORIENTED_EDGE ( 'NONE', *, *, #22288, .T. ) ;
#6627=ORIENTED_EDGE ( 'NONE', *, *, #6438, .T. ) ;
#6629=ORIENTED_EDGE ( 'NONE', *, *, #8145, .T. ) ;
#6632=CARTESIAN_POINT ( 'NONE',  ( 58.75000000000004263, -2.008165151418373373, -0.5380862305909229759 ) ) ;
#6636=CARTESIAN_POINT ( 'NONE',  ( 50.25000000000002842, -1.039502773796191937, -1.650471618824325359 ) ) ;
#6644=CARTESIAN_POINT ( 'NONE',  ( 61.25000000000002132, 6.415596960124259844E-13, 3.111507638930570854E-58 ) ) ;
#6651=CARTESIAN_POINT ( 'NONE',  ( 58.65000000000003411, -1.589751505945435239, -0.9947034709617927906 ) ) ;
#6652=EDGE_CURVE ( 'NONE', #21568, #1882, #8175, .T. ) ;
#6656=CARTESIAN_POINT ( 'NONE',  ( 58.74154451056428883, -1.784780193103109092, -0.5746581230773456506 ) ) ;
#6661=VECTOR ( 'NONE', #4387, 1000.000000000000000 ) ;
#6662=CARTESIAN_POINT ( 'NONE',  ( 58.75000000000002132, 6.153735859711025284E-13, 3.111507638930570854E-58 ) ) ;
#6671=EDGE_LOOP ( 'NONE', ( #29685, #5707, #3053, #672 ) ) ;
#6672=CARTESIAN_POINT ( 'NONE',  ( 58.73868664959847052, 0.5000000000006151746, 1.844330893389497072 ) ) ;
#6686=CARTESIAN_POINT ( 'NONE',  ( 58.75000000000002132, 6.153735859711025284E-13, 3.111507638930570854E-58 ) ) ;
#6689=CARTESIAN_POINT ( 'NONE',  ( 61.25000000000002132, 0.8718791990819803051, 1.626461527140064423 ) ) ;
#6693=( NAMED_UNIT ( * ) SI_UNIT ( $, .STERADIAN. ) SOLID_ANGLE_UNIT ( ) );
#6703=DIRECTION ( 'NONE',  ( 1.000000000000000000, 1.047444401652940007E-14, 0.000000000000000000 ) ) ;
#6709=ORIENTED_EDGE ( 'NONE', *, *, #25661, .T. ) ;
#6712=CARTESIAN_POINT ( 'NONE',  ( 58.74999981404335614, -1.649595783783118774, 1.050697058759348934 ) ) ;
#6725=CARTESIAN_POINT ( 'NONE',  ( 51.45655683570191741, -0.9591657938390835136, 1.468576096419531574 ) ) ;
#6728=ADVANCED_FACE ( 'NONE', ( #18492 ), #17194, .T. ) ;
#6730=CARTESIAN_POINT ( 'NONE',  ( 58.64999999999999858, 1.760622601996781667, 0.8948927608044729975 ) ) ;
#6733=CARTESIAN_POINT ( 'NONE',  ( 58.75000018803720536, -1.010830333486641974, 1.651902078983862321 ) ) ;
#6740=ORIENTED_EDGE ( 'NONE', *, *, #20319, .F. ) ;
#6741=CARTESIAN_POINT ( 'NONE',  ( 51.13341687362841270, 0.9248174436456687575, 1.495576127288423818 ) ) ;
#6745=CYLINDRICAL_SURFACE ( 'NONE', #11487, 2.000000000000000000 ) ;
#6751=DIRECTION ( 'NONE',  ( 0.000000000000000000, 0.000000000000000000, 1.000000000000000000 ) ) ;
#6759=CARTESIAN_POINT ( 'NONE',  ( 58.75000000000000000, 1.922112613535394310, -0.4146634982021765170 ) ) ;
#6771=CYLINDRICAL_SURFACE ( 'NONE', #5913, 0.5000000000000000000 ) ;
#6772=DIRECTION ( 'NONE',  ( 0.000000000000000000, 0.000000000000000000, 1.000000000000000000 ) ) ;
#6777=ORIENTED_EDGE ( 'NONE', *, *, #28050, .F. ) ;
#6781=DIRECTION ( 'NONE',  ( 0.000000000000000000, 0.000000000000000000, 1.000000000000000000 ) ) ;
#6789=CARTESIAN_POINT ( 'NONE',  ( 58.66107449606931823, -1.349793924521457855, 1.301839550768250753 ) ) ;
#6791=ORIENTED_EDGE ( 'NONE', *, *, #21208, .F. ) ;
#6795=TOROIDAL_SURFACE ( 'NONE', #22464, 1.975000000000001865, 0.1000000000000000056 ) ;
#6802=DIRECTION ( 'NONE',  ( 1.000000000000000000, 1.047444401652940007E-14, 0.000000000000000000 ) ) ;
#6813=CARTESIAN_POINT ( 'NONE',  ( 51.84772254680353143, 0.6924618999072389425, 1.653428777428159746 ) ) ;
#6829=CARTESIAN_POINT ( 'NONE',  ( 58.75000000694004854, 1.928945400590568626, 0.02494613115323923019 ) ) ;
#6830=ORIENTED_EDGE ( 'NONE', *, *, #25732, .T. ) ;
#6843=PLANE ( 'NONE',  #9912 ) ;
#6844=TOROIDAL_SURFACE ( 'NONE', #760, 1.975000000000001865, 0.1000000000000000056 ) ;
#6851=AXIS2_PLACEMENT_3D ( 'NONE', #6889, #21325, #16388 ) ;
#6857=B_SPLINE_CURVE_WITH_KNOTS ( 'NONE', 3,
 ( #9067, #1301, #20799, #10971, #20654, #11123 ),
 .UNSPECIFIED., .F., .F.,
 ( 4, 2, 4 ),
 ( 0.000000000000000000, 0.0001000270069606238189, 0.0002000540139212476378 ),
 .UNSPECIFIED. ) ;
#6860=CARTESIAN_POINT ( 'NONE',  ( 61.25000000000003553, -1.039502773796944890, 1.800471618824829756 ) ) ;
#6862=FACE_OUTER_BOUND ( 'NONE', #30137, .T. ) ;
#6874=CARTESIAN_POINT ( 'NONE',  ( 50.95599726996783829, 0.9532299437236954054, -1.316046228059489120 ) ) ;
#6876=EDGE_LOOP ( 'NONE', ( #5474, #6254, #25928, #30692, #19504 ) ) ;
#6877=DIRECTION ( 'NONE',  ( -0.000000000000000000, -0.000000000000000000, -1.000000000000000000 ) ) ;
#6882=CIRCLE ( 'NONE', #20546, 0.1500000000000001887 ) ;
#6889=CARTESIAN_POINT ( 'NONE',  ( 50.50000000000002132, 5.291762632692320630E-13, -1.996089927833914146 ) ) ;
#6890=B_SPLINE_CURVE_WITH_KNOTS ( 'NONE', 3,
 ( #6725, #23839, #6418, #11015, #20693, #16081, #30318, #8626, #27942, #6258 ),
 .UNSPECIFIED., .F., .F.,
 ( 4, 2, 2, 2, 4 ),
 ( 0.000000000000000000, 9.706686070839353657E-05, 0.0001941337214167870731, 0.0002912005821251806097, 0.0003882674428335743089 ),
 .UNSPECIFIED. ) ;
#6891=FACE_OUTER_BOUND ( 'NONE', #5653, .T. ) ;
#6894=CARTESIAN_POINT ( 'NONE',  ( 58.65000000000004121, -1.793224408421451477, 0.5487562170608006884 ) ) ;
#6895=CARTESIAN_POINT ( 'NONE',  ( 58.65000000000001990, -0.5811678240976237975, -1.782657835994593487 ) ) ;
#6899=CARTESIAN_POINT ( 'NONE',  ( 51.31943556899493331, 1.088761256244167086, 1.206353010735628395 ) ) ;
#6925=CIRCLE ( 'NONE', #24602, 0.1000000000000001027 ) ;
#6928=CARTESIAN_POINT ( 'NONE',  ( 58.75000000000000000, 1.782657835995382190, -0.5811678240976815291 ) ) ;
#6929=B_SPLINE_CURVE_WITH_KNOTS ( 'NONE', 3,
 ( #22371, #10034, #2593, #7500 ),
 .UNSPECIFIED., .F., .F.,
 ( 4, 4 ),
 ( 6.653267247438212099E-05, 0.0002183616642542154668 ),
 .UNSPECIFIED. ) ;
#6936=AXIS2_PLACEMENT_3D ( 'NONE', #25566, #16085, #23369 ) ;
#6939=AXIS2_PLACEMENT_3D ( 'NONE', #4347, #14480, #7356 ) ;
#6944=ORIENTED_EDGE ( 'NONE', *, *, #15111, .F. ) ;
#6947=AXIS2_PLACEMENT_3D ( 'NONE', #12616, #5184, #27021 ) ;
#6952=AXIS2_PLACEMENT_3D ( 'NONE', #989, #18249, #25668 ) ;
#6958=ORIENTED_EDGE ( 'NONE', *, *, #6324, .F. ) ;
#6960=VECTOR ( 'NONE', #3285, 1000.000000000000000 ) ;
#6976=CIRCLE ( 'NONE', #30235, 1.875000000000001776 ) ;
#6982=EDGE_CURVE ( 'NONE', #16343, #29981, #25297, .T. ) ;
#6985=AXIS2_PLACEMENT_3D ( 'NONE', #5476, #13206, #13058 ) ;
#6993=CARTESIAN_POINT ( 'NONE',  ( 58.74154451056429593, -1.832994048937183429, 0.3947215634758409197 ) ) ;
#6999=ORIENTED_EDGE ( 'NONE', *, *, #28902, .T. ) ;
#7000=ORIENTED_EDGE ( 'NONE', *, *, #11316, .T. ) ;
#7006=DIRECTION ( 'NONE',  ( 0.000000000000000000, 0.000000000000000000, 1.000000000000000000 ) ) ;
#7008=FACE_OUTER_BOUND ( 'NONE', #21008, .T. ) ;
#7017=DIRECTION ( 'NONE',  ( 0.000000000000000000, 0.000000000000000000, 1.000000000000000000 ) ) ;
#7018=AXIS2_PLACEMENT_3D ( 'NONE', #16441, #18987, #21375 ) ;
#7021=EDGE_CURVE ( 'NONE', #4586, #16552, #2910, .T. ) ;
#7023=CARTESIAN_POINT ( 'NONE',  ( 61.25000000000002132, 6.415596960124259844E-13, 3.111507638930570854E-58 ) ) ;
#7025=CARTESIAN_POINT ( 'NONE',  ( 52.20711756518984004, -0.4999999999994533817, 1.718465885608440491 ) ) ;
#7028=B_SPLINE_CURVE_WITH_KNOTS ( 'NONE', 3,
 ( #18493, #28136, #1681, #11342 ),
 .UNSPECIFIED., .F., .F.,
 ( 4, 4 ),
 ( 5.935267624065488723E-05, 0.0002061672048306624071 ),
 .UNSPECIFIED. ) ;
#7031=VERTEX_POINT ( 'NONE', #26853 ) ;
#7032=CARTESIAN_POINT ( 'NONE',  ( 58.65000000000002700, -0.8948927608030060599, -1.760622601996600922 ) ) ;
#7041=VERTEX_POINT ( 'NONE', #24788 ) ;
#7044=VERTEX_POINT ( 'NONE', #17674 ) ;
#7051=CARTESIAN_POINT ( 'NONE',  ( 58.65000000000001990, 6.143261415694495821E-13, 3.111507638930570854E-58 ) ) ;
#7056=CARTESIAN_POINT ( 'NONE',  ( 58.75000000694009117, -0.9428687169905247689, -1.682988785000552934 ) ) ;
#7061=EDGE_CURVE ( 'NONE', #13972, #21159, #14383, .T. ) ;
#7063=CARTESIAN_POINT ( 'NONE',  ( 58.75000000000002132, -0.4991218602006210481, -1.863314270025920649 ) ) ;
#7065=CARTESIAN_POINT ( 'NONE',  ( 58.72153194576689117, -0.4999999999993851585, 1.827449685319723738 ) ) ;
#7066=CARTESIAN_POINT ( 'NONE',  ( 50.25000000000000000, 1.996089927834441502, -0.1249999999989956784 ) ) ;
#7078=CARTESIAN_POINT ( 'NONE',  ( 60.87997700083086272, 0.6727827007665463377, -1.479885446458162113 ) ) ;
#7087=VECTOR ( 'NONE', #29550, 1000.000000000000000 ) ;
#7088=DIRECTION ( 'NONE',  ( 1.000000000000000000, 1.047444401652940007E-14, -0.000000000000000000 ) ) ;
#7099=AXIS2_PLACEMENT_3D ( 'NONE', #11157, #27792, #25556 ) ;
#7110=CARTESIAN_POINT ( 'NONE',  ( 58.72419296898065255, 0.9760445624820607291, -1.601054456121077330 ) ) ;
#7117=CARTESIAN_POINT ( 'NONE',  ( 52.20711756518982583, 0.7500000000005468959, -1.718465885608440269 ) ) ;
#7123=EDGE_CURVE ( 'NONE', #12424, #1382, #28853, .T. ) ;
#7125=DIRECTION ( 'NONE',  ( 0.000000000000000000, 0.8381322357044638238, 0.5454670984331106975 ) ) ;
#7132=EDGE_CURVE ( 'NONE', #23389, #15285, #20829, .T. ) ;
#7144=CARTESIAN_POINT ( 'NONE',  ( 58.75000000000004263, -1.871971993774602661, 0.6020210199438860155 ) ) ;
#7149=ORIENTED_EDGE ( 'NONE', *, *, #29166, .F. ) ;
#7151=CIRCLE ( 'NONE', #11175, 0.2500000000000000000 ) ;
#7152=DIRECTION ( 'NONE',  ( 0.000000000000000000, 0.6683962987614510132, -0.7438053426818022063 ) ) ;
#7153=VERTEX_POINT ( 'NONE', #15757 ) ;
#7156=EDGE_LOOP ( 'NONE', ( #11793, #19924, #10896, #4507, #24627, #29866, #20367, #16383, #31311, #12556, #14506, #9907 ) ) ;
#7158=CARTESIAN_POINT ( 'NONE',  ( 58.65266784251152643, 1.873893454699072869, 0.06654060276385889705 ) ) ;
#7172=DIRECTION ( 'NONE',  ( 0.000000000000000000, 0.000000000000000000, 1.000000000000000000 ) ) ;
#7191=DIRECTION ( 'NONE',  ( 1.000000000000000000, 1.047444401652940007E-14, 0.000000000000000000 ) ) ;
#7193=AXIS2_PLACEMENT_3D ( 'NONE', #2047, #21236, #25637 ) ;
#7202=ORIENTED_EDGE ( 'NONE', *, *, #967, .T. ) ;
#7205=CARTESIAN_POINT ( 'NONE',  ( 58.74160516400036158, -1.017053542743307171, -1.575205926126072908 ) ) ;
#7218=( BOUNDED_SURFACE ( )  B_SPLINE_SURFACE ( 3, 2, ( 
 ( #11580, #6345, #25353 ),
 ( #16171, #3659, #22986 ),
 ( #8412, #28203, #3973 ),
 ( #15706, #16004, #1586 ),
 ( #25666, #13613, #13924 ),
 ( #8564, #18393, #23450 ),
 ( #11247, #11407, #23621 ),
 ( #1737, #27735, #15845 ),
 ( #8864, #9042, #23154 ),
 ( #30405, #25497, #18555 ) ),
 .UNSPECIFIED., .F., .F., .F. ) 
 B_SPLINE_SURFACE_WITH_KNOTS ( ( 4, 2, 2, 2, 4 ),
 ( 3, 3 ),
 ( 0.0001706658715692554269, 0.0002229276920778087870, 0.0002751895125863621470, 0.0003274513330949155613, 0.0003797131536034689214 ),
 ( 0.000000000000000000, 1.000000000000000000 ),
 .UNSPECIFIED. ) 
 GEOMETRIC_REPRESENTATION_ITEM ( )  RATIONAL_B_SPLINE_SURFACE ( (
 ( 1.000000000000000000, 0.7071067811865192621, 1.000000000000000000),
 ( 1.000000000000000000, 0.7375607040701905870, 1.000000000000000000),
 ( 1.000000000000000000, 0.7730431127427920268, 1.000000000000000000),
 ( 1.000000000000000000, 0.8321012486986795187, 1.000000000000000000),
 ( 1.000000000000000000, 0.8541932017409041844, 1.000000000000000000),
 ( 1.000000000000000000, 0.8545723906061826192, 1.000000000000000000),
 ( 1.000000000000000000, 0.8327032135051340989, 1.000000000000000000),
 ( 1.000000000000000000, 0.7734559727061557366, 1.000000000000000000),
 ( 1.000000000000000000, 0.7377766653997592794, 1.000000000000000000),
 ( 1.000000000000000000, 0.7071067811865198172, 1.000000000000000000) ) ) 
 REPRESENTATION_ITEM ( '' )  SURFACE ( )  );
#7222=PLANE ( 'NONE',  #1901 ) ;
#7225=ORIENTED_EDGE ( 'NONE', *, *, #25092, .F. ) ;
#7229=CARTESIAN_POINT ( 'NONE',  ( 50.50000000000002842, -0.7374999999994747979, 1.362419564051435130E-16 ) ) ;
#7242=CARTESIAN_POINT ( 'NONE',  ( 58.75000000000002132, 6.153735859711025284E-13, 3.111507638930570854E-58 ) ) ;
#7243=ORIENTED_EDGE ( 'NONE', *, *, #29449, .T. ) ;
#7245=CARTESIAN_POINT ( 'NONE',  ( 58.65000000000000568, 1.372267738822026573, -1.278133834459896478 ) ) ;
#7256=CARTESIAN_POINT ( 'NONE',  ( 50.78793970012933556, 0.4223115601901949456, -0.9680023493207204899 ) ) ;
#7258=CARTESIAN_POINT ( 'NONE',  ( 58.75000000000000711, 0.8495817349399600316, 1.671477153794648229 ) ) ;
#7262=DIRECTION ( 'NONE',  ( 0.000000000000000000, 0.000000000000000000, 1.000000000000000000 ) ) ;
#7280=AXIS2_PLACEMENT_3D ( 'NONE', #16965, #14581, #7152 ) ;
#7288=CARTESIAN_POINT ( 'NONE',  ( 51.85262340636813860, -0.6891204047484754680, -1.750401715244590539 ) ) ;
#7293=CIRCLE ( 'NONE', #24974, 0.1500000000000001887 ) ;
#7296=ADVANCED_FACE ( 'NONE', ( #23832 ), #4657, .F. ) ;
#7317=DIRECTION ( 'NONE',  ( 0.000000000000000000, 0.5454670984320038052, 0.8381322357051842475 ) ) ;
#7324=CARTESIAN_POINT ( 'NONE',  ( 51.23644008536121675, 1.080112125196981410, -1.214076932077873039 ) ) ;
#7327=ADVANCED_FACE ( 'NONE', ( #26354 ), #30355, .F. ) ;
#7333=ORIENTED_EDGE ( 'NONE', *, *, #13390, .F. ) ;
#7339=EDGE_LOOP ( 'NONE', ( #10725, #26159, #29671, #22346, #25362, #19851 ) ) ;
#7343=CARTESIAN_POINT ( 'NONE',  ( 50.78793970012933556, 0.4223115601901947791, 0.9680023493207204899 ) ) ;
#7356=DIRECTION ( 'NONE',  ( 0.000000000000000000, 0.3099561728523109738, -0.9507508458638090909 ) ) ;
#7358=DIRECTION ( 'NONE',  ( 0.000000000000000000, 0.000000000000000000, -1.000000000000000000 ) ) ;
#7359=EDGE_CURVE ( 'NONE', #16552, #11068, #30080, .T. ) ;
#7367=ORIENTED_EDGE ( 'NONE', *, *, #3362, .T. ) ;
#7372=DIRECTION ( 'NONE',  ( 0.000000000000000000, 0.000000000000000000, 1.000000000000000000 ) ) ;
#7380=EDGE_CURVE ( 'NONE', #29298, #29220, #16469, .T. ) ;
#7383=CARTESIAN_POINT ( 'NONE',  ( 58.65000000000003411, -1.571497941946429444, 1.022750809560281970 ) ) ;
#7384=AXIS2_PLACEMENT_3D ( 'NONE', #22164, #7879, #17388 ) ;
#7397=AXIS2_PLACEMENT_3D ( 'NONE', #30281, #8591, #27910 ) ;
#7404=VERTEX_POINT ( 'NONE', #21156 ) ;
#7415=CARTESIAN_POINT ( 'NONE',  ( 58.66118217212531505, 0.9228675180758563190, -1.632243256842949464 ) ) ;
#7417=VERTEX_POINT ( 'NONE', #10184 ) ;
#7419=DIRECTION ( 'NONE',  ( 0.000000000000000000, -1.000000000000000000, 0.000000000000000000 ) ) ;
#7423=LINE ( 'NONE', #12306, #29713 ) ;
#7431=AXIS2_PLACEMENT_3D ( 'NONE', #25923, #14040, #1686 ) ;
#7438=DIRECTION ( 'NONE',  ( 0.000000000000000000, 0.000000000000000000, 1.000000000000000000 ) ) ;
#7446=CARTESIAN_POINT ( 'NONE',  ( 61.23837541685315244, -0.8927489269147697026, 1.767200183694116244 ) ) ;
#7448=DIRECTION ( 'NONE',  ( 9.188255586753834161E-15, -0.8381322357045576377, -0.5454670984329669237 ) ) ;
#7451=CARTESIAN_POINT ( 'NONE',  ( 58.66118217212473240, -1.806736155626957663, 0.5016043952914784887 ) ) ;
#7453=CARTESIAN_POINT ( 'NONE',  ( 50.25000000000003553, -1.666164585742576421, -1.106298139390194724 ) ) ;
#7456=CARTESIAN_POINT ( 'NONE',  ( 58.64999999999999858, 1.932246131437592052, 0.4087173687853762338 ) ) ;
#7460=DIRECTION ( 'NONE',  ( 0.000000000000000000, 0.000000000000000000, 1.000000000000000000 ) ) ;
#7461=VERTEX_POINT ( 'NONE', #26821 ) ;
#7464=AXIS2_PLACEMENT_3D ( 'NONE', #25913, #16593, #14028 ) ;
#7473=EDGE_CURVE ( 'NONE', #2793, #29835, #29834, .T. ) ;
#7479=CARTESIAN_POINT ( 'NONE',  ( 60.88100035777595309, -0.5130564158037707045, -1.858165151418244010 ) ) ;
#7484=EDGE_CURVE ( 'NONE', #4931, #29991, #28876, .T. ) ;
#7494=CARTESIAN_POINT ( 'NONE',  ( 58.75000000000003553, -1.469015551795666452, 1.320082690054176666 ) ) ;
#7495=CARTESIAN_POINT ( 'NONE',  ( 58.75000000000002132, 6.153735859711025284E-13, 3.111507638930570854E-58 ) ) ;
#7500=CARTESIAN_POINT ( 'NONE',  ( 51.45655683570189609, 0.9591657938401613182, 1.611094652690528317 ) ) ;
#7503=CARTESIAN_POINT ( 'NONE',  ( 60.98985426489756634, 0.5466942006297351719, -1.538695758318366691 ) ) ;
#7509=DIRECTION ( 'NONE',  ( 0.000000000000000000, 0.6683962987610957418, 0.7438053426821212843 ) ) ;
#7511=ORIENTED_EDGE ( 'NONE', *, *, #29422, .F. ) ;
#7516=ORIENTED_EDGE ( 'NONE', *, *, #24684, .T. ) ;
#7521=CARTESIAN_POINT ( 'NONE',  ( 58.65844932252345245, -0.9087029769943339996, -1.640171707772822396 ) ) ;
#7531=DIRECTION ( 'NONE',  ( 0.000000000000000000, -0.3099561728522105541, -0.9507508458638417315 ) ) ;
#7532=ORIENTED_EDGE ( 'NONE', *, *, #28171, .F. ) ;
#7535=AXIS2_PLACEMENT_3D ( 'NONE', #6860, #16526, #26183 ) ;
#7540=DIRECTION ( 'NONE',  ( 0.000000000000000000, 0.000000000000000000, 1.000000000000000000 ) ) ;
#7544=VERTEX_POINT ( 'NONE', #29649 ) ;
#7550=ADVANCED_FACE ( 'NONE', ( #29346 ), #9735, .F. ) ;
#7559=DIRECTION ( 'NONE',  ( -0.8262273428075421755, -0.5633368246415177971, 0.000000000000000000 ) ) ;
#7560=CARTESIAN_POINT ( 'NONE',  ( 58.75000000000002132, 6.153735859711025284E-13, 3.111507638930570854E-58 ) ) ;
#7563=ORIENTED_EDGE ( 'NONE', *, *, #2544, .F. ) ;
#7564=CARTESIAN_POINT ( 'NONE',  ( 61.25000000000000711, 1.470078920827461166, 1.470078920828533420 ) ) ;
#7565=CARTESIAN_POINT ( 'NONE',  ( 51.40674769956039114, -0.9873535814794003329, -1.422142864483648461 ) ) ;
#7572=DIRECTION ( 'NONE',  ( 0.000000000000000000, 0.000000000000000000, -1.000000000000000000 ) ) ;
#7573=CARTESIAN_POINT ( 'NONE',  ( 58.66107449606953139, 0.9081280691414966855, 1.640741681270895036 ) ) ;
#7574=CARTESIAN_POINT ( 'NONE',  ( 58.65000000000004121, -1.782657835994225781, -0.5811678240974800236 ) ) ;
#7586=DIRECTION ( 'NONE',  ( -1.000000000000000000, -1.047444401652940007E-14, -0.000000000000000000 ) ) ;
#7589=CARTESIAN_POINT ( 'NONE',  ( 58.64999999999992752, -1.972190280207374968, 0.1053114364786527507 ) ) ;
#7596=DIRECTION ( 'NONE',  ( -7.790947421114572685E-15, 0.7438053426816656488, -0.6683962987616028917 ) ) ;
#7601=CARTESIAN_POINT ( 'NONE',  ( 58.73309930451056005, 0.5681566835776329372, 1.786899855580384555 ) ) ;
#7604=CARTESIAN_POINT ( 'NONE',  ( 58.65844932252318245, -1.819473848873478516, 0.4532319986951370838 ) ) ;
#7612=EDGE_LOOP ( 'NONE', ( #3665, #27999, #18323, #19364 ) ) ;
#7631=CARTESIAN_POINT ( 'NONE',  ( 50.56951033778286586, -0.1019484954143860672, -1.190698274346102092 ) ) ;
#7633=CARTESIAN_POINT ( 'NONE',  ( 50.25000000000000000, 1.666164585742626159, 1.106298139391201030 ) ) ;
#7640=CARTESIAN_POINT ( 'NONE',  ( 51.39880218607839168, -0.9985439640369458969, -1.587650844584835852 ) ) ;
#7643=EDGE_LOOP ( 'NONE', ( #23859, #11767, #3359, #13508 ) ) ;
#7647=VERTEX_POINT ( 'NONE', #20336 ) ;
#7648=ORIENTED_EDGE ( 'NONE', *, *, #3216, .T. ) ;
#7654=ORIENTED_EDGE ( 'NONE', *, *, #27488, .T. ) ;
#7663=DIRECTION ( 'NONE',  ( 0.000000000000000000, 0.000000000000000000, 1.000000000000000000 ) ) ;
#7664=CARTESIAN_POINT ( 'NONE',  ( 52.06628335902944826, 0.5434431642986584654, 1.794517909405660250 ) ) ;
#7666=EDGE_CURVE ( 'NONE', #15285, #21568, #19684, .T. ) ;
#7668=CARTESIAN_POINT ( 'NONE',  ( 58.75000000000003553, -1.022750809560422525, 1.571497941946552901 ) ) ;
#7671=VECTOR ( 'NONE', #12713, 1000.000000000000000 ) ;
#7673=VERTEX_POINT ( 'NONE', #29965 ) ;
#7680=DIRECTION ( 'NONE',  ( 1.000000000000000000, 1.047444401652940007E-14, 0.000000000000000000 ) ) ;
#7681=CYLINDRICAL_SURFACE ( 'NONE', #5062, 0.1500000000000000777 ) ;
#7682=ORIENTED_EDGE ( 'NONE', *, *, #20337, .T. ) ;
#7688=ORIENTED_EDGE ( 'NONE', *, *, #23564, .T. ) ;
#7703=ORIENTED_EDGE ( 'NONE', *, *, #25651, .F. ) ;
#7707=DIRECTION ( 'NONE',  ( 1.000000000000000000, 1.047444401652940007E-14, 0.000000000000000000 ) ) ;
#7714=CARTESIAN_POINT ( 'NONE',  ( 58.75000000000002842, -0.8897917884444737080, 1.791164585743103999 ) ) ;
#7717=CARTESIAN_POINT ( 'NONE',  ( 61.02723049001807709, -0.5636288612503438378, -1.705074539937696976 ) ) ;
#7728=CIRCLE ( 'NONE', #26449, 1.875000000000000222 ) ;
#7734=DIRECTION ( 'NONE',  ( 0.8023336663629262455, -0.5470456816110725873, 0.2387503090077610912 ) ) ;
#7736=CARTESIAN_POINT ( 'NONE',  ( 61.23787131559264907, -0.8905369330980658082, 1.779178344870881556 ) ) ;
#7737=CARTESIAN_POINT ( 'NONE',  ( 61.25000000000002132, 6.415596960124259844E-13, 3.111507638930570854E-58 ) ) ;
#7743=DIRECTION ( 'NONE',  ( 0.000000000000000000, 0.5333333333333335480, 0.8459051693633012903 ) ) ;
#7748=AXIS2_PLACEMENT_3D ( 'NONE', #13923, #23302, #4126 ) ;
#7752=CARTESIAN_POINT ( 'NONE',  ( 51.89360908398765559, 0.6611756245550114430, 1.497563819581031241 ) ) ;
#7754=DIRECTION ( 'NONE',  ( -1.000000000000000000, -1.047444401652940007E-14, 0.000000000000000000 ) ) ;
#7771=CARTESIAN_POINT ( 'NONE',  ( 61.23770293222991512, 0.8897917884447287262, -1.791164585742097914 ) ) ;
#7775=LINE ( 'NONE', #5102, #31181 ) ;
#7779=ORIENTED_EDGE ( 'NONE', *, *, #21581, .T. ) ;
#7785=ORIENTED_EDGE ( 'NONE', *, *, #5984, .F. ) ;
#7787=DIRECTION ( 'NONE',  ( 1.000000000000000000, 1.047444401652940007E-14, 0.000000000000000000 ) ) ;
#7796=ORIENTED_EDGE ( 'NONE', *, *, #27040, .F. ) ;
#7799=CIRCLE ( 'NONE', #20455, 0.1500000000000003830 ) ;
#7811=AXIS2_PLACEMENT_3D ( 'NONE', #442, #27024, #18803 ) ;
#7813=CARTESIAN_POINT ( 'NONE',  ( 52.20711756518983293, 0.5000000000005468959, -1.807104036850122109 ) ) ;
#7818=VERTEX_POINT ( 'NONE', #31017 ) ;
#7820=EDGE_LOOP ( 'NONE', ( #26464, #482, #28128, #29593, #16891 ) ) ;
#7838=CIRCLE ( 'NONE', #26560, 0.2500000000000002776 ) ;
#7842=CARTESIAN_POINT ( 'NONE',  ( 58.65000000000000568, 1.827356000910769440, 0.4213753797520914390 ) ) ;
#7844=DIRECTION ( 'NONE',  ( 1.000000000000000000, 1.047444401652940007E-14, 0.000000000000000000 ) ) ;
#7852=EDGE_CURVE ( 'NONE', #3598, #4273, #16088, .T. ) ;
#7854=CARTESIAN_POINT ( 'NONE',  ( 58.75000000000000711, 1.039502773796331159, 1.800471618825331355 ) ) ;
#7855=CARTESIAN_POINT ( 'NONE',  ( 51.43355796162965987, -0.9748468443428969232, -1.443681521171313653 ) ) ;
#7861=VECTOR ( 'NONE', #22461, 1000.000000000000000 ) ;
#7863=DIRECTION ( 'NONE',  ( 0.000000000000000000, 0.000000000000000000, 1.000000000000000000 ) ) ;
#7866=ORIENTED_EDGE ( 'NONE', *, *, #6050, .T. ) ;
#7871=VERTEX_POINT ( 'NONE', #295 ) ;
#7873=FACE_OUTER_BOUND ( 'NONE', #19412, .T. ) ;
#7878=CARTESIAN_POINT ( 'NONE',  ( 58.66122797211882300, 1.632010475559142915, -0.9232791089886424052 ) ) ;
#7879=DIRECTION ( 'NONE',  ( 1.000000000000000000, 1.047444401652940007E-14, 0.000000000000000000 ) ) ;
#7880=DIRECTION ( 'NONE',  ( 0.000000000000000000, 0.000000000000000000, 1.000000000000000000 ) ) ;
#7885=ORIENTED_EDGE ( 'NONE', *, *, #20587, .T. ) ;
#7892=AXIS2_PLACEMENT_3D ( 'NONE', #4289, #13938, #28218 ) ;
#7894=EDGE_CURVE ( 'NONE', #27829, #18852, #28347, .T. ) ;
#7895=ADVANCED_FACE ( 'NONE', ( #1079 ), #22635, .T. ) ;
#7901=FACE_OUTER_BOUND ( 'NONE', #29581, .T. ) ;
#7902=AXIS2_PLACEMENT_3D ( 'NONE', #4780, #10022, #26479 ) ;
#7907=CARTESIAN_POINT ( 'NONE',  ( 58.74840439586703411, -0.4999999999993848254, -1.859896009349159884 ) ) ;
#7908=STYLED_ITEM ( 'NONE', ( #13793 ), #15609 ) ;
#7916=AXIS2_PLACEMENT_3D ( 'NONE', #20802, #28385, #21432 ) ;
#7919=( BOUNDED_SURFACE ( )  B_SPLINE_SURFACE ( 3, 2, ( 
 ( #24595, #5604, #29350 ),
 ( #5447, #383, #10339 ),
 ( #14927, #22246, #24898 ),
 ( #8129, #15097, #5130 ) ),
 .UNSPECIFIED., .F., .F., .F. ) 
 B_SPLINE_SURFACE_WITH_KNOTS ( ( 4, 4 ),
 ( 3, 3 ),
 ( 1.982313172862385287, 2.241731514487932841 ),
 ( 0.000000000000000000, 1.000000000000000000 ),
 .UNSPECIFIED. ) 
 GEOMETRIC_REPRESENTATION_ITEM ( )  RATIONAL_B_SPLINE_SURFACE ( (
 ( 1.000000000000000000, 0.8156258140602938855, 1.000000000000000000),
 ( 1.000000000000000000, 0.8356979842195433328, 1.000000000000000000),
 ( 1.000000000000000000, 0.8538860448759271193, 1.000000000000000000),
 ( 1.000000000000000000, 0.8699658093904928391, 1.000000000000000000) ) ) 
 REPRESENTATION_ITEM ( '' )  SURFACE ( )  );
#7923=CARTESIAN_POINT ( 'NONE',  ( 58.72419296898084440, -1.293880926823457900, -1.357170035999710089 ) ) ;
#7928=VERTEX_POINT ( 'NONE', #15174 ) ;
#7938=FACE_OUTER_BOUND ( 'NONE', #24670, .T. ) ;
#7941=AXIS2_PLACEMENT_3D ( 'NONE', #15627, #5800, #23061 ) ;
#7942=CARTESIAN_POINT ( 'NONE',  ( 52.06628335902944826, 0.5434431642986584654, 1.794517909405660250 ) ) ;
#7956=ORIENTED_EDGE ( 'NONE', *, *, #31253, .F. ) ;
#7959=AXIS2_PLACEMENT_3D ( 'NONE', #28477, #18988, #28943 ) ;
#7961=VECTOR ( 'NONE', #25617, 1000.000000000000000 ) ;
#7963=CARTESIAN_POINT ( 'NONE',  ( 58.75000000000002132, 6.153735859711025284E-13, 3.111507638930570854E-58 ) ) ;
#7979=EDGE_CURVE ( 'NONE', #23889, #10218, #16240, .T. ) ;
#7985=CYLINDRICAL_SURFACE ( 'NONE', #8436, 0.1500000000000001887 ) ;
#8008=CARTESIAN_POINT ( 'NONE',  ( 51.47729133425608694, 0.9526829978903045282, -1.321356857234299520 ) ) ;
#8032=CARTESIAN_POINT ( 'NONE',  ( 50.25000000000002842, -0.5380862305904318132, -2.008165151418244143 ) ) ;
#8044=CARTESIAN_POINT ( 'NONE',  ( 58.75000000000002132, 6.153735859711025284E-13, 3.111507638930570854E-58 ) ) ;
#8048=CARTESIAN_POINT ( 'NONE',  ( 58.75000000694005564, 1.682988785001006793, -0.9428687169902416620 ) ) ;
#8052=DIRECTION ( 'NONE',  ( 1.000000000000000000, 1.047444401652940007E-14, 0.000000000000000000 ) ) ;
#8057=DIRECTION ( 'NONE',  ( 0.000000000000000000, 0.000000000000000000, 1.000000000000000000 ) ) ;
#8068=ORIENTED_EDGE ( 'NONE', *, *, #7132, .T. ) ;
#8069=AXIS2_PLACEMENT_3D ( 'NONE', #26945, #3193, #12835 ) ;
#8072=LINE ( 'NONE', #22810, #21706 ) ;
#8074=FACE_OUTER_BOUND ( 'NONE', #12878, .T. ) ;
#8075=EDGE_CURVE ( 'NONE', #15123, #7818, #5645, .T. ) ;
#8077=ORIENTED_EDGE ( 'NONE', *, *, #28892, .F. ) ;
#8083=DIRECTION ( 'NONE',  ( 1.000000000000000000, 1.047444401652940007E-14, 0.000000000000000000 ) ) ;
#8092=AXIS2_PLACEMENT_3D ( 'NONE', #919, #18183, #1067 ) ;
#8097=CARTESIAN_POINT ( 'NONE',  ( 50.25000000000003553, -1.666164585743077131, 1.106298139390331947 ) ) ;
#8098=CARTESIAN_POINT ( 'NONE',  ( 58.74999999999981526, -1.834410884275056386, -0.3880228184668537694 ) ) ;
#8108=PLANE ( 'NONE',  #2407 ) ;
#8109=EDGE_CURVE ( 'NONE', #2034, #507, #16119, .T. ) ;
#8114=ORIENTED_EDGE ( 'NONE', *, *, #23479, .T. ) ;
#8117=ORIENTED_EDGE ( 'NONE', *, *, #3762, .F. ) ;
#8118=ORIENTED_EDGE ( 'NONE', *, *, #29176, .F. ) ;
#8129=CARTESIAN_POINT ( 'NONE',  ( 51.59739104186226655, 1.010292945603183501, -1.272765950230259735 ) ) ;
#8131=CARTESIAN_POINT ( 'NONE',  ( 58.75000000000001421, 0.5380862305915540267, -1.858165151417984218 ) ) ;
#8140=CARTESIAN_POINT ( 'NONE',  ( 58.65263613458535019, 1.277852321299496552, -1.372222488449735378 ) ) ;
#8145=EDGE_CURVE ( 'NONE', #23567, #7041, #15252, .T. ) ;
#8153=ORIENTED_EDGE ( 'NONE', *, *, #22798, .T. ) ;
#8171=CARTESIAN_POINT ( 'NONE',  ( 50.56951033778286586, 0.1019484954154457890, 1.190698274346101648 ) ) ;
#8172=CYLINDRICAL_SURFACE ( 'NONE', #28140, 0.1500000000000001887 ) ;
#8175=B_SPLINE_CURVE_WITH_KNOTS ( 'NONE', 3,
 ( #5907, #13022, #17313, #5742, #15392, #25042 ),
 .UNSPECIFIED., .F., .F.,
 ( 4, 2, 4 ),
 ( 0.000000000000000000, 8.451199622854574779E-05, 0.0001690239924570914956 ),
 .UNSPECIFIED. ) ;
#8179=CARTESIAN_POINT ( 'NONE',  ( 51.47729133425627168, -0.9526829978892129569, 1.321356857233838777 ) ) ;
#8180=ORIENTED_EDGE ( 'NONE', *, *, #2379, .F. ) ;
#8183=ORIENTED_EDGE ( 'NONE', *, *, #26237, .F. ) ;
#8192=CARTESIAN_POINT ( 'NONE',  ( 61.00000000000003553, -0.8666666666660277629, -1.374595900215364708 ) ) ;
#8195=DIRECTION ( 'NONE',  ( 0.000000000000000000, 0.7438053426816615410, -0.6683962987616075546 ) ) ;
#8199=CARTESIAN_POINT ( 'NONE',  ( 58.75000000000003553, -1.323060376181803832, 1.499837071478349326 ) ) ;
#8202=CARTESIAN_POINT ( 'NONE',  ( 58.72419296898052465, 1.645806614395798340, -0.8985315506020565834 ) ) ;
#8209=AXIS2_PLACEMENT_3D ( 'NONE', #1992, #16731, #28277 ) ;
#8213=CARTESIAN_POINT ( 'NONE',  ( 58.73379417893116994, -1.873409305145653292, 0.08040888200709349343 ) ) ;
#8218=ORIENTED_EDGE ( 'NONE', *, *, #28589, .T. ) ;
#8220=CARTESIAN_POINT ( 'NONE',  ( 51.85262340636813150, -0.6891204047484758011, 1.750401715244590539 ) ) ;
#8221=CARTESIAN_POINT ( 'NONE',  ( 51.25000000000001421, 0.6500000000005367040, 1.489337100860647967 ) ) ;
#8222=CARTESIAN_POINT ( 'NONE',  ( 58.73379417893119836, -1.267842757871934012, 1.381558089341300422 ) ) ;
#8224=VERTEX_POINT ( 'NONE', #26240 ) ;
#8227=VERTEX_POINT ( 'NONE', #24185 ) ;
#8231=AXIS2_PLACEMENT_3D ( 'NONE', #12767, #29875, #30019 ) ;
#8234=EDGE_CURVE ( 'NONE', #7417, #22240, #25873, .T. ) ;
#8235=CARTESIAN_POINT ( 'NONE',  ( 58.73371041428924144, -1.267950628961127757, -1.381461519773210522 ) ) ;
#8245=CARTESIAN_POINT ( 'NONE',  ( 58.75000018803721957, -1.857237022264228044, -0.5488434064257393663 ) ) ;
#8254=DIRECTION ( 'NONE',  ( 1.000000000000000000, 1.047444401652940007E-14, 0.000000000000000000 ) ) ;
#8258=EDGE_CURVE ( 'NONE', #16066, #30797, #21968, .T. ) ;
#8262=VERTEX_POINT ( 'NONE', #21825 ) ;
#8272=AXIS2_PLACEMENT_3D ( 'NONE', #8032, #14829, #17697 ) ;
#8275=VERTEX_POINT ( 'NONE', #9472 ) ;
#8289=CARTESIAN_POINT ( 'NONE',  ( 58.75000018803716983, 1.403930843797543293, -1.333992738915948051 ) ) ;
#8292=ORIENTED_EDGE ( 'NONE', *, *, #12677, .F. ) ;
#8300=DIRECTION ( 'NONE',  ( -4.636120533309209166E-15, 0.3099561728519886206, -0.9507508458639142290 ) ) ;
#8302=ORIENTED_EDGE ( 'NONE', *, *, #22179, .F. ) ;
#8304=DIRECTION ( 'NONE',  ( -4.439792124536519685E-15, 0.3099561728528805182, -0.9507508458636233506 ) ) ;
#8306=FACE_OUTER_BOUND ( 'NONE', #19591, .T. ) ;
#8315=EDGE_CURVE ( 'NONE', #7461, #21159, #18338, .T. ) ;
#8320=CARTESIAN_POINT ( 'NONE',  ( 58.75000002382375897, -0.5510104498256471750, 1.849358057802746425 ) ) ;
#8321=DIRECTION ( 'NONE',  ( 1.000000000000000000, 1.047444401652940007E-14, 0.000000000000000000 ) ) ;
#8324=CARTESIAN_POINT ( 'NONE',  ( 51.50435016707359637, -0.9265794315402090531, 1.339215852266876672 ) ) ;
#8328=CARTESIAN_POINT ( 'NONE',  ( 50.59602332238209499, 0.1408342061609073048, 0.8215393206232031176 ) ) ;
#8337=FACE_OUTER_BOUND ( 'NONE', #30706, .T. ) ;
#8349=CARTESIAN_POINT ( 'NONE',  ( 58.75000018595668649, 1.651828233789292222, -1.011330950599448109 ) ) ;
#8359=CIRCLE ( 'NONE', #24546, 1.975000000000001865 ) ;
#8363=CARTESIAN_POINT ( 'NONE',  ( 58.65263613458533598, -1.873885868624304729, 0.06672978513340610540 ) ) ;
#8366=EDGE_CURVE ( 'NONE', #10836, #23636, #21337, .T. ) ;
#8370=DIRECTION ( 'NONE',  ( 0.000000000000000000, 0.000000000000000000, 1.000000000000000000 ) ) ;
#8372=CIRCLE ( 'NONE', #22560, 0.09999999999999993616 ) ;
#8394=VECTOR ( 'NONE', #20312, 1000.000000000000000 ) ;
#8397=CARTESIAN_POINT ( 'NONE',  ( 51.45655683570189609, 0.9591657938401613182, 1.611094652690528317 ) ) ;
#8398=CARTESIAN_POINT ( 'NONE',  ( 58.72204580543426289, -1.816949979608304178, -0.4634803957297197186 ) ) ;
#8402=AXIS2_PLACEMENT_3D ( 'NONE', #18660, #11204, #9310 ) ;
#8403=DIRECTION ( 'NONE',  ( 0.000000000000000000, 0.000000000000000000, 1.000000000000000000 ) ) ;
#8404=LINE ( 'NONE', #30398, #8394 ) ;
#8410=CIRCLE ( 'NONE', #14475, 1.625000000000000222 ) ;
#8412=CARTESIAN_POINT ( 'NONE',  ( 58.74999981404330640, 1.909395380152493438, 0.4234853497079917872 ) ) ;
#8418=ORIENTED_EDGE ( 'NONE', *, *, #5617, .T. ) ;
#8426=VECTOR ( 'NONE', #19799, 1000.000000000000000 ) ;
#8431=TOROIDAL_SURFACE ( 'NONE', #3379, 1.975000000000001865, 0.1000000000000000056 ) ;
#8436=AXIS2_PLACEMENT_3D ( 'NONE', #1014, #17648, #12865 ) ;
#8443=FACE_OUTER_BOUND ( 'NONE', #23452, .T. ) ;
#8446=CIRCLE ( 'NONE', #6947, 2.000000000000000000 ) ;
#8459=ORIENTED_EDGE ( 'NONE', *, *, #20530, .F. ) ;
#8460=AXIS2_PLACEMENT_3D ( 'NONE', #1910, #25811, #21086 ) ;
#8463=CARTESIAN_POINT ( 'NONE',  ( 61.00000000000001421, 0.8666666666673057406, -1.374595900215365152 ) ) ;
#8466=ORIENTED_EDGE ( 'NONE', *, *, #27419, .T. ) ;
#8478=CIRCLE ( 'NONE', #20142, 0.2500000000000000000 ) ;
#8483=CARTESIAN_POINT ( 'NONE',  ( 58.65263613458532888, 1.372222488449602595, 1.277852321299682847 ) ) ;
#8487=CARTESIAN_POINT ( 'NONE',  ( 51.12687253673781385, -0.9194130538815391551, 1.491219977510798600 ) ) ;
#8488=CYLINDRICAL_SURFACE ( 'NONE', #23012, 0.2500000000000000000 ) ;
#8491=CARTESIAN_POINT ( 'NONE',  ( 60.75000000000001421, 0.6500000000006362910, -1.489337100860648189 ) ) ;
#8493=AXIS2_PLACEMENT_3D ( 'NONE', #13559, #25593, #18649 ) ;
#8495=ORIENTED_EDGE ( 'NONE', *, *, #20452, .T. ) ;
#8498=DIRECTION ( 'NONE',  ( 0.000000000000000000, 0.000000000000000000, 1.000000000000000000 ) ) ;
#8507=ORIENTED_EDGE ( 'NONE', *, *, #2508, .T. ) ;
#8511=CARTESIAN_POINT ( 'NONE',  ( 51.45655683570189609, 0.9591657938401613182, -1.611094652690528317 ) ) ;
#8512=ORIENTED_EDGE ( 'NONE', *, *, #10626, .T. ) ;
#8514=CARTESIAN_POINT ( 'NONE',  ( 58.74999981196283727, 1.734557215429400001, -0.9033020670118147022 ) ) ;
#8525=CARTESIAN_POINT ( 'NONE',  ( 58.65000000000004121, -1.872332544500606044, -0.09997921184723318477 ) ) ;
#8528=CARTESIAN_POINT ( 'NONE',  ( 58.74154451056412540, 1.575232816092658972, 1.017012227665773150 ) ) ;
#8531=CARTESIAN_POINT ( 'NONE',  ( 58.75000000000000711, 0.8495817349404619634, -1.671477153794393322 ) ) ;
#8550=CYLINDRICAL_SURFACE ( 'NONE', #18705, 0.1500000000000001887 ) ;
#8554=TOROIDAL_SURFACE ( 'NONE', #24748, 1.975000000000001865, 0.1000000000000000056 ) ;
#8555=CARTESIAN_POINT ( 'NONE',  ( 50.80258015808398397, 5.323456221955952384E-13, -1.996089927833914146 ) ) ;
#8564=CARTESIAN_POINT ( 'NONE',  ( 58.75000000694004854, 1.856761646088006978, 0.5233439189825915827 ) ) ;
#8587=EDGE_CURVE ( 'NONE', #36, #30639, #17603, .T. ) ;
#8589=CARTESIAN_POINT ( 'NONE',  ( 60.87107532335745930, 0.5000002988029885742, 1.554802360349133661 ) ) ;
#8591=DIRECTION ( 'NONE',  ( -0.8262273428075540549, 0.5633368246415005887, 0.000000000000000000 ) ) ;
#8595=FACE_OUTER_BOUND ( 'NONE', #14161, .T. ) ;
#8597=B_SPLINE_CURVE_WITH_KNOTS ( 'NONE', 3,
 ( #25230, #3075, #10524, #20348, #10348, #27448 ),
 .UNSPECIFIED., .F., .F.,
 ( 4, 2, 4 ),
 ( 0.0002203024014533751739, 0.0003053046653303950015, 0.0003903069292074148834 ),
 .UNSPECIFIED. ) ;
#8600=CARTESIAN_POINT ( 'NONE',  ( 51.25000000000001421, 5.368159983410797313E-13, 3.111507638930570854E-58 ) ) ;
#8601=CARTESIAN_POINT ( 'NONE',  ( 58.66118217212494557, -1.632243256842334844, -0.9228675180752388130 ) ) ;
#8604=ORIENTED_EDGE ( 'NONE', *, *, #5524, .F. ) ;
#8617=CARTESIAN_POINT ( 'NONE',  ( 58.65838214097809811, -1.606847897767968547, 0.9664062014974877934 ) ) ;
#8618=VERTEX_POINT ( 'NONE', #9425 ) ;
#8626=CARTESIAN_POINT ( 'NONE',  ( 51.18285175554922972, -0.9660043368199603409, 1.457922727165797294 ) ) ;
#8627=CARTESIAN_POINT ( 'NONE',  ( 51.31572262954152563, 1.002608958138273554, 1.584424273060082378 ) ) ;
#8628=CARTESIAN_POINT ( 'NONE',  ( 58.75000000000000711, 1.320165430233467552, 1.457266603154374618 ) ) ;
#8635=FACE_OUTER_BOUND ( 'NONE', #3353, .T. ) ;
#8643=EDGE_CURVE ( 'NONE', #4204, #17696, #13821, .T. ) ;
#8649=VERTEX_POINT ( 'NONE', #9267 ) ;
#8660=CARTESIAN_POINT ( 'NONE',  ( 58.75000018595668649, 1.857295262527451696, -0.5493460779666961002 ) ) ;
#8667=CARTESIAN_POINT ( 'NONE',  ( 58.75000000000001421, 0.5000000000004131140, 1.863080903344439321 ) ) ;
#8669=CARTESIAN_POINT ( 'NONE',  ( 61.00000000000002842, -0.8112099027092640746, -1.409560742431901437 ) ) ;
#8678=ORIENTED_EDGE ( 'NONE', *, *, #13910, .T. ) ;
#8684=CARTESIAN_POINT ( 'NONE',  ( 61.25000000000004263, -1.470078920827889268, 1.470078920827824209 ) ) ;
#8685=ORIENTED_EDGE ( 'NONE', *, *, #14452, .T. ) ;
#8693=CARTESIAN_POINT ( 'NONE',  ( 61.24796382359978253, 0.9549219522845532326, -1.676592304036239378 ) ) ;
#8699=CARTESIAN_POINT ( 'NONE',  ( 51.84772254680354564, -0.6924618999061495916, 1.653428777428161078 ) ) ;
#8708=VECTOR ( 'NONE', #30101, 1000.000000000000114 ) ;
#8721=ORIENTED_EDGE ( 'NONE', *, *, #13093, .T. ) ;
#8727=ORIENTED_EDGE ( 'NONE', *, *, #3174, .F. ) ;
#8730=CARTESIAN_POINT ( 'NONE',  ( 61.02723049001765077, 0.5636288612511761720, 1.705074539937785572 ) ) ;
#8736=DIRECTION ( 'NONE',  ( 0.000000000000000000, 0.000000000000000000, 1.000000000000000000 ) ) ;
#8738=DIRECTION ( 'NONE',  ( 0.000000000000000000, 0.000000000000000000, 1.000000000000000000 ) ) ;
#8745=ADVANCED_FACE ( 'NONE', ( #28573 ), #7919, .T. ) ;
#8751=CARTESIAN_POINT ( 'NONE',  ( 50.25000000000004263, -1.895722432253035050, 0.6373668173470157239 ) ) ;
#8752=ORIENTED_EDGE ( 'NONE', *, *, #1858, .T. ) ;
#8755=DIRECTION ( 'NONE',  ( 1.000000000000000000, 1.047444401652940007E-14, 0.000000000000000000 ) ) ;
#8757=CARTESIAN_POINT ( 'NONE',  ( 58.75000000694009827, -1.682988785000789855, 0.9428687169914291566 ) ) ;
#8770=CARTESIAN_POINT ( 'NONE',  ( 58.75000000694006275, 1.346330794793899166, 1.381609951798974834 ) ) ;
#8773=DIRECTION ( 'NONE',  ( 0.000000000000000000, 0.9985773570673163180, 0.05332224631852457153 ) ) ;
#8776=AXIS2_PLACEMENT_3D ( 'NONE', #24083, #14262, #7460 ) ;
#8778=CARTESIAN_POINT ( 'NONE',  ( 58.65000000000003411, -1.022750809560422747, 1.571497941946552457 ) ) ;
#8782=CIRCLE ( 'NONE', #20950, 0.1500000000000000777 ) ;
#8786=VERTEX_POINT ( 'NONE', #12710 ) ;
#8799=DIRECTION ( 'NONE',  ( 1.000000000000000000, 1.047444401652940007E-14, 0.000000000000000000 ) ) ;
#8804=PLANE ( 'NONE',  #18834 ) ;
#8822=CARTESIAN_POINT ( 'NONE',  ( 58.75000000694006275, 1.658042653848306625, 0.9860766836000441904 ) ) ;
#8833=ORIENTED_EDGE ( 'NONE', *, *, #2225, .F. ) ;
#8843=ORIENTED_EDGE ( 'NONE', *, *, #1652, .F. ) ;
#8847=CARTESIAN_POINT ( 'NONE',  ( 61.24504608472940248, 0.9290853280814357351, -1.697615787669267240 ) ) ;
#8850=DIRECTION ( 'NONE',  ( 0.000000000000000000, 0.000000000000000000, 1.000000000000000000 ) ) ;
#8853=CARTESIAN_POINT ( 'NONE',  ( 51.25000000000002842, -0.9938153758920951208, 1.589954715908409977 ) ) ;
#8859=CARTESIAN_POINT ( 'NONE',  ( 60.75000000000002842, -0.6499999999993638644, 1.489337100860647967 ) ) ;
#8861=ORIENTED_EDGE ( 'NONE', *, *, #21512, .F. ) ;
#8864=CARTESIAN_POINT ( 'NONE',  ( 58.75000000000000000, 1.871930101357349940, 0.6019471833021664553 ) ) ;
#8873=DIRECTION ( 'NONE',  ( 1.000000000000000000, 1.047444401652940007E-14, 0.000000000000000000 ) ) ;
#8876=CARTESIAN_POINT ( 'NONE',  ( 58.75000000000000000, 1.963941025093405957, 0.09694516908175258851 ) ) ;
#8892=LINE ( 'NONE', #28381, #27596 ) ;
#8897=AXIS2_PLACEMENT_3D ( 'NONE', #27806, #6263, #27643 ) ;
#8898=DIRECTION ( 'NONE',  ( 1.000000000000000000, 1.047444401652940007E-14, 0.000000000000000000 ) ) ;
#8901=CARTESIAN_POINT ( 'NONE',  ( 52.20711756518982583, 0.7500000000005468959, -1.718465885608440269 ) ) ;
#8903=CARTESIAN_POINT ( 'NONE',  ( 58.74999981196286569, -1.649561145038163756, -1.050519579371713252 ) ) ;
#8912=AXIS2_PLACEMENT_3D ( 'NONE', #3802, #17612, #27257 ) ;
#8924=CARTESIAN_POINT ( 'NONE',  ( 58.75000018803721247, -1.701355787207014192, 0.9251739982210235302 ) ) ;
#8925=ORIENTED_EDGE ( 'NONE', *, *, #17110, .T. ) ;
#8926=CYLINDRICAL_SURFACE ( 'NONE', #12528, 0.2500000000000000000 ) ;
#8929=( BOUNDED_CURVE ( )  B_SPLINE_CURVE ( 3, ( #5810, #17854, #25121, #5654 ),
 .UNSPECIFIED., .F., .T. ) 
 B_SPLINE_CURVE_WITH_KNOTS ( ( 4, 4 ),
 ( 4.041453792691655167, 4.300872134317202722 ),
 .UNSPECIFIED. ) 
 CURVE ( )  GEOMETRIC_REPRESENTATION_ITEM ( )  RATIONAL_B_SPLINE_CURVE ( ( 1.000000000000000000, 0.9943997021150918769, 0.9943997021150918769, 1.000000000000000000 ) ) 
 REPRESENTATION_ITEM ( '' )  );
#8938=LINE ( 'NONE', #28266, #13425 ) ;
#8952=VECTOR ( 'NONE', #1196, 1000.000000000000000 ) ;
#8953=CARTESIAN_POINT ( 'NONE',  ( 61.25000000000000000, 1.960427193528571532, 0.3958853607757182314 ) ) ;
#8954=VECTOR ( 'NONE', #11707, 1000.000000000000000 ) ;
#8970=DIRECTION ( 'NONE',  ( -1.000000000000000000, -1.047444401652940007E-14, -0.000000000000000000 ) ) ;
#8971=( BOUNDED_SURFACE ( )  B_SPLINE_SURFACE ( 3, 2, ( 
 ( #21646, #9603, #4351 ),
 ( #16394, #9277, #19263 ),
 ( #28899, #2462, #14482 ),
 ( #24157, #6585, #16244 ),
 ( #4193, #23517, #1816 ),
 ( #30803, #9116, #28429 ),
 ( #6733, #21329, #30962 ),
 ( #18940, #28584, #24448 ),
 ( #22254, #17188, #27134 ),
 ( #392, #7668, #10346 ) ),
 .UNSPECIFIED., .F., .F., .F. ) 
 B_SPLINE_SURFACE_WITH_KNOTS ( ( 4, 2, 2, 2, 4 ),
 ( 3, 3 ),
 ( 0.0001706658715701353925, 0.0002229276920781100868, 0.0002751895125860847539, 0.0003274513330940594211, 0.0003797131536020340883 ),
 ( 0.000000000000000000, 1.000000000000000000 ),
 .UNSPECIFIED. ) 
 GEOMETRIC_REPRESENTATION_ITEM ( )  RATIONAL_B_SPLINE_SURFACE ( (
 ( 1.000000000000000000, 0.7071067811873461562, 1.000000000000000000),
 ( 1.000000000000000000, 0.7375607040708931361, 1.000000000000000000),
 ( 1.000000000000000000, 0.7730431127425965165, 1.000000000000000000),
 ( 1.000000000000000000, 0.8321012486971868238, 1.000000000000000000),
 ( 1.000000000000000000, 0.8541932017382776188, 1.000000000000000000),
 ( 1.000000000000000000, 0.8545723906027511418, 1.000000000000000000),
 ( 1.000000000000000000, 0.8327032135021242842, 1.000000000000000000),
 ( 1.000000000000000000, 0.7734559727054323153, 1.000000000000000000),
 ( 1.000000000000000000, 0.7377766653991476575, 1.000000000000000000),
 ( 1.000000000000000000, 0.7071067811865509034, 1.000000000000000000) ) ) 
 REPRESENTATION_ITEM ( '' )  SURFACE ( )  );
#8980=CARTESIAN_POINT ( 'NONE',  ( 58.73371041428907091, 1.830356084956107798, -0.4073466955372750942 ) ) ;
#8987=EDGE_CURVE ( 'NONE', #16661, #15552, #2365, .T. ) ;
#9000=CARTESIAN_POINT ( 'NONE',  ( 51.45655683570189609, 0.9591657938401617622, 1.468576096419531352 ) ) ;
#9002=CARTESIAN_POINT ( 'NONE',  ( 58.74999981404332061, 1.734728236459932127, 0.9032433253523316496 ) ) ;
#9005=CARTESIAN_POINT ( 'NONE',  ( 58.75000000000003553, -1.469015551795666674, 1.320082690054176666 ) ) ;
#9006=ORIENTED_EDGE ( 'NONE', *, *, #12259, .F. ) ;
#9018=AXIS2_PLACEMENT_3D ( 'NONE', #25987, #9060, #11596 ) ;
#9033=( GEOMETRIC_REPRESENTATION_CONTEXT ( 3 ) GLOBAL_UNCERTAINTY_ASSIGNED_CONTEXT ( ( #10133 ) ) GLOBAL_UNIT_ASSIGNED_CONTEXT ( ( #18108, #5595, #20175 ) ) REPRESENTATION_CONTEXT ( 'NONE', 'WORKASPACE' ) );
#9039=FACE_OUTER_BOUND ( 'NONE', #9614, .T. ) ;
#9041=B_SPLINE_CURVE_WITH_KNOTS ( 'NONE', 3,
 ( #28720, #18903, #21137, #26006, #4633, #13963 ),
 .UNSPECIFIED., .F., .F.,
 ( 4, 2, 4 ),
 ( 0.000000000000000000, 0.0001924639855377290119, 0.0003849279710754580238 ),
 .UNSPECIFIED. ) ;
#9042=CARTESIAN_POINT ( 'NONE',  ( 58.74154451056408988, 1.784780193104163359, 0.5746581230792165984 ) ) ;
#9045=ORIENTED_EDGE ( 'NONE', *, *, #25736, .F. ) ;
#9049=ADVANCED_FACE ( 'NONE', ( #12751 ), #4892, .F. ) ;
#9051=EDGE_CURVE ( 'NONE', #5002, #6209, #4690, .T. ) ;
#9055=CARTESIAN_POINT ( 'NONE',  ( 58.74999981404331351, 1.953940384112647033, -0.08513245267633837154 ) ) ;
#9059=ORIENTED_EDGE ( 'NONE', *, *, #19326, .T. ) ;
#9060=DIRECTION ( 'NONE',  ( 0.000000000000000000, 0.000000000000000000, 1.000000000000000000 ) ) ;
#9064=AXIS2_PLACEMENT_3D ( 'NONE', #19656, #24529, #17412 ) ;
#9067=CARTESIAN_POINT ( 'NONE',  ( 58.65000000000000568, 1.571497941946485177, 1.022750809562084306 ) ) ;
#9069=CARTESIAN_POINT ( 'NONE',  ( 61.01567056675808942, 0.5566600462024857698, 1.706616170210761618 ) ) ;
#9073=DIRECTION ( 'NONE',  ( 1.000000000000000000, 1.047444401652940007E-14, 0.000000000000000000 ) ) ;
#9081=CARTESIAN_POINT ( 'NONE',  ( 50.56924445453659445, -0.1015585333197664281, 0.8011027422770335971 ) ) ;
#9088=CARTESIAN_POINT ( 'NONE',  ( 58.75000000000002132, 6.153735859711025284E-13, 3.111507638930570854E-58 ) ) ;
#9093=ADVANCED_FACE ( 'NONE', ( #28964 ), #18472, .F. ) ;
#9094=CARTESIAN_POINT ( 'NONE',  ( 58.75000000000004263, -2.008165151418373373, -0.5380862305909229759 ) ) ;
#9097=CARTESIAN_POINT ( 'NONE',  ( 51.22715433738865443, 0.9941391646906797552, -1.410349289489640334 ) ) ;
#9106=DIRECTION ( 'NONE',  ( 0.000000000000000000, 0.000000000000000000, 1.000000000000000000 ) ) ;
#9108=B_SPLINE_CURVE_WITH_KNOTS ( 'NONE', 3,
 ( #12752, #13361, #8171, #22429 ),
 .UNSPECIFIED., .F., .F.,
 ( 4, 4 ),
 ( 0.0001543670095910070058, 0.0003084486524517391867 ),
 .UNSPECIFIED. ) ;
#9111=CARTESIAN_POINT ( 'NONE',  ( 58.74999981404331351, 1.441842230226507926, 1.321446761054005492 ) ) ;
#9112=CIRCLE ( 'NONE', #18729, 0.1500000000000000777 ) ;
#9115=CARTESIAN_POINT ( 'NONE',  ( 58.75000000000002132, -0.6121634413828838106, -1.877732920580933218 ) ) ;
#9116=CARTESIAN_POINT ( 'NONE',  ( 58.72200624034183392, -0.9564954546387592904, 1.612834625125136201 ) ) ;
#9128=ORIENTED_EDGE ( 'NONE', *, *, #25696, .T. ) ;
#9131=ORIENTED_EDGE ( 'NONE', *, *, #28044, .F. ) ;
#9140=ORIENTED_EDGE ( 'NONE', *, *, #13911, .T. ) ;
#9143=ORIENTED_EDGE ( 'NONE', *, *, #14286, .F. ) ;
#9152=CARTESIAN_POINT ( 'NONE',  ( 50.25000000000003553, -1.470078920827295965, -1.320078920827526758 ) ) ;
#9172=CARTESIAN_POINT ( 'NONE',  ( 58.73379417893112731, 0.8670685180646029444, -1.662624490946997602 ) ) ;
#9173=CARTESIAN_POINT ( 'NONE',  ( 58.73371041428941908, -1.381461519772573698, 1.267950628961816095 ) ) ;
#9180=CARTESIAN_POINT ( 'NONE',  ( 58.65000000000003411, -1.394635017527501297, 1.253243060178016455 ) ) ;
#9189=EDGE_CURVE ( 'NONE', #7404, #30905, #9600, .T. ) ;
#9195=CARTESIAN_POINT ( 'NONE',  ( 58.75000000000002842, -1.039502773796102897, -1.800471618824325493 ) ) ;
#9204=EDGE_LOOP ( 'NONE', ( #19772, #27743, #11329, #4528 ) ) ;
#9206=CARTESIAN_POINT ( 'NONE',  ( 61.25000000000004263, -1.499837071477705619, -1.323060376181415254 ) ) ;
#9211=ORIENTED_EDGE ( 'NONE', *, *, #19459, .T. ) ;
#9213=CARTESIAN_POINT ( 'NONE',  ( 51.31572262954152563, 0.7526089581382734428, -1.996089927833914146 ) ) ;
#9215=EDGE_CURVE ( 'NONE', #7041, #23567, #17560, .T. ) ;
#9219=CARTESIAN_POINT ( 'NONE',  ( 58.65263613458530045, 1.873885868625531304, -0.06672978513348816476 ) ) ;
#9222=ORIENTED_EDGE ( 'NONE', *, *, #26286, .T. ) ;
#9225=CIRCLE ( 'NONE', #26896, 0.1500000000000001887 ) ;
#9226=EDGE_CURVE ( 'NONE', #24848, #17885, #19583, .T. ) ;
#9231=CYLINDRICAL_SURFACE ( 'NONE', #2825, 2.000000000000000000 ) ;
#9232=LINE ( 'NONE', #18894, #6463 ) ;
#9235=CARTESIAN_POINT ( 'NONE',  ( 50.25000000000000000, 1.470078920828055358, -1.470078920826818125 ) ) ;
#9236=EDGE_CURVE ( 'NONE', #2824, #4687, #27346, .T. ) ;
#9237=CIRCLE ( 'NONE', #18850, 0.1500000000000003830 ) ;
#9241=CARTESIAN_POINT ( 'NONE',  ( 58.74999999305997989, -1.683452862812675921, -0.9423072185564655978 ) ) ;
#9245=CARTESIAN_POINT ( 'NONE',  ( 51.31802667458096323, -1.005866567096536546, -1.281163073955422504 ) ) ;
#9248=CARTESIAN_POINT ( 'NONE',  ( 58.75000000000002132, 6.153735859711025284E-13, 3.111507638930570854E-58 ) ) ;
#9249=ORIENTED_EDGE ( 'NONE', *, *, #5312, .T. ) ;
#9251=CARTESIAN_POINT ( 'NONE',  ( 61.09423418604053069, -0.6373668173463740150, -1.895722432252557432 ) ) ;
#9254=EDGE_LOOP ( 'NONE', ( #13991, #6101, #25540, #12963 ) ) ;
#9257=CARTESIAN_POINT ( 'NONE',  ( 50.25000000000002842, -1.039502773796191937, -1.800471618824325493 ) ) ;
#9258=SHAPE_REPRESENTATION ( 'Eraser Holder', ( #9018 ), #3487 ) ;
#9261=LINE ( 'NONE', #1795, #15581 ) ;
#9262=DIRECTION ( 'NONE',  ( 1.000000000000000000, 1.047444401652940007E-14, 0.000000000000000000 ) ) ;
#9263=EDGE_CURVE ( 'NONE', #8618, #29589, #3385, .T. ) ;
#9267=CARTESIAN_POINT ( 'NONE',  ( 61.25000000000000000, 1.895722432252729739, 0.6373668173479285493 ) ) ;
#9275=CARTESIAN_POINT ( 'NONE',  ( 58.65000000000004121, -1.827485639842249876, 0.4207625006690558500 ) ) ;
#9277=CARTESIAN_POINT ( 'NONE',  ( 58.74160516400041132, -0.8556415768458849325, 1.668397168087476956 ) ) ;
#9278=ADVANCED_FACE ( 'NONE', ( #6891 ), #2289, .F. ) ;
#9284=AXIS2_PLACEMENT_3D ( 'NONE', #15376, #20777, #22691 ) ;
#9289=DIRECTION ( 'NONE',  ( 1.000000000000000000, 1.047444401652940007E-14, 0.000000000000000000 ) ) ;
#9291=ORIENTED_EDGE ( 'NONE', *, *, #17860, .T. ) ;
#9298=ORIENTED_EDGE ( 'NONE', *, *, #5393, .T. ) ;
#9301=CARTESIAN_POINT ( 'NONE',  ( 58.65266784251154775, 1.827264058875769370, -0.4207260278625468697 ) ) ;
#9309=AXIS2_PLACEMENT_3D ( 'NONE', #4525, #13693, #21000 ) ;
#9310=DIRECTION ( 'NONE',  ( 0.000000000000000000, 0.000000000000000000, 1.000000000000000000 ) ) ;
#9312=ADVANCED_FACE ( 'NONE', ( #29659 ), #7985, .F. ) ;
#9315=CARTESIAN_POINT ( 'NONE',  ( 60.81555826527926456, -0.6499999999993623101, -1.489337100860648855 ) ) ;
#9320=ORIENTED_EDGE ( 'NONE', *, *, #2508, .F. ) ;
#9322=AXIS2_PLACEMENT_3D ( 'NONE', #27528, #25171, #3486 ) ;
#9323=CARTESIAN_POINT ( 'NONE',  ( 58.75000000000000000, 2.008165151418601191, 0.5380862305919300592 ) ) ;
#9324=DIRECTION ( 'NONE',  ( 1.000000000000000000, 1.047444401652940007E-14, 0.000000000000000000 ) ) ;
#9325=ORIENTED_EDGE ( 'NONE', *, *, #29176, .T. ) ;
#9326=PLANE ( 'NONE',  #23995 ) ;
#9327=DIRECTION ( 'NONE',  ( 1.000000000000000000, 1.047444401652940007E-14, 0.000000000000000000 ) ) ;
#9329=CARTESIAN_POINT ( 'NONE',  ( 58.65000000000003411, -1.372267738820216021, 1.278133834460509100 ) ) ;
#9337=EDGE_CURVE ( 'NONE', #24348, #12125, #26625, .T. ) ;
#9347=CARTESIAN_POINT ( 'NONE',  ( 58.66054497608038076, -0.4999999999994944599, -1.807104036850091688 ) ) ;
#9350=AXIS2_PLACEMENT_3D ( 'NONE', #23164, #8873, #3527 ) ;
#9351=LINE ( 'NONE', #11723, #3409 ) ;
#9356=ORIENTED_EDGE ( 'NONE', *, *, #5617, .F. ) ;
#9357=CARTESIAN_POINT ( 'NONE',  ( 58.75000000000004974, -1.834410884275049947, 0.3880228184668815250 ) ) ;
#9363=TOROIDAL_SURFACE ( 'NONE', #29068, 1.975000000000001865, 0.1000000000000000056 ) ;
#9364=ORIENTED_EDGE ( 'NONE', *, *, #27794, .T. ) ;
#9371=FACE_OUTER_BOUND ( 'NONE', #26619, .T. ) ;
#9382=CARTESIAN_POINT ( 'NONE',  ( 58.75000000000002132, 6.153735859711025284E-13, 3.111507638930570854E-58 ) ) ;
#9386=EDGE_CURVE ( 'NONE', #19192, #1382, #11999, .T. ) ;
#9391=AXIS2_PLACEMENT_3D ( 'NONE', #16868, #31099, #1806 ) ;
#9402=CARTESIAN_POINT ( 'NONE',  ( 58.65000000000001990, 6.143261415694495821E-13, 3.111507638930570854E-58 ) ) ;
#9424=AXIS2_PLACEMENT_3D ( 'NONE', #21755, #23650, #11606 ) ;
#9425=CARTESIAN_POINT ( 'NONE',  ( 52.06628335902946247, -0.5434431642975677823, -1.718465885608440713 ) ) ;
#9428=CARTESIAN_POINT ( 'NONE',  ( 58.65000000000002700, -0.8495817349395322626, -1.671477153794241444 ) ) ;
#9431=DIRECTION ( 'NONE',  ( 0.000000000000000000, 0.000000000000000000, 1.000000000000000000 ) ) ;
#9435=CARTESIAN_POINT ( 'NONE',  ( 58.75000000000002132, -0.5933779550749339604, -1.867062706145875772 ) ) ;
#9436=DIRECTION ( 'NONE',  ( -1.000000000000000000, -1.047444401652940007E-14, 0.000000000000000000 ) ) ;
#9438=CARTESIAN_POINT ( 'NONE',  ( 58.73794315689227830, -0.4999999999993849364, 1.843373610711628974 ) ) ;
#9440=CONICAL_SURFACE ( 'NONE', #20065, 1.487500000000000933, 0.7853981633974481680 ) ;
#9460=ORIENTED_EDGE ( 'NONE', *, *, #26462, .F. ) ;
#9470=CARTESIAN_POINT ( 'NONE',  ( 58.75000000000002132, 6.153735859711025284E-13, 3.111507638930570854E-58 ) ) ;
#9472=CARTESIAN_POINT ( 'NONE',  ( 61.25000000000003553, -1.106298139389688462, -1.666164585742599513 ) ) ;
#9478=AXIS2_PLACEMENT_3D ( 'NONE', #22719, #852, #20193 ) ;
#9485=DIRECTION ( 'NONE',  ( 1.000000000000000000, 1.047444401652940007E-14, 0.000000000000000000 ) ) ;
#9496=CARTESIAN_POINT ( 'NONE',  ( 58.74999981196284438, 1.050519579373341506, -1.649561145037804266 ) ) ;
#9498=ORIENTED_EDGE ( 'NONE', *, *, #25165, .T. ) ;
#9500=CARTESIAN_POINT ( 'NONE',  ( 50.78793970012935688, -0.4223115601891289650, 0.9680023493207207119 ) ) ;
#9507=EDGE_LOOP ( 'NONE', ( #297, #8512, #21483, #28222, #1135, #1598, #23229 ) ) ;
#9511=DIRECTION ( 'NONE',  ( 1.000000000000000000, 1.047444401652940007E-14, 0.000000000000000000 ) ) ;
#9513=CARTESIAN_POINT ( 'NONE',  ( 50.56948141424500420, 0.1019060742265078534, -1.190674082256531818 ) ) ;
#9515=CARTESIAN_POINT ( 'NONE',  ( 51.25000000000002842, -1.099999999999462963, 1.196087371390569087 ) ) ;
#9520=VECTOR ( 'NONE', #14728, 1000.000000000000000 ) ;
#9533=CARTESIAN_POINT ( 'NONE',  ( 58.72204580543434105, -1.805265037611284873, 0.5070891929461229797 ) ) ;
#9541=CARTESIAN_POINT ( 'NONE',  ( 51.43640408064043612, -0.9729063086537432792, -1.446762274037361573 ) ) ;
#9546=ORIENTED_EDGE ( 'NONE', *, *, #14078, .F. ) ;
#9547=CARTESIAN_POINT ( 'NONE',  ( 58.74999981196283017, 1.953821646385494715, 0.08499607039126413910 ) ) ;
#9578=CARTESIAN_POINT ( 'NONE',  ( 60.75000000000001421, 0.5000000000006329381, -1.554802467931481580 ) ) ;
#9594=CARTESIAN_POINT ( 'NONE',  ( 52.20711756518984004, -0.4999999999994533817, -1.807104036850122109 ) ) ;
#9596=CARTESIAN_POINT ( 'NONE',  ( 58.65266784251154064, -0.8793208749730293539, -1.656109637135622981 ) ) ;
#9600=LINE ( 'NONE', #21471, #17050 ) ;
#9601=VECTOR ( 'NONE', #9327, 1000.000000000000000 ) ;
#9603=CARTESIAN_POINT ( 'NONE',  ( 58.74999999999980815, -0.8495817349408062436, 1.671477153793593740 ) ) ;
#9610=ORIENTED_EDGE ( 'NONE', *, *, #13915, .T. ) ;
#9611=ADVANCED_FACE ( 'NONE', ( #25997 ), #11501, .T. ) ;
#9613=CARTESIAN_POINT ( 'NONE',  ( 58.71182503183384682, 0.5000000000006149525, -1.820794158165981003 ) ) ;
#9614=EDGE_LOOP ( 'NONE', ( #6709, #21412, #26340, #7202 ) ) ;
#9625=ORIENTED_EDGE ( 'NONE', *, *, #5209, .T. ) ;
#9630=VECTOR ( 'NONE', #12617, 1000.000000000000000 ) ;
#9632=DIRECTION ( 'NONE',  ( 1.000000000000000000, 1.047444401652940007E-14, 0.000000000000000000 ) ) ;
#9637=B_SPLINE_CURVE_WITH_KNOTS ( 'NONE', 3,
 ( #14416, #2228, #2078, #24089, #28368, #28520, #4457, #31045, #6672, #12064, #26308, #4610, #25981 ),
 .UNSPECIFIED., .F., .F.,
 ( 4, 3, 3, 3, 4 ),
 ( 0.000000000000000000, 3.315084464040651867E-05, 6.626473632996253958E-05, 9.991171812043499688E-05, 0.0001104636331268446688 ),
 .UNSPECIFIED. ) ;
#9647=CARTESIAN_POINT ( 'NONE',  ( 61.25000000000000000, 2.008165151418627836, 0.5380862305919300592 ) ) ;
#9656=DIRECTION ( 'NONE',  ( 9.337490065241209392E-15, -0.8914544820236761646, -0.4531102586345839844 ) ) ;
#9660=CARTESIAN_POINT ( 'NONE',  ( 58.75000018803718405, 0.9251739982205126056, 1.701355787207728509 ) ) ;
#9680=ORIENTED_EDGE ( 'NONE', *, *, #22072, .T. ) ;
#9685=CARTESIAN_POINT ( 'NONE',  ( 50.25000000000000000, 1.666164585743128423, -1.106298139389324975 ) ) ;
#9688=AXIS2_PLACEMENT_3D ( 'NONE', #14059, #6309, #18513 ) ;
#9689=CARTESIAN_POINT ( 'NONE',  ( 51.59739104186229497, -1.010292945602101256, -1.272765950230260623 ) ) ;
#9690=ORIENTED_EDGE ( 'NONE', *, *, #1875, .T. ) ;
#9699=EDGE_CURVE ( 'NONE', #8227, #20392, #20125, .T. ) ;
#9700=EDGE_LOOP ( 'NONE', ( #17536, #25438, #26531, #8843 ) ) ;
#9703=EDGE_CURVE ( 'NONE', #5737, #3048, #9232, .T. ) ;
#9709=DIRECTION ( 'NONE',  ( -8.778969181342580612E-15, 0.8381322357051846916, -0.5454670984320033611 ) ) ;
#9715=EDGE_CURVE ( 'NONE', #585, #7031, #5264, .T. ) ;
#9716=ORIENTED_EDGE ( 'NONE', *, *, #7979, .F. ) ;
#9733=VERTEX_POINT ( 'NONE', #26167 ) ;
#9735=CYLINDRICAL_SURFACE ( 'NONE', #17732, 0.1500000000000000777 ) ;
#9741=CARTESIAN_POINT ( 'NONE',  ( 58.75000018803719826, -0.9251739982198918799, -1.701355787207161852 ) ) ;
#9742=CYLINDRICAL_SURFACE ( 'NONE', #14472, 0.1500000000000001887 ) ;
#9743=CARTESIAN_POINT ( 'NONE',  ( 52.20711756518984714, -0.7499999999994533262, -1.718465885608440713 ) ) ;
#9745=CYLINDRICAL_SURFACE ( 'NONE', #29567, 2.000000000000000000 ) ;
#9746=CARTESIAN_POINT ( 'NONE',  ( 51.50435016707358926, 0.9265794315412880788, 1.339215852266871565 ) ) ;
#9757=ORIENTED_EDGE ( 'NONE', *, *, #12510, .T. ) ;
#9764=CARTESIAN_POINT ( 'NONE',  ( 58.66107449606931823, -1.640741681269791030, 0.9081280691417603634 ) ) ;
#9766=ORIENTED_EDGE ( 'NONE', *, *, #28456, .T. ) ;
#9773=CARTESIAN_POINT ( 'NONE',  ( 58.64999999999999858, 1.760622601997808845, -0.8948927608024527247 ) ) ;
#9774=AXIS2_PLACEMENT_3D ( 'NONE', #10131, #19796, #29430 ) ;
#9775=CYLINDRICAL_SURFACE ( 'NONE', #11942, 0.2500000000000000000 ) ;
#9776=ADVANCED_FACE ( 'NONE', ( #7938 ), #12360, .F. ) ;
#9783=ORIENTED_EDGE ( 'NONE', *, *, #23524, .T. ) ;
#9787=CARTESIAN_POINT ( 'NONE',  ( 58.74154451056412540, 1.017012227666128643, -1.575232816092163590 ) ) ;
#9791=FACE_OUTER_BOUND ( 'NONE', #24086, .T. ) ;
#9805=DIRECTION ( 'NONE',  ( 1.000000000000000000, 1.047444401652940007E-14, 0.000000000000000000 ) ) ;
#9807=( BOUNDED_SURFACE ( )  B_SPLINE_SURFACE ( 3, 2, ( 
 ( #29782, #8098, #3650 ),
 ( #13285, #13148, #17765 ),
 ( #10771, #27406, #20454 ),
 ( #30079, #15366, #25016 ),
 ( #978, #8398, #3346 ),
 ( #22682, #10630, #29936 ),
 ( #8245, #28503, #18707 ),
 ( #16319, #4268, #20915 ),
 ( #21555, #6656, #3962 ),
 ( #13914, #21087, #25962 ) ),
 .UNSPECIFIED., .F., .F., .T. ) 
 B_SPLINE_SURFACE_WITH_KNOTS ( ( 4, 2, 2, 2, 4 ),
 ( 3, 3 ),
 ( 0.0001706658715699975362, 0.0002229276920781214167, 0.0002751895125862452701, 0.0003274513330943691234, 0.0003797131536024929768 ),
 ( 0.000000000000000000, 1.000000000000000000 ),
 .UNSPECIFIED. ) 
 GEOMETRIC_REPRESENTATION_ITEM ( )  RATIONAL_B_SPLINE_SURFACE ( (
 ( 1.000000000000000000, 0.7071067811873480435, 1.000000000000000000),
 ( 1.000000000000000000, 0.7375607040708425099, 1.000000000000000000),
 ( 1.000000000000000000, 0.7730431127430062999, 1.000000000000000000),
 ( 1.000000000000000000, 0.8321012486976929745, 1.000000000000000000),
 ( 1.000000000000000000, 0.8541932017391521414, 1.000000000000000000),
 ( 1.000000000000000000, 0.8545723906038292794, 1.000000000000000000),
 ( 1.000000000000000000, 0.8327032135030432158, 1.000000000000000000),
 ( 1.000000000000000000, 0.7734559727055867473, 1.000000000000000000),
 ( 1.000000000000000000, 0.7377766653993185209, 1.000000000000000000),
 ( 1.000000000000000000, 0.7071067811865511255, 1.000000000000000000) ) ) 
 REPRESENTATION_ITEM ( '' )  SURFACE ( )  );
#9813=AXIS2_PLACEMENT_3D ( 'NONE', #21885, #12502, #24534 ) ;
#9814=CARTESIAN_POINT ( 'NONE',  ( 58.75000000000003553, -1.791164585742988757, 0.8897917884442223535 ) ) ;
#9815=DIRECTION ( 'NONE',  ( -1.000000000000000000, -1.047444401652940007E-14, -0.000000000000000000 ) ) ;
#9816=CARTESIAN_POINT ( 'NONE',  ( 58.65000000000000568, 1.077297519405725046, -1.655311165516502925 ) ) ;
#9818=CARTESIAN_POINT ( 'NONE',  ( 58.74999999999981526, -1.782657835994365003, 0.5811678240970542531 ) ) ;
#9822=CARTESIAN_POINT ( 'NONE',  ( 58.72219294808299139, -0.4999999999993851585, -1.828782891498922369 ) ) ;
#9825=ORIENTED_EDGE ( 'NONE', *, *, #22984, .F. ) ;
#9827=VERTEX_POINT ( 'NONE', #24364 ) ;
#9837=CARTESIAN_POINT ( 'NONE',  ( 58.65000000000003411, -1.394635017527474430, -1.253243060178046875 ) ) ;
#9848=CARTESIAN_POINT ( 'NONE',  ( 58.64999999999992752, -1.932246131436387682, -0.4087173687853297710 ) ) ;
#9852=CARTESIAN_POINT ( 'NONE',  ( 58.75000000000002132, 6.153735859711025284E-13, 3.111507638930570854E-58 ) ) ;
#9855=DIRECTION ( 'NONE',  ( 1.000000000000000000, 1.047444401652940007E-14, 0.000000000000000000 ) ) ;
#9856=VERTEX_POINT ( 'NONE', #5050 ) ;
#9865=DIRECTION ( 'NONE',  ( 0.7071067811865404673, 0.7071067811865546782, 0.000000000000000000 ) ) ;
#9871=ORIENTED_EDGE ( 'NONE', *, *, #12025, .T. ) ;
#9872=ORIENTED_EDGE ( 'NONE', *, *, #13093, .F. ) ;
#9886=CARTESIAN_POINT ( 'NONE',  ( 50.56924445453658024, 0.1015585333208254837, -0.8011027422770338191 ) ) ;
#9888=DIRECTION ( 'NONE',  ( -1.000000000000000000, -1.047444401652940007E-14, -0.000000000000000000 ) ) ;
#9892=CARTESIAN_POINT ( 'NONE',  ( 58.65000000000001990, 6.143261415694495821E-13, 3.111507638930570854E-58 ) ) ;
#9893=CARTESIAN_POINT ( 'NONE',  ( 51.31802667458094902, 1.005866567097610575, 1.281163073955430720 ) ) ;
#9895=DIRECTION ( 'NONE',  ( 0.000000000000000000, 0.000000000000000000, 1.000000000000000000 ) ) ;
#9900=AXIS2_PLACEMENT_3D ( 'NONE', #16197, #28056, #25845 ) ;
#9907=ORIENTED_EDGE ( 'NONE', *, *, #26129, .F. ) ;
#9912=AXIS2_PLACEMENT_3D ( 'NONE', #9382, #16508, #23948 ) ;
#9913=DIRECTION ( 'NONE',  ( 0.000000000000000000, 0.000000000000000000, 1.000000000000000000 ) ) ;
#9928=DIRECTION ( 'NONE',  ( -0.000000000000000000, -0.000000000000000000, -1.000000000000000000 ) ) ;
#9929=DIRECTION ( 'NONE',  ( 0.000000000000000000, 0.000000000000000000, 1.000000000000000000 ) ) ;
#9933=CIRCLE ( 'NONE', #31150, 0.1500000000000001887 ) ;
#9939=ORIENTED_EDGE ( 'NONE', *, *, #25683, .T. ) ;
#9944=EDGE_CURVE ( 'NONE', #25442, #7031, #2529, .T. ) ;
#9946=LINE ( 'NONE', #29260, #3184 ) ;
#9949=ORIENTED_EDGE ( 'NONE', *, *, #24930, .F. ) ;
#9950=AXIS2_PLACEMENT_3D ( 'NONE', #30254, #18242, #3968 ) ;
#9953=AXIS2_PLACEMENT_3D ( 'NONE', #3351, #13289, #25020 ) ;
#9967=( BOUNDED_CURVE ( )  B_SPLINE_CURVE ( 3, ( #6482, #16142, #13739, #30702 ),
 .UNSPECIFIED., .F., .T. ) 
 B_SPLINE_CURVE_WITH_KNOTS ( ( 4, 4 ),
 ( 1.454199501120271742, 2.189070931013919807 ),
 .UNSPECIFIED. ) 
 CURVE ( )  GEOMETRIC_REPRESENTATION_ITEM ( )  RATIONAL_B_SPLINE_CURVE ( ( 1.000000000000000000, 0.9555010429016488338, 0.9555010429016488338, 1.000000000000000000 ) ) 
 REPRESENTATION_ITEM ( '' )  );
#9973=CIRCLE ( 'NONE', #27166, 0.1500000000000001887 ) ;
#9978=CARTESIAN_POINT ( 'NONE',  ( 58.65000000000001279, 0.5811678240972314446, 1.782657835995122175 ) ) ;
#9983=CARTESIAN_POINT ( 'NONE',  ( 58.75000000000004263, -1.877732920580553300, 0.6121634413821477327 ) ) ;
#9987=DIRECTION ( 'NONE',  ( 0.000000000000000000, 0.000000000000000000, 1.000000000000000000 ) ) ;
#9994=CARTESIAN_POINT ( 'NONE',  ( 51.45655683570191741, -0.9591657938390835136, -1.468576096419531574 ) ) ;
#9998=FACE_OUTER_BOUND ( 'NONE', #12217, .T. ) ;
#10001=VERTEX_POINT ( 'NONE', #29273 ) ;
#10003=AXIS2_PLACEMENT_3D ( 'NONE', #8684, #6317, #4248 ) ;
#10005=CARTESIAN_POINT ( 'NONE',  ( 58.72427158855720108, -1.357477749119001098, -1.293556822994985422 ) ) ;
#10006=( BOUNDED_SURFACE ( )  B_SPLINE_SURFACE ( 3, 2, ( 
 ( #14219, #10104, #3283 ),
 ( #12928, #10718, #29553 ),
 ( #2978, #24958, #7717 ),
 ( #22154, #15642, #22450 ),
 ( #27198, #25127, #22620 ),
 ( #8192, #19922, #22778 ) ),
 .UNSPECIFIED., .F., .F., .F. ) 
 B_SPLINE_SURFACE_WITH_KNOTS ( ( 4, 2, 4 ),
 ( 3, 3 ),
 ( -5.854691731421723944E-18, 0.0002091250881941168597, 0.0004182501763882395742 ),
 ( 0.000000000000000000, 1.000000000000000000 ),
 .UNSPECIFIED. ) 
 GEOMETRIC_REPRESENTATION_ITEM ( )  RATIONAL_B_SPLINE_SURFACE ( (
 ( 1.000000000000000000, 0.8366600265340757847, 1.000000000000000000),
 ( 1.000000000000000000, 0.8366252886217447893, 1.000000000000000000),
 ( 1.000000000000000000, 0.8275698663184574144, 1.000000000000000000),
 ( 1.000000000000000000, 0.7855086314083459254, 1.000000000000000000),
 ( 1.000000000000000000, 0.7518972359450074583, 1.000000000000000000),
 ( 1.000000000000000000, 0.7071067811865494601, 1.000000000000000000) ) ) 
 REPRESENTATION_ITEM ( '' )  SURFACE ( )  );
#10008=VERTEX_POINT ( 'NONE', #27359 ) ;
#10011=DIRECTION ( 'NONE',  ( 0.000000000000000000, 0.000000000000000000, 1.000000000000000000 ) ) ;
#10015=DIRECTION ( 'NONE',  ( 0.000000000000000000, 0.000000000000000000, 1.000000000000000000 ) ) ;
#10017=CARTESIAN_POINT ( 'NONE',  ( 51.13989201884562874, -0.9305404255926473800, -1.499649012356343958 ) ) ;
#10020=CARTESIAN_POINT ( 'NONE',  ( 61.25000000000004263, -1.996089927833272881, -0.1249999999999982098 ) ) ;
#10022=DIRECTION ( 'NONE',  ( 1.000000000000000000, 1.047444401652940007E-14, 0.000000000000000000 ) ) ;
#10028=EDGE_CURVE ( 'NONE', #31243, #26954, #1889, .T. ) ;
#10034=CARTESIAN_POINT ( 'NONE',  ( 51.36685778188466855, 1.002608958138272444, 1.584424273060086152 ) ) ;
#10043=DIRECTION ( 'NONE',  ( 0.000000000000000000, 0.000000000000000000, 1.000000000000000000 ) ) ;
#10054=LINE ( 'NONE', #19724, #31092 ) ;
#10061=AXIS2_PLACEMENT_3D ( 'NONE', #27048, #19337, #5532 ) ;
#10070=ORIENTED_EDGE ( 'NONE', *, *, #7666, .T. ) ;
#10071=CARTESIAN_POINT ( 'NONE',  ( 51.25000000000002842, -1.099999999999462963, -1.996089927833914146 ) ) ;
#10084=VECTOR ( 'NONE', #29182, 1000.000000000000000 ) ;
#10086=CYLINDRICAL_SURFACE ( 'NONE', #1333, 0.1500000000000001887 ) ;
#10087=CARTESIAN_POINT ( 'NONE',  ( 58.65000000000001990, 6.143261415694495821E-13, 3.111507638930570854E-58 ) ) ;
#10104=CARTESIAN_POINT ( 'NONE',  ( 60.75000000000002842, -0.4999999999993641198, -1.554802467931445609 ) ) ;
#10118=CARTESIAN_POINT ( 'NONE',  ( 58.65000000000000568, 1.253243060177670287, 1.394635017528978782 ) ) ;
#10120=EDGE_CURVE ( 'NONE', #11926, #21490, #24189, .T. ) ;
#10122=DIRECTION ( 'NONE',  ( 0.000000000000000000, 0.000000000000000000, 1.000000000000000000 ) ) ;
#10124=DIRECTION ( 'NONE',  ( 0.000000000000000000, 0.000000000000000000, 1.000000000000000000 ) ) ;
#10127=CARTESIAN_POINT ( 'NONE',  ( 51.23644008536122385, 1.080112125196981854, 1.214076932077872817 ) ) ;
#10131=CARTESIAN_POINT ( 'NONE',  ( 58.75000000000000711, 1.039502773797200019, -1.800471618823823450 ) ) ;
#10133=UNCERTAINTY_MEASURE_WITH_UNIT (LENGTH_MEASURE( 1.000000000000000082E-05 ), #18108, 'distance_accuracy_value', 'NONE');
#10140=CARTESIAN_POINT ( 'NONE',  ( 52.20711756518984714, -0.6499999999994534594, -1.489337100860648189 ) ) ;
#10141=DIRECTION ( 'NONE',  ( 1.000000000000000000, 1.047444401652940007E-14, 0.000000000000000000 ) ) ;
#10162=CARTESIAN_POINT ( 'NONE',  ( 51.25000000000001421, 1.100000000000537215, -1.196087371390568643 ) ) ;
#10174=B_SPLINE_CURVE_WITH_KNOTS ( 'NONE', 3,
 ( #20875, #30504, #18500, #16278 ),
 .UNSPECIFIED., .F., .F.,
 ( 4, 4 ),
 ( 0.0001956043251250877066, 0.0003834565248886559865 ),
 .UNSPECIFIED. ) ;
#10184=CARTESIAN_POINT ( 'NONE',  ( 58.75000000000003553, -1.972190280207336555, -0.1053114364790862928 ) ) ;
#10186=VERTEX_POINT ( 'NONE', #7025 ) ;
#10200=CARTESIAN_POINT ( 'NONE',  ( 58.64999999999999858, 1.874116925335308714, 0.06656272211392090521 ) ) ;
#10201=CARTESIAN_POINT ( 'NONE',  ( 58.72200624034157812, 1.341335979948039547, -1.310319377727088064 ) ) ;
#10205=VERTEX_POINT ( 'NONE', #26478 ) ;
#10208=DIRECTION ( 'NONE',  ( 0.000000000000000000, 0.000000000000000000, 1.000000000000000000 ) ) ;
#10211=CARTESIAN_POINT ( 'NONE',  ( 51.45655683570189609, 0.9591657938401613182, -1.611094652690528317 ) ) ;
#10213=EDGE_CURVE ( 'NONE', #24355, #28012, #11440, .T. ) ;
#10214=EDGE_LOOP ( 'NONE', ( #10779, #10620, #8604, #1718 ) ) ;
#10218=VERTEX_POINT ( 'NONE', #21761 ) ;
#10230=CARTESIAN_POINT ( 'NONE',  ( 58.64999999999999858, 1.394635017528131904, 1.253243060178682367 ) ) ;
#10231=DIRECTION ( 'NONE',  ( 1.000000000000000000, 1.047444401652940007E-14, 0.000000000000000000 ) ) ;
#10232=FACE_OUTER_BOUND ( 'NONE', #20851, .T. ) ;
#10233=PLANE ( 'NONE',  #4433 ) ;
#10251=DIRECTION ( 'NONE',  ( -0.5633368246415186853, 0.8262273428075416204, 0.000000000000000000 ) ) ;
#10252=EDGE_CURVE ( 'NONE', #12009, #19299, #7775, .T. ) ;
#10261=CARTESIAN_POINT ( 'NONE',  ( 58.64999999999999858, 1.571497941947157750, -1.022750809561051133 ) ) ;
#10264=CIRCLE ( 'NONE', #28978, 0.1000000000000001998 ) ;
#10273=B_SPLINE_CURVE_WITH_KNOTS ( 'NONE', 3,
 ( #28345, #6651, #16314, #25958, #11085, #13908 ),
 .UNSPECIFIED., .F., .F.,
 ( 4, 2, 4 ),
 ( 0.000000000000000000, 0.0001000270069603067982, 0.0002000540139206135964 ),
 .UNSPECIFIED. ) ;
#10280=DIRECTION ( 'NONE',  ( 1.000000000000000000, 1.047444401652940007E-14, -0.000000000000000000 ) ) ;
#10289=CARTESIAN_POINT ( 'NONE',  ( 51.84831113588973039, 0.6920605891666480325, 1.653603923793167674 ) ) ;
#10305=FACE_OUTER_BOUND ( 'NONE', #17970, .T. ) ;
#10313=ORIENTED_EDGE ( 'NONE', *, *, #11746, .T. ) ;
#10314=DIRECTION ( 'NONE',  ( 0.000000000000000000, 0.000000000000000000, 1.000000000000000000 ) ) ;
#10320=ORIENTED_EDGE ( 'NONE', *, *, #1505, .T. ) ;
#10323=EDGE_CURVE ( 'NONE', #23389, #203, #25305, .T. ) ;
#10339=CARTESIAN_POINT ( 'NONE',  ( 51.84831113588968066, 0.6920605891666815612, -1.653603923793075081 ) ) ;
#10346=CARTESIAN_POINT ( 'NONE',  ( 58.65000000000002700, -1.022750809560422969, 1.571497941946552679 ) ) ;
#10348=CARTESIAN_POINT ( 'NONE',  ( 51.43900111557092458, 0.9711356030203728285, 1.449573366541679009 ) ) ;
#10350=CARTESIAN_POINT ( 'NONE',  ( 58.75000000000000711, 1.457266603154988793, -1.320165430232766557 ) ) ;
#10357=ORIENTED_EDGE ( 'NONE', *, *, #2823, .F. ) ;
#10358=EDGE_CURVE ( 'NONE', #5946, #10684, #3652, .T. ) ;
#10368=CARTESIAN_POINT ( 'NONE',  ( 58.65000000000000568, 1.469015551797813179, -1.320082690053157037 ) ) ;
#10373=FACE_OUTER_BOUND ( 'NONE', #6671, .T. ) ;
#10376=CIRCLE ( 'NONE', #28067, 0.1500000000000002720 ) ;
#10381=DIRECTION ( 'NONE',  ( 0.000000000000000000, 0.000000000000000000, 1.000000000000000000 ) ) ;
#10388=CARTESIAN_POINT ( 'NONE',  ( 51.55144386500332132, -1.037443573994098811, 1.251214392908860829 ) ) ;
#10391=DIRECTION ( 'NONE',  ( 1.000000000000000000, 1.047444401652940007E-14, 0.000000000000000000 ) ) ;
#10405=EDGE_CURVE ( 'NONE', #4841, #5779, #27127, .T. ) ;
#10409=ORIENTED_EDGE ( 'NONE', *, *, #25059, .T. ) ;
#10410=CARTESIAN_POINT ( 'NONE',  ( 58.65000000000003411, -1.469015551795667784, 1.320082690054176666 ) ) ;
#10416=AXIS2_PLACEMENT_3D ( 'NONE', #14855, #17399, #19791 ) ;
#10417=CARTESIAN_POINT ( 'NONE',  ( 58.72204580543390762, 1.612507782426283898, -0.9570475208907850417 ) ) ;
#10434=VECTOR ( 'NONE', #18471, 1000.000000000000000 ) ;
#10442=PRODUCT_DEFINITION_CONTEXT ( 'detailed design', #17699, 'design' ) ;
#10445=CARTESIAN_POINT ( 'NONE',  ( 58.70362814788261119, -0.4999999999993853805, -1.816403611747765767 ) ) ;
#10452=( BOUNDED_CURVE ( )  B_SPLINE_CURVE ( 3, ( #8397, #18083, #29614, #7942 ),
 .UNSPECIFIED., .F., .T. ) 
 B_SPLINE_CURVE_WITH_KNOTS ( ( 4, 4 ),
 ( 1.033802687944701759, 1.276740478505648202 ),
 .UNSPECIFIED. ) 
 CURVE ( )  GEOMETRIC_REPRESENTATION_ITEM ( )  RATIONAL_B_SPLINE_CURVE ( ( 1.000000000000000000, 0.9950878134350369386, 0.9950878134350369386, 1.000000000000000000 ) ) 
 REPRESENTATION_ITEM ( '' )  );
#10460=CARTESIAN_POINT ( 'NONE',  ( 58.65844932252340982, -1.302247349114548980, -1.349094575298717347 ) ) ;
#10480=CARTESIAN_POINT ( 'NONE',  ( 50.25000000000000000, 1.791164585743128423, -0.8897917884432153812 ) ) ;
#10484=DIRECTION ( 'NONE',  ( 1.000000000000000000, 1.047444401652940007E-14, 0.000000000000000000 ) ) ;
#10490=EDGE_LOOP ( 'NONE', ( #22386, #7243, #12744, #27156 ) ) ;
#10491=CARTESIAN_POINT ( 'NONE',  ( 61.20026580823483187, -0.7453886133000856562, 1.660366360129213348 ) ) ;
#10493=AXIS2_PLACEMENT_3D ( 'NONE', #24619, #7680, #7372 ) ;
#10495=CIRCLE ( 'NONE', #13499, 1.625000000000000222 ) ;
#10498=ORIENTED_EDGE ( 'NONE', *, *, #9263, .F. ) ;
#10504=VECTOR ( 'NONE', #13853, 1000.000000000000000 ) ;
#10507=DIRECTION ( 'NONE',  ( 0.000000000000000000, -6.217248937900896348E-15, 1.000000000000000000 ) ) ;
#10512=VERTEX_POINT ( 'NONE', #11574 ) ;
#10514=CARTESIAN_POINT ( 'NONE',  ( 58.65000000000001279, 0.5811678240991622335, -1.782657835994492679 ) ) ;
#10516=AXIS2_PLACEMENT_3D ( 'NONE', #17252, #12480, #10122 ) ;
#10524=CARTESIAN_POINT ( 'NONE',  ( 51.37191502447495139, 0.9974949139205757653, 1.404479416154130522 ) ) ;
#10526=CARTESIAN_POINT ( 'NONE',  ( 58.64999999999999858, 1.253243060178337087, -1.394635017528379484 ) ) ;
#10528=EDGE_LOOP ( 'NONE', ( #25758, #164, #28817, #24398 ) ) ;
#10547=ORIENTED_EDGE ( 'NONE', *, *, #3219, .T. ) ;
#10562=ORIENTED_EDGE ( 'NONE', *, *, #29291, .T. ) ;
#10565=ORIENTED_EDGE ( 'NONE', *, *, #24895, .T. ) ;
#10570=DIRECTION ( 'NONE',  ( 1.000000000000000000, 1.047444401652940007E-14, 0.000000000000000000 ) ) ;
#10573=VERTEX_POINT ( 'NONE', #9814 ) ;
#10577=DIRECTION ( 'NONE',  ( 0.000000000000000000, 0.000000000000000000, 1.000000000000000000 ) ) ;
#10585=CARTESIAN_POINT ( 'NONE',  ( 58.75000000000002132, -0.5380862305903428844, -2.008165151418244143 ) ) ;
#10586=CARTESIAN_POINT ( 'NONE',  ( 51.45655683570191741, -0.9591657938390818483, 1.468576096419532906 ) ) ;
#10601=FACE_OUTER_BOUND ( 'NONE', #26352, .T. ) ;
#10602=ORIENTED_EDGE ( 'NONE', *, *, #17564, .F. ) ;
#10605=CARTESIAN_POINT ( 'NONE',  ( 58.74999981404334903, -1.321446761053663099, 1.441842230225543808 ) ) ;
#10606=ORIENTED_EDGE ( 'NONE', *, *, #29178, .F. ) ;
#10610=ORIENTED_EDGE ( 'NONE', *, *, #24907, .F. ) ;
#10619=EDGE_CURVE ( 'NONE', #5779, #8227, #23726, .T. ) ;
#10620=ORIENTED_EDGE ( 'NONE', *, *, #26060, .T. ) ;
#10626=EDGE_CURVE ( 'NONE', #19375, #23193, #719, .T. ) ;
#10630=CARTESIAN_POINT ( 'NONE',  ( 58.72200624034177707, -1.805437858155882758, -0.5064713447804831681 ) ) ;
#10631=DIRECTION ( 'NONE',  ( 1.000000000000000000, 1.047444401652940007E-14, 0.000000000000000000 ) ) ;
#10649=LINE ( 'NONE', #27896, #8708 ) ;
#10651=EDGE_LOOP ( 'NONE', ( #17346, #19544, #26356, #16591, #18801, #2311 ) ) ;
#10657=CARTESIAN_POINT ( 'NONE',  ( 58.65000000000004121, -1.782657835994308604, 0.5811678240972268927 ) ) ;
#10671=CARTESIAN_POINT ( 'NONE',  ( 50.59602332238209499, 0.1408342061609078322, 1.212874140286674063 ) ) ;
#10678=ORIENTED_EDGE ( 'NONE', *, *, #14883, .F. ) ;
#10684=VERTEX_POINT ( 'NONE', #12328 ) ;
#10691=B_SPLINE_CURVE_WITH_KNOTS ( 'NONE', 3,
 ( #1484, #16060, #20967, #18437 ),
 .UNSPECIFIED., .F., .F.,
 ( 4, 4 ),
 ( 0.000000000000000000, 6.653267247438212099E-05 ),
 .UNSPECIFIED. ) ;
#10708=CARTESIAN_POINT ( 'NONE',  ( 51.31757909864148104, -1.004435980685438157, -1.391945786376508343 ) ) ;
#10711=CARTESIAN_POINT ( 'NONE',  ( 58.75000000000003553, -1.470078920827915470, 1.470078920827824209 ) ) ;
#10715=DIRECTION ( 'NONE',  ( 0.000000000000000000, 0.000000000000000000, 1.000000000000000000 ) ) ;
#10718=CARTESIAN_POINT ( 'NONE',  ( 60.87107532335728166, -0.5000002988016893912, -1.554802360349110790 ) ) ;
#10721=VERTEX_POINT ( 'NONE', #1091 ) ;
#10725=ORIENTED_EDGE ( 'NONE', *, *, #4429, .F. ) ;
#10728=EDGE_CURVE ( 'NONE', #21568, #22153, #4500, .T. ) ;
#10731=CARTESIAN_POINT ( 'NONE',  ( 51.50435016707358926, -0.9265794315402072767, 1.339215852266877782 ) ) ;
#10746=UNCERTAINTY_MEASURE_WITH_UNIT (LENGTH_MEASURE( 1.000000000000000082E-05 ), #30587, 'distance_accuracy_value', 'NONE');
#10749=CARTESIAN_POINT ( 'NONE',  ( 58.75000000000002842, -1.106298139389714663, -1.666164585742599513 ) ) ;
#10753=ADVANCED_FACE ( 'NONE', ( #30048 ), #25112, .F. ) ;
#10757=CARTESIAN_POINT ( 'NONE',  ( 61.25000000000000711, 1.666164585743243665, -1.106298139389324975 ) ) ;
#10771=CARTESIAN_POINT ( 'NONE',  ( 58.74999981404336324, -1.909395380151198252, -0.4234853497079255624 ) ) ;
#10774=ADVANCED_FACE ( 'NONE', ( #15954 ), #25931, .F. ) ;
#10775=DIRECTION ( 'NONE',  ( 0.000000000000000000, 0.000000000000000000, -1.000000000000000000 ) ) ;
#10779=ORIENTED_EDGE ( 'NONE', *, *, #30590, .T. ) ;
#10792=VERTEX_POINT ( 'NONE', #3080 ) ;
#10793=EDGE_CURVE ( 'NONE', #16714, #7404, #6010, .T. ) ;
#10795=CARTESIAN_POINT ( 'NONE',  ( 58.65000000000000568, 1.590093208333579256, -0.9941784314382211551 ) ) ;
#10799=ORIENTED_EDGE ( 'NONE', *, *, #22427, .T. ) ;
#10800=VERTEX_POINT ( 'NONE', #22559 ) ;
#10810=FACE_OUTER_BOUND ( 'NONE', #12927, .T. ) ;
#10813=CARTESIAN_POINT ( 'NONE',  ( 58.67990267795905623, -0.4999999999993856026, 1.808383001045803073 ) ) ;
#10822=CARTESIAN_POINT ( 'NONE',  ( 52.20711756518983293, 0.6500000000005468070, -1.489337100860647967 ) ) ;
#10831=DIRECTION ( 'NONE',  ( 0.000000000000000000, 0.9507508458639141180, 0.3099561728519886206 ) ) ;
#10836=VERTEX_POINT ( 'NONE', #26733 ) ;
#10838=ORIENTED_EDGE ( 'NONE', *, *, #29178, .T. ) ;
#10849=PLANE ( 'NONE',  #20493 ) ;
#10852=CARTESIAN_POINT ( 'NONE',  ( 58.65000000000001279, 1.371849028670515835, 1.278599783849900806 ) ) ;
#10855=CIRCLE ( 'NONE', #4280, 2.000000000000000000 ) ;
#10861=B_SPLINE_CURVE_WITH_KNOTS ( 'NONE', 3,
 ( #8328, #911, #22766, #20390, #9081, #21299 ),
 .UNSPECIFIED., .F., .F.,
 ( 4, 2, 4 ),
 ( 4.207835982932403546E-19, 0.0001531825249253921327, 0.0003063650498507838318 ),
 .UNSPECIFIED. ) ;
#10865=CARTESIAN_POINT ( 'NONE',  ( 58.75000000000002132, 6.153735859711025284E-13, 3.111507638930570854E-58 ) ) ;
#10869=EDGE_CURVE ( 'NONE', #22739, #26116, #26243, .T. ) ;
#10880=DIRECTION ( 'NONE',  ( -1.000000000000000000, -1.047444401652940007E-14, -0.000000000000000000 ) ) ;
#10887=CYLINDRICAL_SURFACE ( 'NONE', #10912, 0.1499999999999999667 ) ;
#10894=CARTESIAN_POINT ( 'NONE',  ( 58.75000000694010538, -1.928945400590438730, -0.02494613115224967453 ) ) ;
#10896=ORIENTED_EDGE ( 'NONE', *, *, #4817, .T. ) ;
#10899=CARTESIAN_POINT ( 'NONE',  ( 58.65000000000001990, 6.143261415694495821E-13, 3.111507638930570854E-58 ) ) ;
#10900=DIRECTION ( 'NONE',  ( 1.000000000000000000, 1.047444401652940007E-14, 0.000000000000000000 ) ) ;
#10903=AXIS2_PLACEMENT_3D ( 'NONE', #18977, #28625, #13573 ) ;
#10907=EDGE_CURVE ( 'NONE', #10218, #1939, #2977, .T. ) ;
#10908=DIRECTION ( 'NONE',  ( 1.000000000000000000, 1.047444401652940007E-14, 0.000000000000000000 ) ) ;
#10912=AXIS2_PLACEMENT_3D ( 'NONE', #764, #29747, #17570 ) ;
#10916=CARTESIAN_POINT ( 'NONE',  ( 58.75000000000000000, 2.008165151418861427, -0.5380862305899540843 ) ) ;
#10922=FACE_OUTER_BOUND ( 'NONE', #22457, .T. ) ;
#10928=LINE ( 'NONE', #12822, #2389 ) ;
#10934=CARTESIAN_POINT ( 'NONE',  ( 58.64999999999999858, 1.782657835995388407, -0.5811678240976838605 ) ) ;
#10938=DIRECTION ( 'NONE',  ( 0.000000000000000000, 0.000000000000000000, 1.000000000000000000 ) ) ;
#10939=CIRCLE ( 'NONE', #4365, 0.1000000000000001027 ) ;
#10944=ORIENTED_EDGE ( 'NONE', *, *, #23598, .T. ) ;
#10958=ORIENTED_EDGE ( 'NONE', *, *, #19574, .F. ) ;
#10961=ORIENTED_EDGE ( 'NONE', *, *, #22698, .F. ) ;
#10963=ADVANCED_FACE ( 'NONE', ( #27921 ), #6235, .T. ) ;
#10965=VECTOR ( 'NONE', #26439, 1000.000000000000000 ) ;
#10971=CARTESIAN_POINT ( 'NONE',  ( 58.66133336607610005, 1.640092727267837169, 0.9092995659222322669 ) ) ;
#10979=EDGE_CURVE ( 'NONE', #22153, #7818, #1249, .T. ) ;
#10983=DIRECTION ( 'NONE',  ( 1.000000000000000000, 1.047444401652940007E-14, 0.000000000000000000 ) ) ;
#10985=CIRCLE ( 'NONE', #28699, 0.1500000000000001887 ) ;
#10995=CARTESIAN_POINT ( 'NONE',  ( 60.97860563121728461, 0.7618031158903413314, -1.436139941719672297 ) ) ;
#11014=CARTESIAN_POINT ( 'NONE',  ( 52.10126625705172643, -0.5195911883732953207, -1.546252172343134390 ) ) ;
#11015=CARTESIAN_POINT ( 'NONE',  ( 51.35663036796566416, -1.000990641333583175, 1.398271059358102475 ) ) ;
#11016=B_SPLINE_CURVE_WITH_KNOTS ( 'NONE', 3,
 ( #14281, #42, #7479, #11753 ),
 .UNSPECIFIED., .F., .F.,
 ( 4, 4 ),
 ( 0.000000000000000000, 0.0001956043251250877066 ),
 .UNSPECIFIED. ) ;
#11037=DIRECTION ( 'NONE',  ( 0.000000000000000000, 0.000000000000000000, -1.000000000000000000 ) ) ;
#11038=EDGE_LOOP ( 'NONE', ( #29754, #5729, #2397, #21667 ) ) ;
#11052=EDGE_CURVE ( 'NONE', #22512, #16027, #6026, .T. ) ;
#11059=CARTESIAN_POINT ( 'NONE',  ( 58.75000018803721247, -1.936004331707231296, -0.04945370822344325595 ) ) ;
#11061=ORIENTED_EDGE ( 'NONE', *, *, #8987, .F. ) ;
#11068=VERTEX_POINT ( 'NONE', #24277 ) ;
#11070=STYLED_ITEM ( 'NONE', ( #20000 ), #27074 ) ;
#11085=CARTESIAN_POINT ( 'NONE',  ( 58.65000000000004121, -1.656030381686081743, -0.8799718970820468167 ) ) ;
#11091=CARTESIAN_POINT ( 'NONE',  ( 51.25000000000001421, 1.100000000000537215, -1.996089927833914146 ) ) ;
#11093=CARTESIAN_POINT ( 'NONE',  ( 58.65000000000000568, 1.022750809562428476, -1.571497941946047083 ) ) ;
#11109=EDGE_LOOP ( 'NONE', ( #20716, #11743, #26902, #16823, #4969 ) ) ;
#11122=FACE_OUTER_BOUND ( 'NONE', #104, .T. ) ;
#11123=CARTESIAN_POINT ( 'NONE',  ( 58.65000000000000568, 1.671477153794444392, 0.8495817349409554575 ) ) ;
#11127=CARTESIAN_POINT ( 'NONE',  ( 58.75000000000003553, -1.470078920827915470, 1.470078920827824209 ) ) ;
#11149=EDGE_CURVE ( 'NONE', #4925, #19375, #21727, .T. ) ;
#11150=CARTESIAN_POINT ( 'NONE',  ( 51.25000000000001421, 1.100000000000537215, -1.996089927833914146 ) ) ;
#11154=( BOUNDED_SURFACE ( )  B_SPLINE_SURFACE ( 3, 2, ( 
 ( #5605, #27289, #30279 ),
 ( #20190, #8589, #6076 ),
 ( #13179, #13032, #8730 ),
 ( #22544, #30113, #1152 ),
 ( #22865, #15727, #25224 ),
 ( #20488, #25055, #12860 ) ),
 .UNSPECIFIED., .F., .F., .F. ) 
 B_SPLINE_SURFACE_WITH_KNOTS ( ( 4, 2, 4 ),
 ( 3, 3 ),
 ( 7.318364664277154930E-19, 0.0002091250881941232294, 0.0004182501763882457541 ),
 ( 0.000000000000000000, 1.000000000000000000 ),
 .UNSPECIFIED. ) 
 GEOMETRIC_REPRESENTATION_ITEM ( )  RATIONAL_B_SPLINE_SURFACE ( (
 ( 1.000000000000000000, 0.8366600265340756737, 1.000000000000000000),
 ( 1.000000000000000000, 0.8366252886216574147, 1.000000000000000000),
 ( 1.000000000000000000, 0.8275698663185694359, 1.000000000000000000),
 ( 1.000000000000000000, 0.7855086314082263543, 1.000000000000000000),
 ( 1.000000000000000000, 0.7518972359451066012, 1.000000000000000000),
 ( 1.000000000000000000, 0.7071067811865354713, 1.000000000000000000) ) ) 
 REPRESENTATION_ITEM ( '' )  SURFACE ( )  );
#11157=CARTESIAN_POINT ( 'NONE',  ( 58.75000000000002132, 6.153735859711025284E-13, 3.111507638930570854E-58 ) ) ;
#11172=CARTESIAN_POINT ( 'NONE',  ( 51.25000000000002842, -0.6499999999994634514, 1.489337100860647967 ) ) ;
#11175=AXIS2_PLACEMENT_3D ( 'NONE', #15308, #2971, #20082 ) ;
#11178=B_SPLINE_CURVE_WITH_KNOTS ( 'NONE', 3,
 ( #16408, #11668, #7078, #19423, #26383, #29069 ),
 .UNSPECIFIED., .F., .F.,
 ( 4, 2, 4 ),
 ( 0.000000000000000000, 0.0001966045864160461917, 0.0003932091728320923833 ),
 .UNSPECIFIED. ) ;
#11179=CARTESIAN_POINT ( 'NONE',  ( 52.06628335902944826, 0.5434431642986583544, 1.718465885608440491 ) ) ;
#11180=VERTEX_POINT ( 'NONE', #2731 ) ;
#11181=EDGE_CURVE ( 'NONE', #2793, #207, #29628, .T. ) ;
#11186=ORIENTED_EDGE ( 'NONE', *, *, #26083, .F. ) ;
#11198=CARTESIAN_POINT ( 'NONE',  ( 58.65838214097839654, 1.802220213626245515, -0.5175938701871466430 ) ) ;
#11204=DIRECTION ( 'NONE',  ( 1.000000000000000000, 1.047444401652940007E-14, -0.000000000000000000 ) ) ;
#11210=LINE ( 'NONE', #21371, #24156 ) ;
#11211=ADVANCED_FACE ( 'NONE', ( #12376 ), #30807, .F. ) ;
#11213=CARTESIAN_POINT ( 'NONE',  ( 58.75000000000000711, 1.655311165516932803, 1.077297519405395310 ) ) ;
#11214=ORIENTED_EDGE ( 'NONE', *, *, #2212, .T. ) ;
#11226=SHAPE_DEFINITION_REPRESENTATION ( #12578, #9258 ) ;
#11233=CARTESIAN_POINT ( 'NONE',  ( 51.21569492700660930, 0.9844681138065065618, 1.555342057744142581 ) ) ;
#11236=DIRECTION ( 'NONE',  ( 1.000000000000000000, 1.047444401652940007E-14, 0.000000000000000000 ) ) ;
#11240=CARTESIAN_POINT ( 'NONE',  ( 61.00000000000003553, -0.8111533433287256845, 1.409596402460999487 ) ) ;
#11242=ORIENTED_EDGE ( 'NONE', *, *, #19388, .T. ) ;
#11247=CARTESIAN_POINT ( 'NONE',  ( 58.75000018803716273, 1.857237022264430326, 0.5488434064270322210 ) ) ;
#11248=CARTESIAN_POINT ( 'NONE',  ( 58.65000000000004121, -1.834410884275050169, 0.3880228184668811364 ) ) ;
#11252=LINE ( 'NONE', #3815, #4224 ) ;
#11262=VERTEX_POINT ( 'NONE', #11248 ) ;
#11266=CARTESIAN_POINT ( 'NONE',  ( 52.13000000000001677, 0.5000000000005460077, -1.718465885608440269 ) ) ;
#11268=CIRCLE ( 'NONE', #1657, 1.975000000000001865 ) ;
#11269=CARTESIAN_POINT ( 'NONE',  ( 60.75000000000002842, -0.7499999999993639532, 1.718465885608440047 ) ) ;
#11280=ORIENTED_EDGE ( 'NONE', *, *, #19388, .F. ) ;
#11286=DIRECTION ( 'NONE',  ( 1.000000000000000000, 1.047444401652940007E-14, 0.000000000000000000 ) ) ;
#11291=DIRECTION ( 'NONE',  ( -1.000000000000000000, -1.047444401652940007E-14, -0.000000000000000000 ) ) ;
#11293=CARTESIAN_POINT ( 'NONE',  ( 58.65000000000001990, 6.143261415694495821E-13, 3.111507638930570854E-58 ) ) ;
#11294=FACE_OUTER_BOUND ( 'NONE', #30994, .T. ) ;
#11300=ORIENTED_EDGE ( 'NONE', *, *, #6050, .F. ) ;
#11303=CARTESIAN_POINT ( 'NONE',  ( 61.25000000000000000, 0.8716090598197026029, -1.626546686965558264 ) ) ;
#11304=EDGE_CURVE ( 'NONE', #15189, #29731, #26267, .T. ) ;
#11305=PLANE ( 'NONE',  #6851 ) ;
#11306=CARTESIAN_POINT ( 'NONE',  ( 58.74154451056414672, 1.258335925860078364, 1.390058629629135956 ) ) ;
#11312=FACE_OUTER_BOUND ( 'NONE', #5685, .T. ) ;
#11316=EDGE_CURVE ( 'NONE', #14207, #4452, #14638, .T. ) ;
#11320=ORIENTED_EDGE ( 'NONE', *, *, #9051, .F. ) ;
#11323=( BOUNDED_SURFACE ( )  B_SPLINE_SURFACE ( 3, 2, ( 
 ( #13045, #20199, #10526 ),
 ( #24608, #20351, #20502 ),
 ( #27604, #12872, #8140 ),
 ( #22556, #545, #12723 ),
 ( #29830, #17813, #17655 ),
 ( #30128, #10201, #15264 ),
 ( #8289, #3077, #27450 ),
 ( #17958, #24911, #15588 ),
 ( #10350, #5764, #5930 ),
 ( #861, #3552, #3398 ) ),
 .UNSPECIFIED., .F., .F., .T. ) 
 B_SPLINE_SURFACE_WITH_KNOTS ( ( 4, 2, 2, 2, 4 ),
 ( 3, 3 ),
 ( 0.0001706658715691072165, 0.0002229276920778219600, 0.0002751895125865367036, 0.0003274513330952514472, 0.0003797131536039661907 ),
 ( 0.000000000000000000, 1.000000000000000000 ),
 .UNSPECIFIED. ) 
 GEOMETRIC_REPRESENTATION_ITEM ( )  RATIONAL_B_SPLINE_SURFACE ( (
 ( 1.000000000000000000, 0.7071067811865444641, 1.000000000000000000),
 ( 1.000000000000000000, 0.7375607040702822914, 1.000000000000000000),
 ( 1.000000000000000000, 0.7730431127429990834, 1.000000000000000000),
 ( 1.000000000000000000, 0.8321012486994672219, 1.000000000000000000),
 ( 1.000000000000000000, 0.8541932017419723300, 1.000000000000000000),
 ( 1.000000000000000000, 0.8545723906072110188, 1.000000000000000000),
 ( 1.000000000000000000, 0.8327032135058637374, 1.000000000000000000),
 ( 1.000000000000000000, 0.7734559727065434265, 1.000000000000000000),
 ( 1.000000000000000000, 0.7377766653997924751, 1.000000000000000000),
 ( 1.000000000000000000, 0.7071067811865456854, 1.000000000000000000) ) ) 
 REPRESENTATION_ITEM ( '' )  SURFACE ( )  );
#11326=CARTESIAN_POINT ( 'NONE',  ( 60.75000000000002842, -0.4999999999993606226, 1.554802467931481802 ) ) ;
#11329=ORIENTED_EDGE ( 'NONE', *, *, #1937, .T. ) ;
#11338=DIRECTION ( 'NONE',  ( 0.000000000000000000, 0.000000000000000000, 1.000000000000000000 ) ) ;
#11340=CIRCLE ( 'NONE', #716, 0.1499999999999999667 ) ;
#11342=CARTESIAN_POINT ( 'NONE',  ( 51.25000000000002842, -0.9938153758920951208, -1.589954715908409977 ) ) ;
#11349=DIRECTION ( 'NONE',  ( 0.000000000000000000, 0.000000000000000000, 1.000000000000000000 ) ) ;
#11362=CARTESIAN_POINT ( 'NONE',  ( 50.50000000000002132, 5.291762632692320630E-13, -1.996089927833914146 ) ) ;
#11367=CIRCLE ( 'NONE', #29080, 0.1500000000000001887 ) ;
#11374=CARTESIAN_POINT ( 'NONE',  ( 58.64999999999992042, -1.320082690054604546, 1.469015551795364916 ) ) ;
#11377=EDGE_LOOP ( 'NONE', ( #16266, #19178, #16739, #19123, #11425 ) ) ;
#11382=CARTESIAN_POINT ( 'NONE',  ( 58.65000000000002700, -0.5811678240974692544, 1.782657835994643447 ) ) ;
#11383=CARTESIAN_POINT ( 'NONE',  ( 51.45655683570189609, 0.9591657938401617622, -1.468576096419531352 ) ) ;
#11394=CARTESIAN_POINT ( 'NONE',  ( 52.20711756518984714, -0.7499999999994533262, -1.996089927833914146 ) ) ;
#11396=CARTESIAN_POINT ( 'NONE',  ( 51.12687253673781385, -0.9194130538815391551, -1.491219977510798600 ) ) ;
#11405=CARTESIAN_POINT ( 'NONE',  ( 51.45655683570189609, 0.9591657938401617622, 1.468576096419531352 ) ) ;
#11407=CARTESIAN_POINT ( 'NONE',  ( 58.72419296898066676, 1.799118770101964859, 0.5284032650199490533 ) ) ;
#11425=ORIENTED_EDGE ( 'NONE', *, *, #28171, .T. ) ;
#11426=ORIENTED_EDGE ( 'NONE', *, *, #17729, .F. ) ;
#11433=EDGE_CURVE ( 'NONE', #28767, #6209, #3507, .T. ) ;
#11436=DIRECTION ( 'NONE',  ( 0.000000000000000000, 0.000000000000000000, 1.000000000000000000 ) ) ;
#11440=CIRCLE ( 'NONE', #4362, 2.000000000000000000 ) ;
#11447=EDGE_CURVE ( 'NONE', #17367, #27461, #27867, .T. ) ;
#11448=CARTESIAN_POINT ( 'NONE',  ( 58.75000000000003553, -1.655311165516605509, -1.077297519404007087 ) ) ;
#11453=LINE ( 'NONE', #18000, #4455 ) ;
#11465=ORIENTED_EDGE ( 'NONE', *, *, #29803, .F. ) ;
#11466=CARTESIAN_POINT ( 'NONE',  ( 58.65000000000001990, 6.143261415694495821E-13, 3.111507638930570854E-58 ) ) ;
#11469=CARTESIAN_POINT ( 'NONE',  ( 58.74160516400039711, -1.575205926126199252, 1.017053542742779149 ) ) ;
#11478=ORIENTED_EDGE ( 'NONE', *, *, #21827, .T. ) ;
#11479=EDGE_CURVE ( 'NONE', #30820, #23063, #466, .T. ) ;
#11483=ORIENTED_EDGE ( 'NONE', *, *, #26317, .T. ) ;
#11485=LINE ( 'NONE', #20990, #24544 ) ;
#11486=CARTESIAN_POINT ( 'NONE',  ( 58.65000045311410304, 1.265716300432286223, 1.383426348887691448 ) ) ;
#11487=AXIS2_PLACEMENT_3D ( 'NONE', #16406, #26058, #16886 ) ;
#11491=FACE_OUTER_BOUND ( 'NONE', #5389, .T. ) ;
#11492=CARTESIAN_POINT ( 'NONE',  ( 51.31572262954152563, 0.7526089581382734428, -1.996089927833914146 ) ) ;
#11500=LINE ( 'NONE', #11172, #10434 ) ;
#11501=TOROIDAL_SURFACE ( 'NONE', #29200, 1.875000000000000222, 0.2500000000000000000 ) ;
#11508=SPHERICAL_SURFACE ( 'NONE', #28149, 0.2500000000000000000 ) ;
#11523=DIRECTION ( 'NONE',  ( 0.8262273428075421755, 0.5633368246415175751, 0.000000000000000000 ) ) ;
#11537=( BOUNDED_CURVE ( )  B_SPLINE_CURVE ( 3, ( #17886, #8220, #1405, #3769 ),
 .UNSPECIFIED., .F., .T. ) 
 B_SPLINE_CURVE_WITH_KNOTS ( ( 4, 4 ),
 ( 5.006444828673937586, 5.249382619234884473 ),
 .UNSPECIFIED. ) 
 CURVE ( )  GEOMETRIC_REPRESENTATION_ITEM ( )  RATIONAL_B_SPLINE_CURVE ( ( 1.000000000000000000, 0.9950878134350367166, 0.9950878134350367166, 1.000000000000000000 ) ) 
 REPRESENTATION_ITEM ( '' )  );
#11543=EDGE_LOOP ( 'NONE', ( #11932, #21937, #20865, #27993 ) ) ;
#11544=CARTESIAN_POINT ( 'NONE',  ( 58.72427158855720819, 1.646019958201105915, 0.8981388483289288738 ) ) ;
#11546=CARTESIAN_POINT ( 'NONE',  ( 58.65266784251151932, 0.9945725797260249745, -1.589569034372600775 ) ) ;
#11552=DIRECTION ( 'NONE',  ( 0.000000000000000000, -0.6683962987621306917, 0.7438053426811914726 ) ) ;
#11553=CARTESIAN_POINT ( 'NONE',  ( 58.75000000000002132, 6.153735859711025284E-13, 3.111507638930570854E-58 ) ) ;
#11554=CARTESIAN_POINT ( 'NONE',  ( 60.94140446608462014, 0.5380862305989584371, -1.858165151370887669 ) ) ;
#11570=DIRECTION ( 'NONE',  ( 1.000000000000000000, 1.047444401652940007E-14, 0.000000000000000000 ) ) ;
#11574=CARTESIAN_POINT ( 'NONE',  ( 58.75000000000003553, -1.320082690054267704, 1.469015551795647356 ) ) ;
#11578=DIRECTION ( 'NONE',  ( 0.000000000000000000, 0.000000000000000000, 1.000000000000000000 ) ) ;
#11580=CARTESIAN_POINT ( 'NONE',  ( 58.75000000000000000, 1.932246131437593162, 0.4087173687853760673 ) ) ;
#11584=ORIENTED_EDGE ( 'NONE', *, *, #5136, .T. ) ;
#11589=ADVANCED_FACE ( 'NONE', ( #8074 ), #8554, .F. ) ;
#11590=CARTESIAN_POINT ( 'NONE',  ( 58.75000000000000711, 0.8897917884438335534, 1.791164585743606041 ) ) ;
#11592=CARTESIAN_POINT ( 'NONE',  ( 58.65000038048045639, 1.873220289783266601, -0.08335421200033678313 ) ) ;
#11596=DIRECTION ( 'NONE',  ( 1.000000000000000000, 0.000000000000000000, 0.000000000000000000 ) ) ;
#11606=DIRECTION ( 'NONE',  ( 0.000000000000000000, 0.000000000000000000, 1.000000000000000000 ) ) ;
#11607=DIRECTION ( 'NONE',  ( 0.000000000000000000, 0.000000000000000000, 1.000000000000000000 ) ) ;
#11615=VERTEX_POINT ( 'NONE', #10749 ) ;
#11616=CARTESIAN_POINT ( 'NONE',  ( 51.17290532404553716, -0.9646187004837835088, -1.462925393634369353 ) ) ;
#11626=CARTESIAN_POINT ( 'NONE',  ( 51.64281244548084970, 0.8321733326272462428, 1.569379851958426331 ) ) ;
#11633=CARTESIAN_POINT ( 'NONE',  ( 58.74154451056427462, -1.668374833162466153, 0.8556855217791524693 ) ) ;
#11638=FACE_OUTER_BOUND ( 'NONE', #17866, .T. ) ;
#11639=ORIENTED_EDGE ( 'NONE', *, *, #20587, .F. ) ;
#11644=CARTESIAN_POINT ( 'NONE',  ( 58.64999999999999858, 1.655311165517639349, -1.077297519404308179 ) ) ;
#11645=ORIENTED_EDGE ( 'NONE', *, *, #25955, .T. ) ;
#11647=DIRECTION ( 'NONE',  ( 1.000000000000000000, 1.047444401652940007E-14, -0.000000000000000000 ) ) ;
#11654=CARTESIAN_POINT ( 'NONE',  ( 60.94140446606686368, -0.5380862305903196807, -1.858165151418244010 ) ) ;
#11656=CARTESIAN_POINT ( 'NONE',  ( 58.75000000000002132, 6.153735859711025284E-13, 3.111507638930570854E-58 ) ) ;
#11658=ADVANCED_FACE ( 'NONE', ( #25466 ), #3771, .T. ) ;
#11668=CARTESIAN_POINT ( 'NONE',  ( 60.81561938753818453, 0.6500000000006365131, -1.489337100860648633 ) ) ;
#11672=CARTESIAN_POINT ( 'NONE',  ( 58.75000000000003553, -1.932246131436463843, -0.4087173687848976722 ) ) ;
#11675=CARTESIAN_POINT ( 'NONE',  ( 58.65000038048045639, 1.787818198675105386, -0.5653390727695211115 ) ) ;
#11698=FACE_OUTER_BOUND ( 'NONE', #14116, .T. ) ;
#11700=CARTESIAN_POINT ( 'NONE',  ( 50.59602332238209499, -0.1408342061598474859, 0.8215393206232036727 ) ) ;
#11702=DIRECTION ( 'NONE',  ( 0.000000000000000000, -1.000000000000000000, 0.000000000000000000 ) ) ;
#11707=DIRECTION ( 'NONE',  ( -0.000000000000000000, -0.000000000000000000, -1.000000000000000000 ) ) ;
#11710=AXIS2_PLACEMENT_3D ( 'NONE', #19895, #24790, #27323 ) ;
#11712=DIRECTION ( 'NONE',  ( 0.5633368246415186853, -0.8262273428075416204, 0.000000000000000000 ) ) ;
#11718=DIRECTION ( 'NONE',  ( 0.000000000000000000, 0.000000000000000000, 1.000000000000000000 ) ) ;
#11723=CARTESIAN_POINT ( 'NONE',  ( 50.25000000000004263, -1.791164585743077797, 0.8897917884442223535 ) ) ;
#11730=ADVANCED_FACE ( 'NONE', ( #6311 ), #27151, .F. ) ;
#11731=CARTESIAN_POINT ( 'NONE',  ( 58.65000038048068376, -1.787818198674085757, 0.5653390727688525352 ) ) ;
#11737=ORIENTED_EDGE ( 'NONE', *, *, #2062, .T. ) ;
#11738=ORIENTED_EDGE ( 'NONE', *, *, #18563, .F. ) ;
#11743=ORIENTED_EDGE ( 'NONE', *, *, #17031, .F. ) ;
#11744=CARTESIAN_POINT ( 'NONE',  ( 58.66118217212520136, 1.874997884620083211, -0.01689491344017308647 ) ) ;
#11746=EDGE_CURVE ( 'NONE', #22512, #30820, #15161, .T. ) ;
#11753=CARTESIAN_POINT ( 'NONE',  ( 60.94140446606686368, -0.5380862305903196807, -1.858165151418244010 ) ) ;
#11754=DIRECTION ( 'NONE',  ( 1.000000000000000000, 1.047444401652940007E-14, 0.000000000000000000 ) ) ;
#11767=ORIENTED_EDGE ( 'NONE', *, *, #30200, .T. ) ;
#11768=LINE ( 'NONE', #23812, #18045 ) ;
#11792=CARTESIAN_POINT ( 'NONE',  ( 58.75000000000002842, -0.8980135333480974147, -1.749295403805072757 ) ) ;
#11793=ORIENTED_EDGE ( 'NONE', *, *, #1505, .F. ) ;
#11796=DIRECTION ( 'NONE',  ( 0.000000000000000000, -1.000000000000000000, 0.000000000000000000 ) ) ;
#11798=ADVANCED_FACE ( 'NONE', ( #11698 ), #30321, .F. ) ;
#11801=CARTESIAN_POINT ( 'NONE',  ( 58.65000000000004121, -1.834410884275093911, -0.3880228184666750235 ) ) ;
#11802=CARTESIAN_POINT ( 'NONE',  ( 51.22715433738865443, 0.9941391646906797552, 1.410349289489640556 ) ) ;
#11803=DIRECTION ( 'NONE',  ( 1.000000000000000000, 1.047444401652940007E-14, 0.000000000000000000 ) ) ;
#11804=DIRECTION ( 'NONE',  ( 0.000000000000000000, 0.000000000000000000, 1.000000000000000000 ) ) ;
#11806=ORIENTED_EDGE ( 'NONE', *, *, #30479, .T. ) ;
#11809=CARTESIAN_POINT ( 'NONE',  ( 58.72973946704998127, 0.5000000000006151746, -1.835413506853449395 ) ) ;
#11818=ORIENTED_EDGE ( 'NONE', *, *, #6230, .T. ) ;
#11819=LINE ( 'NONE', #6281, #10504 ) ;
#11820=EDGE_LOOP ( 'NONE', ( #14618, #21618, #13125, #9766, #14794 ) ) ;
#11823=ORIENTED_EDGE ( 'NONE', *, *, #17334, .F. ) ;
#11831=EDGE_CURVE ( 'NONE', #21960, #2526, #490, .T. ) ;
#11839=CARTESIAN_POINT ( 'NONE',  ( 50.25000000000004263, -1.895722432252775924, -0.6373668173469783094 ) ) ;
#11843=EDGE_CURVE ( 'NONE', #15867, #704, #19624, .T. ) ;
#11847=CARTESIAN_POINT ( 'NONE',  ( 58.65000045311411014, 1.008695754911338227, -1.580645149930956617 ) ) ;
#11852=DIRECTION ( 'NONE',  ( 0.000000000000000000, 0.000000000000000000, 1.000000000000000000 ) ) ;
#11854=VERTEX_POINT ( 'NONE', #7574 ) ;
#11857=CARTESIAN_POINT ( 'NONE',  ( 61.24473505568541754, 0.9276313280772279235, 1.700547749641277084 ) ) ;
#11859=CARTESIAN_POINT ( 'NONE',  ( 60.75000000000001421, 0.5000000000006363798, 1.718465885608440047 ) ) ;
#11865=EDGE_CURVE ( 'NONE', #7647, #19414, #4876, .T. ) ;
#11873=CIRCLE ( 'NONE', #31078, 1.975000000000001865 ) ;
#11875=DIRECTION ( 'NONE',  ( 0.000000000000000000, 0.000000000000000000, 1.000000000000000000 ) ) ;
#11883=CARTESIAN_POINT ( 'NONE',  ( 51.84772254680354564, -0.6924618999061498137, -1.653428777428161300 ) ) ;
#11889=CARTESIAN_POINT ( 'NONE',  ( 51.45655683570189609, 0.9591657938401617622, -1.468576096419531352 ) ) ;
#11892=AXIS2_PLACEMENT_3D ( 'NONE', #11466, #11291, #27621 ) ;
#11895=CARTESIAN_POINT ( 'NONE',  ( 51.31572262954152563, 1.002608958138273554, -1.996089927833914146 ) ) ;
#11904=LINE ( 'NONE', #11266, #1917 ) ;
#11917=ORIENTED_EDGE ( 'NONE', *, *, #26043, .F. ) ;
#11926=VERTEX_POINT ( 'NONE', #589 ) ;
#11927=DIRECTION ( 'NONE',  ( 0.000000000000000000, 0.000000000000000000, 1.000000000000000000 ) ) ;
#11928=CARTESIAN_POINT ( 'NONE',  ( 58.75000000000000711, 1.800471618824943221, -1.039502773795712987 ) ) ;
#11932=ORIENTED_EDGE ( 'NONE', *, *, #18532, .T. ) ;
#11941=CARTESIAN_POINT ( 'NONE',  ( 51.49472959044967268, -1.070956530527746864, 1.224612562803249594 ) ) ;
#11942=AXIS2_PLACEMENT_3D ( 'NONE', #2170, #21683, #21511 ) ;
#11952=CARTESIAN_POINT ( 'NONE',  ( 58.72204580543405683, -0.9570475208903724829, -1.612507782425579350 ) ) ;
#11963=CIRCLE ( 'NONE', #29646, 2.000000000000000000 ) ;
#11966=VECTOR ( 'NONE', #9928, 1000.000000000000000 ) ;
#11968=CARTESIAN_POINT ( 'NONE',  ( 58.66324791596939292, 0.5000000000006143974, -1.807104036850105677 ) ) ;
#11973=FACE_OUTER_BOUND ( 'NONE', #12806, .T. ) ;
#11978=CARTESIAN_POINT ( 'NONE',  ( 58.65000000000001990, 6.143261415694495821E-13, 3.111507638930570854E-58 ) ) ;
#11979=ORIENTED_EDGE ( 'NONE', *, *, #11447, .F. ) ;
#11981=VERTEX_POINT ( 'NONE', #20246 ) ;
#11983=EDGE_CURVE ( 'NONE', #28572, #5002, #21775, .T. ) ;
#11987=VECTOR ( 'NONE', #16144, 1000.000000000000000 ) ;
#11989=CARTESIAN_POINT ( 'NONE',  ( 50.25000000000000000, 2.079005547593327119, 1.004182178118534636E-12 ) ) ;
#11991=AXIS2_PLACEMENT_3D ( 'NONE', #19793, #24687, #19649 ) ;
#11992=DIRECTION ( 'NONE',  ( 0.000000000000000000, 0.000000000000000000, 1.000000000000000000 ) ) ;
#11998=CARTESIAN_POINT ( 'NONE',  ( 58.65000000000001279, 0.5539202450380567022, 1.791540873398024036 ) ) ;
#11999=CIRCLE ( 'NONE', #9478, 0.1500000000000001887 ) ;
#12007=CARTESIAN_POINT ( 'NONE',  ( 58.65000000000000568, 1.394635017529600507, -1.253243060177047896 ) ) ;
#12009=VERTEX_POINT ( 'NONE', #20555 ) ;
#12011=CIRCLE ( 'NONE', #16048, 0.09999999999999990841 ) ;
#12014=CARTESIAN_POINT ( 'NONE',  ( 58.72427158855710161, 0.8981388483285237534, -1.646019958201040190 ) ) ;
#12017=EDGE_CURVE ( 'NONE', #7673, #19795, #21248, .T. ) ;
#12018=CARTESIAN_POINT ( 'NONE',  ( 51.25000000000002842, -1.099999999999459410, 1.001327244211406953 ) ) ;
#12022=CIRCLE ( 'NONE', #6462, 0.1500000000000003830 ) ;
#12024=CARTESIAN_POINT ( 'NONE',  ( 58.74999999305995857, 0.9867593359915998175, 1.657788420846524557 ) ) ;
#12025=EDGE_CURVE ( 'NONE', #16439, #12125, #29878, .T. ) ;
#12047=CARTESIAN_POINT ( 'NONE',  ( 61.24504608472945932, -0.9290853280804240999, 1.697615787671056697 ) ) ;
#12057=ORIENTED_EDGE ( 'NONE', *, *, #23521, .F. ) ;
#12058=VERTEX_POINT ( 'NONE', #12926 ) ;
#12059=CARTESIAN_POINT ( 'NONE',  ( 58.75000000000000711, 1.039502773797200019, -1.800471618823823450 ) ) ;
#12064=CARTESIAN_POINT ( 'NONE',  ( 58.74472430272347623, 0.5000000000006152856, 1.853787220596809782 ) ) ;
#12072=ORIENTED_EDGE ( 'NONE', *, *, #1847, .F. ) ;
#12078=TOROIDAL_SURFACE ( 'NONE', #425, 1.975000000000001865, 0.1000000000000000056 ) ;
#12089=CARTESIAN_POINT ( 'NONE',  ( 58.75000000000002132, -0.5380862305913116650, 2.008165151418990213 ) ) ;
#12094=EDGE_LOOP ( 'NONE', ( #28660, #10961, #10357, #22879, #15918 ) ) ;
#12097=VERTEX_POINT ( 'NONE', #3124 ) ;
#12113=FACE_OUTER_BOUND ( 'NONE', #14471, .T. ) ;
#12119=CARTESIAN_POINT ( 'NONE',  ( 61.25000000000001421, 1.106298139390920365, -1.666164585742239357 ) ) ;
#12125=VERTEX_POINT ( 'NONE', #5988 ) ;
#12132=DIRECTION ( 'NONE',  ( 0.000000000000000000, 0.000000000000000000, 1.000000000000000000 ) ) ;
#12133=FACE_OUTER_BOUND ( 'NONE', #29502, .T. ) ;
#12144=DIRECTION ( 'NONE',  ( 1.000000000000000000, 1.047444401652940007E-14, 0.000000000000000000 ) ) ;
#12159=CARTESIAN_POINT ( 'NONE',  ( 61.23770293223015670, -0.8897917884444476178, 1.791164585743103999 ) ) ;
#12160=CARTESIAN_POINT ( 'NONE',  ( 58.66133336607639137, 1.302803168108718879, -1.348863877412651791 ) ) ;
#12164=VERTEX_POINT ( 'NONE', #4999 ) ;
#12165=EDGE_CURVE ( 'NONE', #7871, #16027, #9112, .T. ) ;
#12169=ADVANCED_FACE ( 'NONE', ( #24460 ), #7681, .F. ) ;
#12177=CARTESIAN_POINT ( 'NONE',  ( 61.24637336955049705, 0.9388313581417159215, 1.688008567905789237 ) ) ;
#12193=DIRECTION ( 'NONE',  ( -1.451851013137922794E-14, 0.8914544820238117229, -0.4531102586343168093 ) ) ;
#12196=CARTESIAN_POINT ( 'NONE',  ( 58.75000000000001421, 0.6121634413823866527, 1.877732920581527409 ) ) ;
#12198=ORIENTED_EDGE ( 'NONE', *, *, #8075, .F. ) ;
#12199=CARTESIAN_POINT ( 'NONE',  ( 58.75000000000004263, -1.932246131436417436, 0.4087173687851148873 ) ) ;
#12217=EDGE_LOOP ( 'NONE', ( #13060, #22379, #19354, #17414 ) ) ;
#12227=ADVANCED_FACE ( 'NONE', ( #12133 ), #19587, .T. ) ;
#12229=CARTESIAN_POINT ( 'NONE',  ( 51.64837794009019944, 0.8283786772117788244, -1.688958810662479104 ) ) ;
#12232=VERTEX_POINT ( 'NONE', #12581 ) ;
#12238=ORIENTED_EDGE ( 'NONE', *, *, #2544, .T. ) ;
#12241=ORIENTED_EDGE ( 'NONE', *, *, #29768, .F. ) ;
#12245=CARTESIAN_POINT ( 'NONE',  ( 61.09423418604048095, 0.6373668173476213505, -1.895722432252298084 ) ) ;
#12246=ORIENTED_EDGE ( 'NONE', *, *, #27243, .F. ) ;
#12256=CARTESIAN_POINT ( 'NONE',  ( 58.75000000000002842, -1.066009655020577096, -1.652371589363125004 ) ) ;
#12259=EDGE_CURVE ( 'NONE', #203, #9827, #19569, .T. ) ;
#12261=CYLINDRICAL_SURFACE ( 'NONE', #27038, 0.1500000000000002720 ) ;
#12262=FACE_OUTER_BOUND ( 'NONE', #28444, .T. ) ;
#12265=ORIENTED_EDGE ( 'NONE', *, *, #9337, .T. ) ;
#12276=ORIENTED_EDGE ( 'NONE', *, *, #22145, .T. ) ;
#12280=CARTESIAN_POINT ( 'NONE',  ( 51.18880157753722671, -1.010242313720678631, 1.292695951881193794 ) ) ;
#12282=CARTESIAN_POINT ( 'NONE',  ( 58.75000000000004263, -2.079005547593188119, 1.932245437381540134E-15 ) ) ;
#12293=DIRECTION ( 'NONE',  ( 1.000000000000000000, 1.047444401652940007E-14, 0.000000000000000000 ) ) ;
#12297=EDGE_CURVE ( 'NONE', #11854, #22512, #6925, .T. ) ;
#12306=CARTESIAN_POINT ( 'NONE',  ( 51.45655683570191741, -0.9591657938390835136, -1.196087371390569087 ) ) ;
#12308=VERTEX_POINT ( 'NONE', #27155 ) ;
#12311=CARTESIAN_POINT ( 'NONE',  ( 58.75000000000002132, 6.153735859711025284E-13, 3.111507638930570854E-58 ) ) ;
#12317=CARTESIAN_POINT ( 'NONE',  ( 50.25000000000003553, -1.499837071477821082, -1.323060376181415254 ) ) ;
#12326=CARTESIAN_POINT ( 'NONE',  ( 58.65000000000001279, 0.8948927608033908632, 1.760622601997029690 ) ) ;
#12328=CARTESIAN_POINT ( 'NONE',  ( 61.25000000000000000, 1.791164585743364901, -0.8897917884432851032 ) ) ;
#12329=LINE ( 'NONE', #19483, #28154 ) ;
#12331=ORIENTED_EDGE ( 'NONE', *, *, #28902, .F. ) ;
#12332=CARTESIAN_POINT ( 'NONE',  ( 58.75000018595673623, -1.857295262527126845, 0.5493460779660276350 ) ) ;
#12338=DIRECTION ( 'NONE',  ( 1.000000000000000000, 1.047444401652940007E-14, 0.000000000000000000 ) ) ;
#12340=AXIS2_PLACEMENT_3D ( 'NONE', #126, #19151, #4866 ) ;
#12341=ORIENTED_EDGE ( 'NONE', *, *, #22851, .T. ) ;
#12344=DIRECTION ( 'NONE',  ( -1.000000000000000000, -1.047444401652940007E-14, -0.000000000000000000 ) ) ;
#12360=PLANE ( 'NONE',  #24163 ) ;
#12362=DIRECTION ( 'NONE',  ( 0.000000000000000000, 0.000000000000000000, 1.000000000000000000 ) ) ;
#12364=VECTOR ( 'NONE', #24617, 1000.000000000000000 ) ;
#12376=FACE_OUTER_BOUND ( 'NONE', #17333, .T. ) ;
#12385=EDGE_CURVE ( 'NONE', #2387, #12697, #359, .T. ) ;
#12387=EDGE_LOOP ( 'NONE', ( #18884, #27656, #25875, #20850 ) ) ;
#12395=AXIS2_PLACEMENT_3D ( 'NONE', #31237, #4002, #13648 ) ;
#12398=VECTOR ( 'NONE', #10938, 1000.000000000000000 ) ;
#12401=CARTESIAN_POINT ( 'NONE',  ( 58.74999981404334903, -1.050697058759886948, -1.649595783782785263 ) ) ;
#12409=CARTESIAN_POINT ( 'NONE',  ( 58.64999999999999858, 1.874150328521186681, -0.06593717335319848605 ) ) ;
#12418=CYLINDRICAL_SURFACE ( 'NONE', #23160, 0.5000000000000000000 ) ;
#12420=ORIENTED_EDGE ( 'NONE', *, *, #28589, .F. ) ;
#12424=VERTEX_POINT ( 'NONE', #23199 ) ;
#12443=CIRCLE ( 'NONE', #322, 0.1500000000000001887 ) ;
#12449=CARTESIAN_POINT ( 'NONE',  ( 58.75000000000003553, -1.800471618824212694, -1.039502773796582069 ) ) ;
#12473=DIRECTION ( 'NONE',  ( 0.000000000000000000, -0.9985773570673280863, 0.05332224631830469186 ) ) ;
#12480=DIRECTION ( 'NONE',  ( -1.000000000000000000, -1.047444401652940007E-14, -0.000000000000000000 ) ) ;
#12487=EDGE_CURVE ( 'NONE', #29731, #1382, #24088, .T. ) ;
#12489=CARTESIAN_POINT ( 'NONE',  ( 51.15311061045468222, 0.9578955620007181260, 1.386733222354203487 ) ) ;
#12492=CIRCLE ( 'NONE', #25141, 0.1500000000000001887 ) ;
#12494=ORIENTED_EDGE ( 'NONE', *, *, #10358, .T. ) ;
#12502=DIRECTION ( 'NONE',  ( 1.000000000000000000, 1.047444401652940007E-14, 0.000000000000000000 ) ) ;
#12510=EDGE_CURVE ( 'NONE', #21772, #19129, #23630, .T. ) ;
#12514=CIRCLE ( 'NONE', #17080, 0.1500000000000001887 ) ;
#12516=CIRCLE ( 'NONE', #23661, 1.875000000000001776 ) ;
#12519=VECTOR ( 'NONE', #19593, 1000.000000000000000 ) ;
#12528=AXIS2_PLACEMENT_3D ( 'NONE', #15895, #25253, #5782 ) ;
#12533=ORIENTED_EDGE ( 'NONE', *, *, #26718, .F. ) ;
#12544=VERTEX_POINT ( 'NONE', #3325 ) ;
#12554=AXIS2_PLACEMENT_3D ( 'NONE', #19344, #17262, #9987 ) ;
#12556=ORIENTED_EDGE ( 'NONE', *, *, #17031, .T. ) ;
#12560=DIRECTION ( 'NONE',  ( 0.000000000000000000, 0.8381322357049212357, 0.5454670984324081484 ) ) ;
#12564=DIRECTION ( 'NONE',  ( 0.000000000000000000, 0.000000000000000000, 1.000000000000000000 ) ) ;
#12565=EDGE_CURVE ( 'NONE', #28405, #29835, #1372, .T. ) ;
#12566=CARTESIAN_POINT ( 'NONE',  ( 58.66054497608116947, -0.4999999999856035160, 1.807104036853935503 ) ) ;
#12578=PRODUCT_DEFINITION_SHAPE ( 'NONE', 'NONE',  #17468 ) ;
#12581=CARTESIAN_POINT ( 'NONE',  ( 58.75000000000000711, 1.323060376182032760, -1.499837071477343242 ) ) ;
#12582=VERTEX_POINT ( 'NONE', #22489 ) ;
#12585=ORIENTED_EDGE ( 'NONE', *, *, #26718, .T. ) ;
#12598=CARTESIAN_POINT ( 'NONE',  ( 58.66133336607619952, 1.819551968141050136, 0.4538287010067406646 ) ) ;
#12603=DIRECTION ( 'NONE',  ( 0.000000000000000000, 0.000000000000000000, 1.000000000000000000 ) ) ;
#12609=CARTESIAN_POINT ( 'NONE',  ( 51.49777277048506363, -1.059151787767940389, -1.232523824083111563 ) ) ;
#12612=CARTESIAN_POINT ( 'NONE',  ( 58.75000000000003553, -1.666164585742988091, 1.106298139390331947 ) ) ;
#12616=CARTESIAN_POINT ( 'NONE',  ( 61.25000000000002132, 6.415596960124259844E-13, 3.111507638930570854E-58 ) ) ;
#12617=DIRECTION ( 'NONE',  ( 1.000000000000000000, 1.047444401652940007E-14, 0.000000000000000000 ) ) ;
#12620=EDGE_CURVE ( 'NONE', #4687, #9856, #29148, .T. ) ;
#12622=CIRCLE ( 'NONE', #30323, 0.1499999999999999667 ) ;
#12625=DIRECTION ( 'NONE',  ( 1.000000000000000000, 1.047444401652940007E-14, -0.000000000000000000 ) ) ;
#12629=LINE ( 'NONE', #22314, #3253 ) ;
#12635=ORIENTED_EDGE ( 'NONE', *, *, #13473, .F. ) ;
#12644=ORIENTED_EDGE ( 'NONE', *, *, #2782, .F. ) ;
#12648=DIRECTION ( 'NONE',  ( 1.000000000000000000, 1.047444401652940007E-14, 0.000000000000000000 ) ) ;
#12656=( BOUNDED_SURFACE ( )  B_SPLINE_SURFACE ( 3, 2, ( 
 ( #12196, #21875, #9978 ),
 ( #162, #7601, #26899 ),
 ( #5211, #24522, #14859 ),
 ( #19944, #27517, #13256 ) ),
 .UNSPECIFIED., .F., .F., .F. ) 
 B_SPLINE_SURFACE_WITH_KNOTS ( ( 4, 4 ),
 ( 3, 3 ),
 ( 0.0001706658715695485952, 0.0002755376070443638472 ),
 ( 0.000000000000000000, 1.000000000000000000 ),
 .UNSPECIFIED. ) 
 GEOMETRIC_REPRESENTATION_ITEM ( )  RATIONAL_B_SPLINE_SURFACE ( (
 ( 1.000000000000000000, 0.7071067811865487940, 1.000000000000000000),
 ( 1.000000000000000000, 0.7664791242981755515, 1.000000000000000000),
 ( 1.000000000000000000, 0.8546216002033862891, 1.000000000000000000),
 ( 1.000000000000000000, 0.8543839179668213379, 1.000000000000000000) ) ) 
 REPRESENTATION_ITEM ( '' )  SURFACE ( )  );
#12659=DIRECTION ( 'NONE',  ( 0.000000000000000000, 0.000000000000000000, 1.000000000000000000 ) ) ;
#12663=CARTESIAN_POINT ( 'NONE',  ( 58.65000045311413857, -1.265716300431979358, -1.383426348886848123 ) ) ;
#12667=AXIS2_PLACEMENT_3D ( 'NONE', #29483, #22385, #17638 ) ;
#12677=EDGE_CURVE ( 'NONE', #14419, #20749, #30381, .T. ) ;
#12679=DIRECTION ( 'NONE',  ( 1.000000000000000000, 1.047444401652940007E-14, -0.000000000000000000 ) ) ;
#12680=CARTESIAN_POINT ( 'NONE',  ( 52.06628335902944826, 0.5434431642986571331, -1.794517909405660694 ) ) ;
#12683=ORIENTED_EDGE ( 'NONE', *, *, #28491, .F. ) ;
#12684=B_SPLINE_CURVE_WITH_KNOTS ( 'NONE', 3,
 ( #26272, #26424, #21534, #2528, #19170, #14702, #11857, #12177, #21997, #23900, #26884, #28810, #2359 ),
 .UNSPECIFIED., .F., .F.,
 ( 4, 3, 3, 3, 4 ),
 ( 0.000000000000000000, 4.994367907427477767E-05, 9.982969917209731626E-05, 0.0001505119896697553904, 0.0001857353029114525904 ),
 .UNSPECIFIED. ) ;
#12696=ORIENTED_EDGE ( 'NONE', *, *, #14849, .T. ) ;
#12697=VERTEX_POINT ( 'NONE', #15969 ) ;
#12703=CARTESIAN_POINT ( 'NONE',  ( 61.23770293222996486, -0.8897917884435792013, -1.791164585742600179 ) ) ;
#12710=CARTESIAN_POINT ( 'NONE',  ( 60.75000000000001421, 0.6500000000006362910, 1.489337100860648189 ) ) ;
#12713=DIRECTION ( 'NONE',  ( 1.000000000000000000, 1.047444401652940007E-14, 0.000000000000000000 ) ) ;
#12715=CARTESIAN_POINT ( 'NONE',  ( 51.31572262954149721, 1.002608958138273554, 1.395204572094392192 ) ) ;
#12723=CARTESIAN_POINT ( 'NONE',  ( 58.65838214097848891, 1.301971553120403025, -1.349359547238234036 ) ) ;
#12724=VECTOR ( 'NONE', #5753, 1000.000000000000000 ) ;
#12728=ORIENTED_EDGE ( 'NONE', *, *, #18537, .F. ) ;
#12730=VERTEX_POINT ( 'NONE', #10757 ) ;
#12736=EDGE_LOOP ( 'NONE', ( #14224, #14835, #21442, #26235, #28832 ) ) ;
#12744=ORIENTED_EDGE ( 'NONE', *, *, #21512, .T. ) ;
#12748=ADVANCED_FACE ( 'NONE', ( #27862 ), #1436, .F. ) ;
#12751=FACE_OUTER_BOUND ( 'NONE', #30146, .T. ) ;
#12752=CARTESIAN_POINT ( 'NONE',  ( 50.55258015808398397, 5.295040916136730406E-13, 1.177580158083963546 ) ) ;
#12755=CARTESIAN_POINT ( 'NONE',  ( 58.75000000000003553, -1.877732920580702958, 0.6121634413824121879 ) ) ;
#12760=CARTESIAN_POINT ( 'NONE',  ( 61.21684424624547205, -0.7974861228894950527, 1.837019011345026653 ) ) ;
#12765=ORIENTED_EDGE ( 'NONE', *, *, #7061, .F. ) ;
#12767=CARTESIAN_POINT ( 'NONE',  ( 50.25000000000003553, -1.470078920827295965, -1.470078920827526892 ) ) ;
#12775=ORIENTED_EDGE ( 'NONE', *, *, #11865, .T. ) ;
#12776=ORIENTED_EDGE ( 'NONE', *, *, #13915, .F. ) ;
#12779=EDGE_CURVE ( 'NONE', #6559, #29235, #30876, .T. ) ;
#12785=DIRECTION ( 'NONE',  ( 1.000000000000000000, 1.047444401652940007E-14, 0.000000000000000000 ) ) ;
#12801=AXIS2_PLACEMENT_3D ( 'NONE', #7495, #17299, #24566 ) ;
#12802=ORIENTED_EDGE ( 'NONE', *, *, #12510, .F. ) ;
#12804=CARTESIAN_POINT ( 'NONE',  ( 51.14630318392396902, -0.9364487020628400327, 1.503522130792752209 ) ) ;
#12806=EDGE_LOOP ( 'NONE', ( #15187, #29119, #3675, #26382 ) ) ;
#12812=CARTESIAN_POINT ( 'NONE',  ( 58.65263613458542835, -1.372222488449002187, -1.277852321299007610 ) ) ;
#12818=CIRCLE ( 'NONE', #7280, 0.1000000000000000333 ) ;
#12822=CARTESIAN_POINT ( 'NONE',  ( 50.25000000000002842, -0.8897917884436942204, -1.791164585742600179 ) ) ;
#12835=DIRECTION ( 'NONE',  ( 0.000000000000000000, 0.000000000000000000, 1.000000000000000000 ) ) ;
#12856=EDGE_CURVE ( 'NONE', #22920, #507, #4465, .T. ) ;
#12860=CARTESIAN_POINT ( 'NONE',  ( 61.25000000000001421, 1.000000000000641709, 1.586072192556190252 ) ) ;
#12863=AXIS2_PLACEMENT_3D ( 'NONE', #1030, #2934, #27152 ) ;
#12865=DIRECTION ( 'NONE',  ( 0.000000000000000000, 0.000000000000000000, 1.000000000000000000 ) ) ;
#12870=CARTESIAN_POINT ( 'NONE',  ( 58.66864673770970029, -0.4999999999993857136, 1.807442289571351335 ) ) ;
#12872=CARTESIAN_POINT ( 'NONE',  ( 58.73379417893110599, 1.267842757871880277, -1.381558089342544537 ) ) ;
#12876=CARTESIAN_POINT ( 'NONE',  ( 52.10742184747378758, 0.5153941949047937676, 1.803012124260139570 ) ) ;
#12877=ORIENTED_EDGE ( 'NONE', *, *, #13333, .F. ) ;
#12878=EDGE_LOOP ( 'NONE', ( #20797, #29399, #26869, #26871 ) ) ;
#12882=CARTESIAN_POINT ( 'NONE',  ( 58.65000000000004121, -1.877732920580617693, -0.6121634413826788634 ) ) ;
#12884=ORIENTED_EDGE ( 'NONE', *, *, #1726, .T. ) ;
#12887=ORIENTED_EDGE ( 'NONE', *, *, #2514, .F. ) ;
#12898=AXIS2_PLACEMENT_3D ( 'NONE', #6644, #1895, #14232 ) ;
#12900=B_SPLINE_CURVE_WITH_KNOTS ( 'NONE', 3,
 ( #15099, #25056, #22248, #22866 ),
 .UNSPECIFIED., .F., .F.,
 ( 4, 4 ),
 ( 0.0001886355468578361809, 0.0003849279710740182033 ),
 .UNSPECIFIED. ) ;
#12903=CARTESIAN_POINT ( 'NONE',  ( 51.36308620441098327, 1.097739233406258563, 1.198394850649636689 ) ) ;
#12910=CARTESIAN_POINT ( 'NONE',  ( 51.59739104186229497, -1.010292945602101256, 1.272765950230260623 ) ) ;
#12918=ORIENTED_EDGE ( 'NONE', *, *, #909, .T. ) ;
#12921=AXIS2_PLACEMENT_3D ( 'NONE', #18137, #15592, #1480 ) ;
#12923=CARTESIAN_POINT ( 'NONE',  ( 61.25000000000000000, 2.008165151418888072, -0.5380862305899540843 ) ) ;
#12926=CARTESIAN_POINT ( 'NONE',  ( 58.75000000000000000, 1.996089927834530986, 0.1250000000010043355 ) ) ;
#12927=EDGE_LOOP ( 'NONE', ( #9872, #6003, #31152, #21463 ) ) ;
#12928=CARTESIAN_POINT ( 'NONE',  ( 60.82068433953604369, -0.6500001811771835003, -1.489337021788164739 ) ) ;
#12930=ORIENTED_EDGE ( 'NONE', *, *, #8109, .F. ) ;
#12934=ORIENTED_EDGE ( 'NONE', *, *, #17523, .F. ) ;
#12942=AXIS2_PLACEMENT_3D ( 'NONE', #30289, #3689, #16046 ) ;
#12944=CARTESIAN_POINT ( 'NONE',  ( 51.98914612709258876, -0.7788013043298228633, 1.433123603079414776 ) ) ;
#12945=CIRCLE ( 'NONE', #6372, 1.975000000000001865 ) ;
#12953=AXIS2_PLACEMENT_3D ( 'NONE', #26892, #4896, #7438 ) ;
#12954=ADVANCED_FACE ( 'NONE', ( #7873 ), #27202, .F. ) ;
#12963=ORIENTED_EDGE ( 'NONE', *, *, #9226, .T. ) ;
#12964=ADVANCED_FACE ( 'NONE', ( #19630 ), #22310, .F. ) ;
#12968=CIRCLE ( 'NONE', #25106, 0.1500000000000001887 ) ;
#13009=CARTESIAN_POINT ( 'NONE',  ( 58.65000000000002700, -0.8495817349395312634, -1.671477153794241666 ) ) ;
#13010=DIRECTION ( 'NONE',  ( 0.000000000000000000, 0.000000000000000000, 1.000000000000000000 ) ) ;
#13021=FILL_AREA_STYLE_COLOUR ( '', #28272 ) ;
#13022=CARTESIAN_POINT ( 'NONE',  ( 51.43901883478556414, 0.9711235217376542606, -1.449592546241924573 ) ) ;
#13029=CARTESIAN_POINT ( 'NONE',  ( 51.64333574538934357, 0.8318165372350851960, -1.569663068107118642 ) ) ;
#13032=CARTESIAN_POINT ( 'NONE',  ( 60.99000702708163857, 0.5469907030331696562, 1.538545889480190665 ) ) ;
#13033=DIRECTION ( 'NONE',  ( 0.000000000000000000, 0.000000000000000000, 1.000000000000000000 ) ) ;
#13037=( BOUNDED_CURVE ( )  B_SPLINE_CURVE ( 3, ( #11405, #13451, #6813, #25495 ),
 .UNSPECIFIED., .F., .T. ) 
 B_SPLINE_CURVE_WITH_KNOTS ( ( 4, 4 ),
 ( 4.041453792691653391, 4.300872134317200945 ),
 .UNSPECIFIED. ) 
 CURVE ( )  GEOMETRIC_REPRESENTATION_ITEM ( )  RATIONAL_B_SPLINE_CURVE ( ( 1.000000000000000000, 0.9943997021150918769, 0.9943997021150918769, 1.000000000000000000 ) ) 
 REPRESENTATION_ITEM ( '' )  );
#13039=DIRECTION ( 'NONE',  ( 0.000000000000000000, 0.000000000000000000, 1.000000000000000000 ) ) ;
#13045=CARTESIAN_POINT ( 'NONE',  ( 58.75000000000000711, 1.320082690054482866, -1.469015551796560404 ) ) ;
#13058=DIRECTION ( 'NONE',  ( 0.000000000000000000, 0.000000000000000000, 1.000000000000000000 ) ) ;
#13060=ORIENTED_EDGE ( 'NONE', *, *, #30510, .F. ) ;
#13071=FACE_OUTER_BOUND ( 'NONE', #25681, .T. ) ;
#13080=ORIENTED_EDGE ( 'NONE', *, *, #7123, .F. ) ;
#13084=EDGE_LOOP ( 'NONE', ( #14607, #30527, #9006, #9546 ) ) ;
#13085=DIRECTION ( 'NONE',  ( 1.000000000000000000, 1.047444401652940007E-14, 0.000000000000000000 ) ) ;
#13086=EDGE_LOOP ( 'NONE', ( #11738, #8459, #23346, #22527 ) ) ;
#13091=CARTESIAN_POINT ( 'NONE',  ( 61.25000000000000000, 1.791164585742741400, 0.8897917884450912140 ) ) ;
#13093=EDGE_CURVE ( 'NONE', #6127, #7673, #13240, .T. ) ;
#13099=CARTESIAN_POINT ( 'NONE',  ( 58.65000045311386145, 1.663878723408452442, -0.8645309767532183276 ) ) ;
#13105=ADVANCED_FACE ( 'NONE', ( #5820 ), #1532, .F. ) ;
#13115=CARTESIAN_POINT ( 'NONE',  ( 58.72200624034179839, -1.875003484780597418, -0.02193204975889442854 ) ) ;
#13123=CARTESIAN_POINT ( 'NONE',  ( 52.20711756518984004, -0.4999999999994533817, -1.718465885608440269 ) ) ;
#13125=ORIENTED_EDGE ( 'NONE', *, *, #19781, .F. ) ;
#13127=DIRECTION ( 'NONE',  ( -1.000000000000000000, -1.047444401652940007E-14, -0.000000000000000000 ) ) ;
#13130=CARTESIAN_POINT ( 'NONE',  ( 58.75000000000000711, 1.066009655020737856, 1.652371589364121984 ) ) ;
#13145=VECTOR ( 'NONE', #25254, 1000.000000000000000 ) ;
#13148=CARTESIAN_POINT ( 'NONE',  ( 58.74160516400037579, -1.833004249032245347, -0.3946733352255804017 ) ) ;
#13155=CARTESIAN_POINT ( 'NONE',  ( 58.75000000000002132, 6.153735859711025284E-13, 3.111507638930570854E-58 ) ) ;
#13162=ORIENTED_EDGE ( 'NONE', *, *, #14355, .T. ) ;
#13168=( NAMED_UNIT ( * ) SI_UNIT ( $, .STERADIAN. ) SOLID_ANGLE_UNIT ( ) );
#13174=EDGE_LOOP ( 'NONE', ( #26454, #7688, #15039, #25317, #17310, #18618, #14730, #12635, #2751, #23675, #4324, #3936, #5850, #7563, #30977, #2513, #2453, #22229, #12057, #9364, #3624, #14362 ) ) ;
#13175=ORIENTED_EDGE ( 'NONE', *, *, #13315, .F. ) ;
#13176=EDGE_CURVE ( 'NONE', #12697, #10836, #5450, .T. ) ;
#13179=CARTESIAN_POINT ( 'NONE',  ( 60.88861521483853778, 0.6775725165985903020, 1.477731239195284596 ) ) ;
#13192=EDGE_LOOP ( 'NONE', ( #29984, #10547, #27388, #22018, #13666, #9356 ) ) ;
#13198=CARTESIAN_POINT ( 'NONE',  ( 58.75000000000003553, -1.320082690053552277, -1.469015551796290397 ) ) ;
#13206=DIRECTION ( 'NONE',  ( 1.000000000000000000, 1.047444401652940007E-14, 0.000000000000000000 ) ) ;
#13217=AXIS2_PLACEMENT_3D ( 'NONE', #224, #29353, #7663 ) ;
#13219=CARTESIAN_POINT ( 'NONE',  ( 58.66122331388437772, -0.5173534011631325535, 1.802520131073039433 ) ) ;
#13220=LINE ( 'NONE', #18166, #30647 ) ;
#13232=DIRECTION ( 'NONE',  ( 1.000000000000000000, 1.018631342913014973E-14, 0.000000000000000000 ) ) ;
#13240=LINE ( 'NONE', #22926, #14530 ) ;
#13243=CARTESIAN_POINT ( 'NONE',  ( 58.74154451056406856, 1.668374833164396387, -0.8556855217776168088 ) ) ;
#13249=ORIENTED_EDGE ( 'NONE', *, *, #4791, .T. ) ;
#13255=CARTESIAN_POINT ( 'NONE',  ( 58.75000000000004263, -1.972190280207336555, -0.1053114364790863067 ) ) ;
#13256=CARTESIAN_POINT ( 'NONE',  ( 58.66120520762562762, 0.4851925435088347838, 1.811135885493970976 ) ) ;
#13262=DIRECTION ( 'NONE',  ( -1.476344542015126068E-16, -0.2069455031814144141, -0.9783524716138818356 ) ) ;
#13263=DIRECTION ( 'NONE',  ( 1.000000000000000000, 1.047444401652940007E-14, 0.000000000000000000 ) ) ;
#13281=CARTESIAN_POINT ( 'NONE',  ( 58.75000000000001421, 0.5380862305915415922, -2.008165151417984351 ) ) ;
#13283=DIRECTION ( 'NONE',  ( 0.000000000000000000, 0.000000000000000000, 1.000000000000000000 ) ) ;
#13285=CARTESIAN_POINT ( 'NONE',  ( 58.75000000000004263, -1.922185811753762241, -0.4146205000034702826 ) ) ;
#13289=DIRECTION ( 'NONE',  ( -1.000000000000000000, -1.018631342913014973E-14, -0.000000000000000000 ) ) ;
#13293=CARTESIAN_POINT ( 'NONE',  ( 58.65000000000002700, -0.8495817349406442620, 1.671477153793675896 ) ) ;
#13299=CARTESIAN_POINT ( 'NONE',  ( 61.25000000000002132, 6.415596960124259844E-13, 3.111507638930570854E-58 ) ) ;
#13302=ORIENTED_EDGE ( 'NONE', *, *, #12385, .T. ) ;
#13314=CIRCLE ( 'NONE', #4736, 1.875000000000000222 ) ;
#13315=EDGE_CURVE ( 'NONE', #4931, #4841, #20110, .T. ) ;
#13323=FACE_OUTER_BOUND ( 'NONE', #7156, .T. ) ;
#13333=EDGE_CURVE ( 'NONE', #15285, #7818, #16072, .T. ) ;
#13344=AXIS2_PLACEMENT_3D ( 'NONE', #9647, #15880, #16051 ) ;
#13345=CARTESIAN_POINT ( 'NONE',  ( 58.65000000000003411, -1.571497941946429444, 1.022750809560281970 ) ) ;
#13347=CARTESIAN_POINT ( 'NONE',  ( 58.66118217212468977, -1.615348343401803666, 0.9521303665437267361 ) ) ;
#13356=CARTESIAN_POINT ( 'NONE',  ( 51.69060524974059945, -0.7995873297237187094, -1.427997211815841050 ) ) ;
#13361=CARTESIAN_POINT ( 'NONE',  ( 50.55258015808398397, 0.05176326469760456073, 1.177580158083963324 ) ) ;
#13376=TOROIDAL_SURFACE ( 'NONE', #14415, 1.975000000000001865, 0.1000000000000000056 ) ;
#13380=ORIENTED_EDGE ( 'NONE', *, *, #21037, .F. ) ;
#13390=EDGE_CURVE ( 'NONE', #28206, #12308, #4676, .T. ) ;
#13394=AXIS2_PLACEMENT_3D ( 'NONE', #7023, #25851, #11607 ) ;
#13400=CARTESIAN_POINT ( 'NONE',  ( 61.21683709729225598, 0.7974544867251615043, 1.837034727152569769 ) ) ;
#13413=AXIS2_PLACEMENT_3D ( 'NONE', #24683, #7734, #4735 ) ;
#13425=VECTOR ( 'NONE', #18778, 1000.000000000000000 ) ;
#13441=CARTESIAN_POINT ( 'NONE',  ( 50.75360625943719839, -0.3719558471739983774, -1.344678919698702124 ) ) ;
#13451=CARTESIAN_POINT ( 'NONE',  ( 51.64333574538934357, 0.8318165372350859732, 1.569663068107118198 ) ) ;
#13452=VECTOR ( 'NONE', #9865, 1000.000000000000114 ) ;
#13458=ADVANCED_FACE ( 'NONE', ( #27908 ), #11154, .T. ) ;
#13467=DIRECTION ( 'NONE',  ( 1.000000000000000000, 1.047444401652940007E-14, 0.000000000000000000 ) ) ;
#13471=AXIS2_PLACEMENT_3D ( 'NONE', #7032, #14137, #198 ) ;
#13473=EDGE_CURVE ( 'NONE', #12424, #22845, #23681, .T. ) ;
#13476=CIRCLE ( 'NONE', #31195, 0.1499999999999999667 ) ;
#13478=ORIENTED_EDGE ( 'NONE', *, *, #29535, .F. ) ;
#13484=AXIS2_PLACEMENT_3D ( 'NONE', #21641, #11647, #4516 ) ;
#13488=ADVANCED_FACE ( 'NONE', ( #11122 ), #17644, .F. ) ;
#13498=CARTESIAN_POINT ( 'NONE',  ( 58.75000000000003553, -1.652350234724367262, -1.065927491743898115 ) ) ;
#13499=AXIS2_PLACEMENT_3D ( 'NONE', #2342, #29395, #4705 ) ;
#13504=CARTESIAN_POINT ( 'NONE',  ( 51.78416995154973534, 0.8999235898787812937, -1.360374659026170718 ) ) ;
#13508=ORIENTED_EDGE ( 'NONE', *, *, #11831, .F. ) ;
#13512=CARTESIAN_POINT ( 'NONE',  ( 61.20721104068438478, 0.7580073711298901395, -1.657084523451298308 ) ) ;
#13519=CARTESIAN_POINT ( 'NONE',  ( 58.65000038048067665, -1.580579251835808829, 1.008797009995473504 ) ) ;
#13521=CARTESIAN_POINT ( 'NONE',  ( 60.87838368727346960, 0.5125281646394148627, 1.858409122016860371 ) ) ;
#13532=CARTESIAN_POINT ( 'NONE',  ( 58.74999999305994436, 1.382203543031596649, 1.345908541131239478 ) ) ;
#13537=CARTESIAN_POINT ( 'NONE',  ( 51.13341687362769505, -0.9248174436469303039, 1.495576127286106338 ) ) ;
#13542=ORIENTED_EDGE ( 'NONE', *, *, #4131, .T. ) ;
#13543=AXIS2_PLACEMENT_3D ( 'NONE', #19249, #28887, #21155 ) ;
#13552=CARTESIAN_POINT ( 'NONE',  ( 60.99999997330887425, -0.8151934526808929382, 1.407049160682770417 ) ) ;
#13559=CARTESIAN_POINT ( 'NONE',  ( 52.20711756518982583, 0.7500000000005468959, 1.718465885608440269 ) ) ;
#13563=CARTESIAN_POINT ( 'NONE',  ( 51.25000000000001421, 5.368152558471320595E-13, 3.111507638930570854E-58 ) ) ;
#13573=DIRECTION ( 'NONE',  ( 0.000000000000000000, 0.000000000000000000, 1.000000000000000000 ) ) ;
#13577=EDGE_CURVE ( 'NONE', #21772, #15123, #11904, .T. ) ;
#13578=CARTESIAN_POINT ( 'NONE',  ( 58.75000000000000711, 1.671477153794444170, 0.8495817349409561237 ) ) ;
#13579=EDGE_LOOP ( 'NONE', ( #16107, #21485, #2559, #25988 ) ) ;
#13584=AXIS2_PLACEMENT_3D ( 'NONE', #4488, #16694, #30929 ) ;
#13600=CARTESIAN_POINT ( 'NONE',  ( 61.24179192282278450, 0.9092026280841983832, -1.724287941703093630 ) ) ;
#13613=CARTESIAN_POINT ( 'NONE',  ( 58.72204580543404262, 1.816949979609431276, 0.4634803957301549260 ) ) ;
#13615=CARTESIAN_POINT ( 'NONE',  ( 51.25000000000001421, 0.9938153758931693726, -1.589954715908409755 ) ) ;
#13618=CARTESIAN_POINT ( 'NONE',  ( 58.75000000000000711, 1.655311165516932803, 1.077297519405395310 ) ) ;
#13621=B_SPLINE_CURVE_WITH_KNOTS ( 'NONE', 3,
 ( #16019, #998, #20479, #30102 ),
 .UNSPECIFIED., .F., .F.,
 ( 4, 4 ),
 ( 0.000000000000000000, 0.0003845111068534305416 ),
 .UNSPECIFIED. ) ;
#13636=ORIENTED_EDGE ( 'NONE', *, *, #5205, .F. ) ;
#13648=DIRECTION ( 'NONE',  ( 0.000000000000000000, 0.000000000000000000, 1.000000000000000000 ) ) ;
#13653=CARTESIAN_POINT ( 'NONE',  ( 50.55258015808398397, 5.295040916136730406E-13, 1.177580158083963546 ) ) ;
#13656=CARTESIAN_POINT ( 'NONE',  ( 51.11922224407864945, -0.9310536428529800901, -1.338077479437885131 ) ) ;
#13661=LINE ( 'NONE', #23343, #20388 ) ;
#13665=EDGE_CURVE ( 'NONE', #10573, #27318, #27632, .T. ) ;
#13666=ORIENTED_EDGE ( 'NONE', *, *, #28044, .T. ) ;
#13668=ORIENTED_EDGE ( 'NONE', *, *, #3153, .F. ) ;
#13669=CARTESIAN_POINT ( 'NONE',  ( 51.02976068049075309, 1.019450805965481877, -1.268081568884019017 ) ) ;
#13685=CARTESIAN_POINT ( 'NONE',  ( 58.73379417893121968, 1.381558089342225015, 1.267842757872280623 ) ) ;
#13688=DIRECTION ( 'NONE',  ( 1.000000000000000000, 1.047444401652940007E-14, 0.000000000000000000 ) ) ;
#13693=DIRECTION ( 'NONE',  ( 1.000000000000000000, 1.047444401652940007E-14, 0.000000000000000000 ) ) ;
#13695=ORIENTED_EDGE ( 'NONE', *, *, #15966, .F. ) ;
#13696=AXIS2_PLACEMENT_3D ( 'NONE', #29874, #22301, #8498 ) ;
#13699=ORIENTED_EDGE ( 'NONE', *, *, #27412, .F. ) ;
#13708=EDGE_CURVE ( 'NONE', #21736, #26230, #18372, .T. ) ;
#13710=ORIENTED_EDGE ( 'NONE', *, *, #25696, .F. ) ;
#13716=DIRECTION ( 'NONE',  ( -1.047444401652940007E-14, 1.000000000000000000, 0.000000000000000000 ) ) ;
#13723=DIRECTION ( 'NONE',  ( 0.000000000000000000, 0.5333333333333335480, -0.8459051693633012903 ) ) ;
#13725=DIRECTION ( 'NONE',  ( 0.000000000000000000, 0.9783524716136867694, -0.2069455031823359825 ) ) ;
#13727=CARTESIAN_POINT ( 'NONE',  ( 58.75000000000001421, 0.6373668173466265907, 1.895722432253563516 ) ) ;
#13729=CARTESIAN_POINT ( 'NONE',  ( 58.74999981196283727, 1.649561145038380028, 1.050519579373024426 ) ) ;
#13730=ORIENTED_EDGE ( 'NONE', *, *, #24181, .F. ) ;
#13731=AXIS2_PLACEMENT_3D ( 'NONE', #14346, #12144, #21823 ) ;
#13733=CARTESIAN_POINT ( 'NONE',  ( 58.72204580543429842, -1.309860786662360832, 1.341784641881585971 ) ) ;
#13734=EDGE_LOOP ( 'NONE', ( #24244, #31314, #19443, #9143, #11979, #5078 ) ) ;
#13736=DIRECTION ( 'NONE',  ( 0.000000000000000000, 0.000000000000000000, 1.000000000000000000 ) ) ;
#13739=CARTESIAN_POINT ( 'NONE',  ( 50.78793970012934267, -0.4223115601891286874, -0.9680023493207206009 ) ) ;
#13749=ADVANCED_FACE ( 'NONE', ( #24371 ), #15578, .F. ) ;
#13752=CARTESIAN_POINT ( 'NONE',  ( 58.75000000000000711, 1.499837071477960304, 1.323060376182421782 ) ) ;
#13759=CARTESIAN_POINT ( 'NONE',  ( 61.25000000000001421, 1.000000000000641709, -1.586072192556190474 ) ) ;
#13769=CARTESIAN_POINT ( 'NONE',  ( 50.25000000000002132, 5.314096449039845576E-13, -0.8749999999999991118 ) ) ;
#13771=EDGE_CURVE ( 'NONE', #6209, #31257, #335, .T. ) ;
#13774=ORIENTED_EDGE ( 'NONE', *, *, #28050, .T. ) ;
#13775=CARTESIAN_POINT ( 'NONE',  ( 58.75000018803716273, 1.936004331707595894, 0.04945370822498024871 ) ) ;
#13783=EDGE_CURVE ( 'NONE', #26230, #22920, #28967, .T. ) ;
#13790=B_SPLINE_CURVE_WITH_KNOTS ( 'NONE', 3,
 ( #5260, #14768, #24884, #29955, #29636, #22073 ),
 .UNSPECIFIED., .F., .F.,
 ( 4, 2, 4 ),
 ( 0.0001690239924570914956, 0.0002786457176453306390, 0.0003882674428335697553 ),
 .UNSPECIFIED. ) ;
#13793=PRESENTATION_STYLE_ASSIGNMENT (( #28234 ) ) ;
#13796=CARTESIAN_POINT ( 'NONE',  ( 58.72204580543421315, -1.635081356932600372, -0.9179489429353107077 ) ) ;
#13812=CARTESIAN_POINT ( 'NONE',  ( 51.08379317338046377, 0.8723108729837811826, -1.374656996893403038 ) ) ;
#13817=CYLINDRICAL_SURFACE ( 'NONE', #7099, 2.000000000000000000 ) ;
#13821=LINE ( 'NONE', #4509, #4653 ) ;
#13830=CARTESIAN_POINT ( 'NONE',  ( 58.66133336607585136, -1.819551968140056264, -0.4538287010057830972 ) ) ;
#13834=CARTESIAN_POINT ( 'NONE',  ( 61.24012582333646293, -0.9011229182321967013, -1.742583661751029300 ) ) ;
#13836=ORIENTED_EDGE ( 'NONE', *, *, #24181, .T. ) ;
#13840=DIRECTION ( 'NONE',  ( 0.000000000000000000, 0.000000000000000000, 1.000000000000000000 ) ) ;
#13842=ORIENTED_EDGE ( 'NONE', *, *, #23966, .T. ) ;
#13846=DIRECTION ( 'NONE',  ( 0.000000000000000000, -1.000000000000000000, 0.000000000000000000 ) ) ;
#13852=AXIS2_PLACEMENT_3D ( 'NONE', #18654, #3919, #11523 ) ;
#13853=DIRECTION ( 'NONE',  ( -1.000000000000000000, -1.047444401652940007E-14, -0.000000000000000000 ) ) ;
#13854=ORIENTED_EDGE ( 'NONE', *, *, #23992, .T. ) ;
#13860=CARTESIAN_POINT ( 'NONE',  ( 58.65844932252363009, 1.819473848874897159, -0.4532319986943835199 ) ) ;
#13868=CIRCLE ( 'NONE', #30067, 0.2500000000000000000 ) ;
#13878=DIRECTION ( 'NONE',  ( 1.000000000000000000, 1.047444401652940007E-14, 0.000000000000000000 ) ) ;
#13879=ORIENTED_EDGE ( 'NONE', *, *, #29608, .T. ) ;
#13880=CARTESIAN_POINT ( 'NONE',  ( 58.73379417893120547, 1.662624490947003153, 0.8670685180651535040 ) ) ;
#13890=CYLINDRICAL_SURFACE ( 'NONE', #4766, 0.1499999999999999667 ) ;
#13893=CARTESIAN_POINT ( 'NONE',  ( 60.99999276535461945, 0.5623636236612823414, -1.858165151419263639 ) ) ;
#13902=CARTESIAN_POINT ( 'NONE',  ( 51.23644008536124517, -1.080112125195908046, 1.214076932077873039 ) ) ;
#13905=DIRECTION ( 'NONE',  ( -1.000000000000000000, -1.047444401652940007E-14, -0.000000000000000000 ) ) ;
#13908=CARTESIAN_POINT ( 'NONE',  ( 58.65000000000003411, -1.671477153793625714, -0.8495817349401489915 ) ) ;
#13910=EDGE_CURVE ( 'NONE', #4338, #22781, #12443, .T. ) ;
#13911=EDGE_CURVE ( 'NONE', #17696, #5594, #1826, .T. ) ;
#13914=CARTESIAN_POINT ( 'NONE',  ( 58.75000000000004263, -1.877732920580616804, -0.6121634413826785304 ) ) ;
#13915=EDGE_CURVE ( 'NONE', #10186, #3598, #15802, .T. ) ;
#13920=AXIS2_PLACEMENT_3D ( 'NONE', #25959, #20910, #30877 ) ;
#13921=EDGE_LOOP ( 'NONE', ( #12198, #4894, #9757, #23347 ) ) ;
#13923=CARTESIAN_POINT ( 'NONE',  ( 58.75000000000002132, 6.153735859711025284E-13, 3.111507638930570854E-58 ) ) ;
#13924=CARTESIAN_POINT ( 'NONE',  ( 58.66118217212512320, 1.815481606355567878, 0.4689659288418223104 ) ) ;
#13933=ADVANCED_FACE ( 'NONE', ( #23256 ), #1542, .F. ) ;
#13938=DIRECTION ( 'NONE',  ( 0.000000000000000000, 0.000000000000000000, -1.000000000000000000 ) ) ;
#13943=ORIENTED_EDGE ( 'NONE', *, *, #2823, .T. ) ;
#13961=CARTESIAN_POINT ( 'NONE',  ( 58.75000018803720536, -1.651902078983118916, -1.010830333486722798 ) ) ;
#13963=CARTESIAN_POINT ( 'NONE',  ( 60.75000000000002842, -0.4999999999993638977, 1.863080903344643380 ) ) ;
#13964=ORIENTED_EDGE ( 'NONE', *, *, #23542, .T. ) ;
#13965=CARTESIAN_POINT ( 'NONE',  ( 51.08379317338048509, -0.8723108729827115937, -1.374656996893404148 ) ) ;
#13970=EDGE_CURVE ( 'NONE', #15300, #23886, #10174, .T. ) ;
#13972=VERTEX_POINT ( 'NONE', #4227 ) ;
#13983=CARTESIAN_POINT ( 'NONE',  ( 58.72204580543428420, -1.612507782425395719, 0.9570475208902531339 ) ) ;
#13986=CIRCLE ( 'NONE', #21597, 0.1500000000000001887 ) ;
#13990=EDGE_LOOP ( 'NONE', ( #6061, #18404, #18878, #1448 ) ) ;
#13991=ORIENTED_EDGE ( 'NONE', *, *, #1897, .T. ) ;
#13992=CARTESIAN_POINT ( 'NONE',  ( 52.06628335902946247, -0.5434431642975682264, -1.794517909405659806 ) ) ;
#13997=FACE_OUTER_BOUND ( 'NONE', #13192, .T. ) ;
#13998=CARTESIAN_POINT ( 'NONE',  ( 58.66054497608050866, 0.5000000000006143974, -1.807104036850122109 ) ) ;
#13999=AXIS2_PLACEMENT_3D ( 'NONE', #18326, #13232, #1066 ) ;
#14003=CARTESIAN_POINT ( 'NONE',  ( 58.65000000000001990, -0.5811678240974686993, 1.782657835994643891 ) ) ;
#14005=DIRECTION ( 'NONE',  ( 0.000000000000000000, 0.000000000000000000, -1.000000000000000000 ) ) ;
#14028=DIRECTION ( 'NONE',  ( 0.000000000000000000, 0.9507508458638780358, -0.3099561728520990322 ) ) ;
#14030=B_SPLINE_CURVE_WITH_KNOTS ( 'NONE', 3,
 ( #28894, #4983, #14635, #26507, #9886, #4814 ),
 .UNSPECIFIED., .F., .F.,
 ( 4, 2, 4 ),
 ( 2.185279341460844539E-19, 0.0001531825249253924851, 0.0003063650498507847534 ),
 .UNSPECIFIED. ) ;
#14033=CARTESIAN_POINT ( 'NONE',  ( 58.66122797211873063, 1.815363284468485716, -0.4694237433637749590 ) ) ;
#14040=DIRECTION ( 'NONE',  ( 1.000000000000000000, 1.047444401652940007E-14, 0.000000000000000000 ) ) ;
#14050=ORIENTED_EDGE ( 'NONE', *, *, #14078, .T. ) ;
#14059=CARTESIAN_POINT ( 'NONE',  ( 51.25000000000002842, -0.7499999999994634292, -1.718465885608440269 ) ) ;
#14060=CARTESIAN_POINT ( 'NONE',  ( 58.65000000000000568, 1.022750809562428476, -1.571497941946047083 ) ) ;
#14067=CARTESIAN_POINT ( 'NONE',  ( 58.74154451056417514, 0.8556855217786469847, 1.668374833163776882 ) ) ;
#14078=EDGE_CURVE ( 'NONE', #21568, #203, #2787, .T. ) ;
#14080=ORIENTED_EDGE ( 'NONE', *, *, #11304, .F. ) ;
#14086=DIRECTION ( 'NONE',  ( 0.000000000000000000, 0.000000000000000000, 1.000000000000000000 ) ) ;
#14092=DIRECTION ( 'NONE',  ( 0.000000000000000000, 0.000000000000000000, 1.000000000000000000 ) ) ;
#14100=CARTESIAN_POINT ( 'NONE',  ( 51.25000000000001421, 5.368159983410797313E-13, 3.111507638930570854E-58 ) ) ;
#14103=DIRECTION ( 'NONE',  ( 0.000000000000000000, 0.000000000000000000, 1.000000000000000000 ) ) ;
#14106=CYLINDRICAL_SURFACE ( 'NONE', #2784, 2.000000000000000000 ) ;
#14110=EDGE_CURVE ( 'NONE', #30905, #16661, #27548, .T. ) ;
#14111=CARTESIAN_POINT ( 'NONE',  ( 58.66122797211872353, 1.875002085570941057, 0.01642207461192947415 ) ) ;
#14116=EDGE_LOOP ( 'NONE', ( #9249, #31040, #16662, #25371 ) ) ;
#14119=ORIENTED_EDGE ( 'NONE', *, *, #18901, .T. ) ;
#14120=ORIENTED_EDGE ( 'NONE', *, *, #7894, .T. ) ;
#14134=AXIS2_PLACEMENT_3D ( 'NONE', #2264, #5225, #31079 ) ;
#14137=DIRECTION ( 'NONE',  ( -9.369508800225548439E-15, 0.8914544820235948963, -0.4531102586347439121 ) ) ;
#14140=FACE_OUTER_BOUND ( 'NONE', #10528, .T. ) ;
#14145=CARTESIAN_POINT ( 'NONE',  ( 51.45655683570189609, 0.9591657938401634276, 1.468576096419530019 ) ) ;
#14146=CARTESIAN_POINT ( 'NONE',  ( 58.65000000000000568, 1.571497941947157084, -1.022750809561052021 ) ) ;
#14153=ADVANCED_FACE ( 'NONE', ( #5018 ), #262, .F. ) ;
#14161=EDGE_LOOP ( 'NONE', ( #18284, #11061, #2437, #2777 ) ) ;
#14166=VERTEX_POINT ( 'NONE', #20230 ) ;
#14169=ADVANCED_FACE ( 'NONE', ( #27642 ), #10086, .F. ) ;
#14173=CARTESIAN_POINT ( 'NONE',  ( 58.74487987613210294, -0.4999999999991334154, 1.852860917433933219 ) ) ;
#14186=EDGE_LOOP ( 'NONE', ( #1362, #10313, #8183, #11426 ) ) ;
#14187=EDGE_CURVE ( 'NONE', #4841, #12697, #4361, .T. ) ;
#14192=ORIENTED_EDGE ( 'NONE', *, *, #10405, .F. ) ;
#14207=VERTEX_POINT ( 'NONE', #27176 ) ;
#14219=CARTESIAN_POINT ( 'NONE',  ( 60.75000000000002842, -0.6499999999993638644, -1.489337100860647967 ) ) ;
#14223=CARTESIAN_POINT ( 'NONE',  ( 58.72204580543412789, 0.9570475208906656928, 1.612507782426095382 ) ) ;
#14224=ORIENTED_EDGE ( 'NONE', *, *, #11181, .T. ) ;
#14230=B_SPLINE_CURVE_WITH_KNOTS ( 'NONE', 3,
 ( #6343, #21094, #23151, #28356, #16323, #1435 ),
 .UNSPECIFIED., .F., .F.,
 ( 4, 2, 4 ),
 ( 0.000000000000000000, 0.0003982002662752204356, 0.0007964005325504408712 ),
 .UNSPECIFIED. ) ;
#14232=DIRECTION ( 'NONE',  ( 0.000000000000000000, 0.000000000000000000, 1.000000000000000000 ) ) ;
#14235=ORIENTED_EDGE ( 'NONE', *, *, #25541, .F. ) ;
#14236=ADVANCED_FACE ( 'NONE', ( #10232 ), #8172, .F. ) ;
#14254=CARTESIAN_POINT ( 'NONE',  ( 58.74160516400040422, -1.784764912519645197, 0.5747049900142376933 ) ) ;
#14262=DIRECTION ( 'NONE',  ( 1.000000000000000000, 1.047444401652940007E-14, 0.000000000000000000 ) ) ;
#14264=ORIENTED_EDGE ( 'NONE', *, *, #24930, .T. ) ;
#14266=ADVANCED_FACE ( 'NONE', ( #13071 ), #5487, .T. ) ;
#14275=ORIENTED_EDGE ( 'NONE', *, *, #14187, .F. ) ;
#14281=CARTESIAN_POINT ( 'NONE',  ( 60.75000000000002842, -0.4999999999993638977, -1.863080903343643069 ) ) ;
#14286=EDGE_CURVE ( 'NONE', #27461, #27051, #27329, .T. ) ;
#14287=FACE_OUTER_BOUND ( 'NONE', #28480, .T. ) ;
#14288=CARTESIAN_POINT ( 'NONE',  ( 51.15311061045470353, -0.9578955619996478710, -1.386733222354205486 ) ) ;
#14297=DIRECTION ( 'NONE',  ( 0.000000000000000000, 0.000000000000000000, 1.000000000000000000 ) ) ;
#14299=DIRECTION ( 'NONE',  ( 1.000000000000000000, 1.047444401652940007E-14, 0.000000000000000000 ) ) ;
#14302=VERTEX_POINT ( 'NONE', #3262 ) ;
#14306=CARTESIAN_POINT ( 'NONE',  ( 50.59602332238209499, 0.1408342061609073048, 0.8215393206232031176 ) ) ;
#14311=DIRECTION ( 'NONE',  ( 0.000000000000000000, 0.000000000000000000, 1.000000000000000000 ) ) ;
#14316=CARTESIAN_POINT ( 'NONE',  ( 58.65000000000000568, 1.253243060178336643, -1.394635017528379928 ) ) ;
#14321=ADVANCED_FACE ( 'NONE', ( #3105 ), #19722, .F. ) ;
#14322=CARTESIAN_POINT ( 'NONE',  ( 51.45655683570189609, 0.9591657938401607630, 1.468576096419531130 ) ) ;
#14325=CARTESIAN_POINT ( 'NONE',  ( 58.64999999999991331, -0.6121634413825071119, -1.877732920581102638 ) ) ;
#14326=EDGE_CURVE ( 'NONE', #29298, #7417, #26111, .T. ) ;
#14331=CARTESIAN_POINT ( 'NONE',  ( 51.13989201884560742, 0.9305404255937191893, 1.499649012356343514 ) ) ;
#14332=ORIENTED_EDGE ( 'NONE', *, *, #30479, .F. ) ;
#14335=CARTESIAN_POINT ( 'NONE',  ( 52.20711756518984714, -0.7499999999994533262, -1.718465885608440713 ) ) ;
#14346=CARTESIAN_POINT ( 'NONE',  ( 58.75000000000002132, 6.153735859711025284E-13, 3.111507638930570854E-58 ) ) ;
#14355=EDGE_CURVE ( 'NONE', #17696, #19795, #20574, .T. ) ;
#14361=DIRECTION ( 'NONE',  ( 0.000000000000000000, 0.000000000000000000, 1.000000000000000000 ) ) ;
#14362=ORIENTED_EDGE ( 'NONE', *, *, #21581, .F. ) ;
#14364=VERTEX_POINT ( 'NONE', #6117 ) ;
#14367=DIRECTION ( 'NONE',  ( 1.000000000000000000, 1.047444401652940007E-14, 0.000000000000000000 ) ) ;
#14373=LINE ( 'NONE', #22625, #16586 ) ;
#14374=CARTESIAN_POINT ( 'NONE',  ( 58.74999981196283727, 0.9033020670129489060, 1.734557215428763621 ) ) ;
#14375=ORIENTED_EDGE ( 'NONE', *, *, #11479, .F. ) ;
#14383=( BOUNDED_CURVE ( )  B_SPLINE_CURVE ( 3, ( #24929, #3251, #5159, #24470 ),
 .UNSPECIFIED., .F., .T. ) 
 B_SPLINE_CURVE_WITH_KNOTS ( ( 4, 4 ),
 ( 4.050220903230332681, 4.465400561421047243 ),
 .UNSPECIFIED. ) 
 CURVE ( )  GEOMETRIC_REPRESENTATION_ITEM ( )  RATIONAL_B_SPLINE_CURVE ( ( 1.000000000000000000, 0.9856869983806465507, 0.9856869983806465507, 1.000000000000000000 ) ) 
 REPRESENTATION_ITEM ( '' )  );
#14385=B_SPLINE_CURVE_WITH_KNOTS ( 'NONE', 3,
 ( #23438, #15690, #18234, #25340, #30722, #30075 ),
 .UNSPECIFIED., .F., .F.,
 ( 4, 2, 4 ),
 ( 0.000000000000000000, 0.0001701207528151761140, 0.0003402415056303522280 ),
 .UNSPECIFIED. ) ;
#14394=CARTESIAN_POINT ( 'NONE',  ( 61.25000000000002842, -0.4999999999993586797, 1.807104036850122109 ) ) ;
#14403=CARTESIAN_POINT ( 'NONE',  ( 58.65000000000004121, -1.834410884275049947, 0.3880228184668815250 ) ) ;
#14412=EDGE_CURVE ( 'NONE', #20276, #1256, #869, .T. ) ;
#14415=AXIS2_PLACEMENT_3D ( 'NONE', #28080, #8755, #15604 ) ;
#14416=CARTESIAN_POINT ( 'NONE',  ( 58.66054497607991891, 0.5000000000007229772, 1.807104036850091910 ) ) ;
#14419=VERTEX_POINT ( 'NONE', #18628 ) ;
#14440=DIRECTION ( 'NONE',  ( 0.000000000000000000, 0.000000000000000000, 1.000000000000000000 ) ) ;
#14451=PLANE ( 'NONE',  #16490 ) ;
#14452=EDGE_CURVE ( 'NONE', #6127, #9733, #16030, .T. ) ;
#14457=ORIENTED_EDGE ( 'NONE', *, *, #1318, .T. ) ;
#14458=CIRCLE ( 'NONE', #28105, 0.2500000000000000000 ) ;
#14469=ADVANCED_FACE ( 'NONE', ( #10305 ), #2875, .T. ) ;
#14471=EDGE_LOOP ( 'NONE', ( #9325, #3381, #8678, #23118, #24949 ) ) ;
#14472=AXIS2_PLACEMENT_3D ( 'NONE', #19564, #5451, #2458 ) ;
#14475=AXIS2_PLACEMENT_3D ( 'NONE', #29860, #27948, #3263 ) ;
#14479=FACE_OUTER_BOUND ( 'NONE', #25280, .T. ) ;
#14480=DIRECTION ( 'NONE',  ( 9.599890688054003756E-15, -0.9507508458638092019, -0.3099561728523110293 ) ) ;
#14482=CARTESIAN_POINT ( 'NONE',  ( 58.65263613458528624, -0.8791532451978957274, 1.656197658588203447 ) ) ;
#14486=CARTESIAN_POINT ( 'NONE',  ( 51.43355796162960303, 0.9748468443439985975, 1.443681521171340520 ) ) ;
#14493=VECTOR ( 'NONE', #11349, 1000.000000000000000 ) ;
#14505=DIRECTION ( 'NONE',  ( -1.000000000000000000, -1.047444401652940007E-14, -0.000000000000000000 ) ) ;
#14506=ORIENTED_EDGE ( 'NONE', *, *, #3219, .F. ) ;
#14510=AXIS2_PLACEMENT_3D ( 'NONE', #2857, #7754, #22342 ) ;
#14515=AXIS2_PLACEMENT_3D ( 'NONE', #1431, #3187, #8403 ) ;
#14517=EDGE_CURVE ( 'NONE', #11262, #31243, #28302, .T. ) ;
#14524=AXIS2_PLACEMENT_3D ( 'NONE', #22591, #16941, #2371 ) ;
#14527=ORIENTED_EDGE ( 'NONE', *, *, #26060, .F. ) ;
#14528=FACE_OUTER_BOUND ( 'NONE', #1364, .T. ) ;
#14530=VECTOR ( 'NONE', #3915, 1000.000000000000000 ) ;
#14532=AXIS2_PLACEMENT_3D ( 'NONE', #26703, #26843, #2768 ) ;
#14540=CARTESIAN_POINT ( 'NONE',  ( 58.73371041428899986, 1.006219588949977650, -1.582294810366573934 ) ) ;
#14541=CARTESIAN_POINT ( 'NONE',  ( 50.25000000000000711, 1.106298139389853885, 1.666164585743605375 ) ) ;
#14550=ORIENTED_EDGE ( 'NONE', *, *, #19188, .F. ) ;
#14557=CARTESIAN_POINT ( 'NONE',  ( 52.20711756518984004, -0.4999999999994533817, 1.807104036850122109 ) ) ;
#14562=CARTESIAN_POINT ( 'NONE',  ( 58.75000000000000711, 1.469015551796267527, 1.320082690054878549 ) ) ;
#14571=CARTESIAN_POINT ( 'NONE',  ( 51.18410987668588064, 1.003361152473140505, 1.282358977530924538 ) ) ;
#14574=CARTESIAN_POINT ( 'NONE',  ( 58.65000000000000568, 1.022750809562428476, -1.571497941946047083 ) ) ;
#14575=CARTESIAN_POINT ( 'NONE',  ( 51.45655683570191741, -0.9591657938390838467, -1.611094652690527873 ) ) ;
#14581=DIRECTION ( 'NONE',  ( 7.790947421116002101E-15, -0.7438053426818020952, -0.6683962987614510132 ) ) ;
#14592=ORIENTED_EDGE ( 'NONE', *, *, #4397, .T. ) ;
#14597=DIRECTION ( 'NONE',  ( 1.000000000000000000, 1.047444401652940007E-14, 0.000000000000000000 ) ) ;
#14604=CARTESIAN_POINT ( 'NONE',  ( 52.20711756518983293, 0.6500000000005468070, 1.489337100860647967 ) ) ;
#14607=ORIENTED_EDGE ( 'NONE', *, *, #6652, .T. ) ;
#14608=CARTESIAN_POINT ( 'NONE',  ( 58.65000000000003411, -1.253243060177392953, -1.394635017528123910 ) ) ;
#14618=ORIENTED_EDGE ( 'NONE', *, *, #22032, .T. ) ;
#14620=DIRECTION ( 'NONE',  ( 1.000000000000000000, 1.047444401652940007E-14, 0.000000000000000000 ) ) ;
#14630=EDGE_CURVE ( 'NONE', #30797, #20483, #345, .T. ) ;
#14635=CARTESIAN_POINT ( 'NONE',  ( 50.55260020142765143, -0.05166409867288173502, -0.7900938592415984729 ) ) ;
#14638=B_SPLINE_CURVE_WITH_KNOTS ( 'NONE', 3,
 ( #13009, #22987, #20317, #27885, #30259, #15707 ),
 .UNSPECIFIED., .F., .F.,
 ( 4, 2, 4 ),
 ( 0.000000000000000000, 0.0001000270069606276543, 0.0002000540139212553085 ),
 .UNSPECIFIED. ) ;
#14643=CARTESIAN_POINT ( 'NONE',  ( 50.25000000000000000, 1.996089927834441946, 0.1250000000010043355 ) ) ;
#14645=DIRECTION ( 'NONE',  ( 0.000000000000000000, 0.000000000000000000, 1.000000000000000000 ) ) ;
#14649=CARTESIAN_POINT ( 'NONE',  ( 61.24794577449344501, -0.9523642485466080609, -1.677218681934459665 ) ) ;
#14667=ORIENTED_EDGE ( 'NONE', *, *, #14824, .F. ) ;
#14680=ORIENTED_EDGE ( 'NONE', *, *, #27040, .T. ) ;
#14687=CARTESIAN_POINT ( 'NONE',  ( 58.65000000000001279, 0.8495817349404606311, -1.671477153794393766 ) ) ;
#14698=FACE_OUTER_BOUND ( 'NONE', #20428, .T. ) ;
#14699=DIRECTION ( 'NONE',  ( 0.000000000000000000, 0.000000000000000000, 1.000000000000000000 ) ) ;
#14702=CARTESIAN_POINT ( 'NONE',  ( 61.24312156765933679, 0.9166010152745406314, 1.712896921566334774 ) ) ;
#14714=DIRECTION ( 'NONE',  ( 0.000000000000000000, 0.6683962987616030027, 0.7438053426816655378 ) ) ;
#14715=CARTESIAN_POINT ( 'NONE',  ( 50.25000000000000000, 1.800471618824351694, 1.039502773797588597 ) ) ;
#14718=DIRECTION ( 'NONE',  ( 0.000000000000000000, 0.000000000000000000, -1.000000000000000000 ) ) ;
#14719=CARTESIAN_POINT ( 'NONE',  ( 58.75000000000002132, 6.153735859711025284E-13, 3.111507638930570854E-58 ) ) ;
#14728=DIRECTION ( 'NONE',  ( 1.000000000000000000, 1.047444401652940007E-14, 0.000000000000000000 ) ) ;
#14730=ORIENTED_EDGE ( 'NONE', *, *, #3509, .T. ) ;
#14742=AXIS2_PLACEMENT_3D ( 'NONE', #6077, #24900, #12560 ) ;
#14752=DIRECTION ( 'NONE',  ( 0.000000000000000000, 0.000000000000000000, 1.000000000000000000 ) ) ;
#14755=LINE ( 'NONE', #2725, #22076 ) ;
#14767=ORIENTED_EDGE ( 'NONE', *, *, #9236, .T. ) ;
#14768=CARTESIAN_POINT ( 'NONE',  ( 51.27864614607251070, 1.002608958138268447, -1.395204572094401740 ) ) ;
#14783=CARTESIAN_POINT ( 'NONE',  ( 58.65838214097836811, -0.9664062014975295378, -1.606847897768189259 ) ) ;
#14789=CARTESIAN_POINT ( 'NONE',  ( 58.75000000000002132, -0.6121634413826994026, 1.877732920581024922 ) ) ;
#14790=CARTESIAN_POINT ( 'NONE',  ( 51.13585994975460380, 0.9262448312174480503, 1.518514878530177414 ) ) ;
#14794=ORIENTED_EDGE ( 'NONE', *, *, #4429, .T. ) ;
#14799=CARTESIAN_POINT ( 'NONE',  ( 50.55258015808398397, 5.295040916136730406E-13, 1.177580158083963546 ) ) ;
#14801=ORIENTED_EDGE ( 'NONE', *, *, #20532, .F. ) ;
#14808=VERTEX_POINT ( 'NONE', #4592 ) ;
#14809=CARTESIAN_POINT ( 'NONE',  ( 51.21021026411729338, -1.041641720704776786, 1.248302399389048079 ) ) ;
#14823=ORIENTED_EDGE ( 'NONE', *, *, #25376, .T. ) ;
#14824=EDGE_CURVE ( 'NONE', #1900, #3598, #28823, .T. ) ;
#14829=DIRECTION ( 'NONE',  ( 1.000000000000000000, 1.047444401652940007E-14, 0.000000000000000000 ) ) ;
#14835=ORIENTED_EDGE ( 'NONE', *, *, #3852, .T. ) ;
#14836=CARTESIAN_POINT ( 'NONE',  ( 51.59739104186227365, 1.010292945603182169, 1.272765950230260401 ) ) ;
#14842=AXIS2_PLACEMENT_3D ( 'NONE', #10711, #1662, #27959 ) ;
#14844=CIRCLE ( 'NONE', #21391, 2.000000000000000000 ) ;
#14849=EDGE_CURVE ( 'NONE', #1083, #23733, #15007, .T. ) ;
#14855=CARTESIAN_POINT ( 'NONE',  ( 58.65000000000003411, -1.077297519403678017, 1.655311165517035166 ) ) ;
#14856=CIRCLE ( 'NONE', #9322, 2.000000000000000000 ) ;
#14858=CARTESIAN_POINT ( 'NONE',  ( 61.23913277633471353, -0.8963220027428320247, 1.755758457447560428 ) ) ;
#14859=CARTESIAN_POINT ( 'NONE',  ( 58.66122389686762517, 0.5174758696803309910, 1.802487374212454307 ) ) ;
#14863=ORIENTED_EDGE ( 'NONE', *, *, #23141, .T. ) ;
#14864=DIRECTION ( 'NONE',  ( -8.860386339788720432E-15, 0.8459051693633012903, -0.5333333333333336590 ) ) ;
#14867=DIRECTION ( 'NONE',  ( 0.000000000000000000, 0.9783524716136585697, 0.2069455031824692648 ) ) ;
#14870=AXIS2_PLACEMENT_3D ( 'NONE', #7564, #2656, #22140 ) ;
#14883=EDGE_CURVE ( 'NONE', #15123, #15285, #4838, .T. ) ;
#14884=ORIENTED_EDGE ( 'NONE', *, *, #27419, .F. ) ;
#14892=DIRECTION ( 'NONE',  ( 1.000000000000000000, 1.047444401652940007E-14, 0.000000000000000000 ) ) ;
#14895=CIRCLE ( 'NONE', #15916, 0.1500000000000001887 ) ;
#14897=CARTESIAN_POINT ( 'NONE',  ( 51.85262340636811729, 0.6891204047495619323, -1.750401715244590539 ) ) ;
#14902=CARTESIAN_POINT ( 'NONE',  ( 58.65000000000003411, -1.371849028670161896, -1.278599783848962668 ) ) ;
#14927=CARTESIAN_POINT ( 'NONE',  ( 51.78364358464229156, 0.9002346248706185605, -1.360127766454892084 ) ) ;
#14929=CARTESIAN_POINT ( 'NONE',  ( 58.74999999999980815, -1.022750809560559526, -1.571497941946463861 ) ) ;
#14943=CIRCLE ( 'NONE', #13413, 0.2499999999999987788 ) ;
#14944=CIRCLE ( 'NONE', #1298, 2.000000000000000000 ) ;
#14951=ORIENTED_EDGE ( 'NONE', *, *, #30046, .F. ) ;
#14953=EDGE_LOOP ( 'NONE', ( #19269, #29505, #10799, #29270 ) ) ;
#14961=ORIENTED_EDGE ( 'NONE', *, *, #23787, .F. ) ;
#14977=AXIS2_PLACEMENT_3D ( 'NONE', #15139, #20066, #5968 ) ;
#14980=CIRCLE ( 'NONE', #3355, 0.2500000000000000000 ) ;
#14983=CARTESIAN_POINT ( 'NONE',  ( 58.75000000000003553, -1.470078920827206925, -1.470078920827526892 ) ) ;
#14988=ORIENTED_EDGE ( 'NONE', *, *, #15227, .F. ) ;
#14994=ADVANCED_FACE ( 'NONE', ( #6155 ), #10887, .F. ) ;
#14996=CIRCLE ( 'NONE', #9950, 1.875000000000001776 ) ;
#14998=CIRCLE ( 'NONE', #17038, 1.875000000000001776 ) ;
#15007=CIRCLE ( 'NONE', #1356, 0.1000000000000000194 ) ;
#15023=CYLINDRICAL_SURFACE ( 'NONE', #30606, 0.1500000000000001887 ) ;
#15026=FACE_OUTER_BOUND ( 'NONE', #3605, .T. ) ;
#15030=DIRECTION ( 'NONE',  ( 1.000000000000000000, 1.047444401652940007E-14, -0.000000000000000000 ) ) ;
#15036=CARTESIAN_POINT ( 'NONE',  ( 58.71354657862850246, -0.4999999999993852695, -1.821913688936154241 ) ) ;
#15039=ORIENTED_EDGE ( 'NONE', *, *, #25043, .T. ) ;
#15046=DIRECTION ( 'NONE',  ( 0.000000000000000000, 0.000000000000000000, 1.000000000000000000 ) ) ;
#15056=VECTOR ( 'NONE', #14505, 1000.000000000000000 ) ;
#15062=CARTESIAN_POINT ( 'NONE',  ( 58.75000000000002132, 6.153735859711025284E-13, 3.111507638930570854E-58 ) ) ;
#15066=LINE ( 'NONE', #7633, #23117 ) ;
#15070=ORIENTED_EDGE ( 'NONE', *, *, #28524, .T. ) ;
#15074=CARTESIAN_POINT ( 'NONE',  ( 51.32028027175453389, -1.012964966966786617, -1.577985093213079448 ) ) ;
#15077=ADVANCED_FACE ( 'NONE', ( #26549 ), #9775, .F. ) ;
#15079=CARTESIAN_POINT ( 'NONE',  ( 58.75000000000004263, -2.008165151418633165, 0.5380862305909606125 ) ) ;
#15092=CARTESIAN_POINT ( 'NONE',  ( 61.16864364483389238, -0.7080009476652142641, -1.871974308544436250 ) ) ;
#15097=CARTESIAN_POINT ( 'NONE',  ( 51.50435016707358216, 0.9265794315412900772, -1.339215852266870233 ) ) ;
#15099=CARTESIAN_POINT ( 'NONE',  ( 60.94140446608462014, 0.5380862305989584371, -1.858165151370887669 ) ) ;
#15101=CARTESIAN_POINT ( 'NONE',  ( 51.14630318392405428, 0.9364487020640391846, 1.503522130792586342 ) ) ;
#15105=CARTESIAN_POINT ( 'NONE',  ( 58.75000000000003553, -1.666164585742487159, -1.106298139390194724 ) ) ;
#15111=EDGE_CURVE ( 'NONE', #15962, #2126, #28112, .T. ) ;
#15114=VERTEX_POINT ( 'NONE', #29086 ) ;
#15116=CYLINDRICAL_SURFACE ( 'NONE', #243, 0.1500000000000001887 ) ;
#15121=ORIENTED_EDGE ( 'NONE', *, *, #25059, .F. ) ;
#15123=VERTEX_POINT ( 'NONE', #26403 ) ;
#15139=CARTESIAN_POINT ( 'NONE',  ( 60.75000000000003553, -0.9999999999993638422, -1.996089927833914146 ) ) ;
#15144=CARTESIAN_POINT ( 'NONE',  ( 51.13585994975462512, -0.9262448312163767961, 1.518514878530177192 ) ) ;
#15146=DIRECTION ( 'NONE',  ( 1.000000000000000000, 1.047444401652940007E-14, 0.000000000000000000 ) ) ;
#15147=CARTESIAN_POINT ( 'NONE',  ( 51.34893360928146677, -1.002183861492330630, -1.396106892655424980 ) ) ;
#15156=CARTESIAN_POINT ( 'NONE',  ( 58.65000000000000568, 0.9941784314380587295, 1.590093208333443142 ) ) ;
#15158=ORIENTED_EDGE ( 'NONE', *, *, #24286, .F. ) ;
#15159=CARTESIAN_POINT ( 'NONE',  ( 58.75000000000003553, -1.972190280207336555, 0.1053114364790900953 ) ) ;
#15161=CIRCLE ( 'NONE', #23768, 0.1499999999999998557 ) ;
#15174=CARTESIAN_POINT ( 'NONE',  ( 51.25000000000002842, -1.099999999999459410, -1.001327244211406953 ) ) ;
#15177=ORIENTED_EDGE ( 'NONE', *, *, #9051, .T. ) ;
#15184=CARTESIAN_POINT ( 'NONE',  ( 58.74154451056425330, -1.872697749442759463, -0.09314201707011884879 ) ) ;
#15185=AXIS2_PLACEMENT_3D ( 'NONE', #29238, #17063, #19597 ) ;
#15187=ORIENTED_EDGE ( 'NONE', *, *, #29061, .T. ) ;
#15189=VERTEX_POINT ( 'NONE', #12755 ) ;
#15199=CARTESIAN_POINT ( 'NONE',  ( 51.59739104186226655, 1.010292945603183723, 1.272765950230259513 ) ) ;
#15206=ADVANCED_FACE ( 'NONE', ( #17527 ), #25270, .T. ) ;
#15219=DIRECTION ( 'NONE',  ( 1.000000000000000000, 1.047444401652940007E-14, 0.000000000000000000 ) ) ;
#15222=CARTESIAN_POINT ( 'NONE',  ( 51.21562071718019382, 0.9844478935114779894, -1.555267182539685100 ) ) ;
#15227=EDGE_CURVE ( 'NONE', #9733, #10205, #6374, .T. ) ;
#15244=CARTESIAN_POINT ( 'NONE',  ( 60.75000000000002842, -0.6499999999993638644, 1.489337100860647967 ) ) ;
#15246=EDGE_LOOP ( 'NONE', ( #2899, #23391, #16407, #1625 ) ) ;
#15252=CIRCLE ( 'NONE', #2093, 0.8749999999999990008 ) ;
#15255=CARTESIAN_POINT ( 'NONE',  ( 50.25000000000003553, -1.323060376181184772, -1.499837071478052453 ) ) ;
#15261=DIRECTION ( 'NONE',  ( 0.000000000000000000, 0.000000000000000000, 1.000000000000000000 ) ) ;
#15264=CARTESIAN_POINT ( 'NONE',  ( 58.66122797211878748, 1.337438849765252069, -1.314214529126763509 ) ) ;
#15269=EDGE_LOOP ( 'NONE', ( #13879, #17315, #3737, #14192 ) ) ;
#15271=VERTEX_POINT ( 'NONE', #30328 ) ;
#15272=CARTESIAN_POINT ( 'NONE',  ( 50.25000000000003553, -1.470078920827295965, -1.470078920827526892 ) ) ;
#15280=CARTESIAN_POINT ( 'NONE',  ( 51.40674769956036272, 0.9873535814804794697, -1.422142864483640912 ) ) ;
#15285=VERTEX_POINT ( 'NONE', #25892 ) ;
#15295=CARTESIAN_POINT ( 'NONE',  ( 58.65000000000004121, -1.760622601995821990, 0.8948927608039443093 ) ) ;
#15299=AXIS2_PLACEMENT_3D ( 'NONE', #18256, #31012, #22999 ) ;
#15300=VERTEX_POINT ( 'NONE', #11654 ) ;
#15307=VERTEX_POINT ( 'NONE', #8778 ) ;
#15308=CARTESIAN_POINT ( 'NONE',  ( 60.75000000000001421, 0.7500000000006363798, 1.718465885608440269 ) ) ;
#15313=DIRECTION ( 'NONE',  ( 0.7542528389311653481, 0.5142632992712595774, -0.4082106245394850341 ) ) ;
#15314=LINE ( 'NONE', #24959, #6960 ) ;
#15333=DIRECTION ( 'NONE',  ( -0.7542528389311761172, 0.5142632992712440343, 0.4082106245394852007 ) ) ;
#15342=CARTESIAN_POINT ( 'NONE',  ( 58.75000000000003553, -1.320164791810108484, 1.457351493770938200 ) ) ;
#15366=CARTESIAN_POINT ( 'NONE',  ( 58.72427158855730056, -1.822388627306549047, -0.4415141953928994889 ) ) ;
#15369=FACE_OUTER_BOUND ( 'NONE', #21926, .T. ) ;
#15371=CARTESIAN_POINT ( 'NONE',  ( 58.66133336607634163, 1.802692578419500258, -0.5167488000321581731 ) ) ;
#15376=CARTESIAN_POINT ( 'NONE',  ( 58.64999999999992752, -1.760622601995799119, -0.8948927608040211368 ) ) ;
#15380=ORIENTED_EDGE ( 'NONE', *, *, #2618, .F. ) ;
#15381=CARTESIAN_POINT ( 'NONE',  ( 60.75000000000002842, -0.4999999999993638977, 1.718465885608440047 ) ) ;
#15386=ORIENTED_EDGE ( 'NONE', *, *, #6553, .F. ) ;
#15387=ADVANCED_FACE ( 'NONE', ( #12262 ), #30143, .F. ) ;
#15392=CARTESIAN_POINT ( 'NONE',  ( 51.34430644926990084, 1.002608958138277773, -1.395204572094386641 ) ) ;
#15407=ADVANCED_FACE ( 'NONE', ( #29214 ), #25979, .T. ) ;
#15413=AXIS2_PLACEMENT_3D ( 'NONE', #20249, #15313, #10251 ) ;
#15416=DIRECTION ( 'NONE',  ( 0.000000000000000000, 0.000000000000000000, 1.000000000000000000 ) ) ;
#15418=EDGE_CURVE ( 'NONE', #10721, #1900, #28627, .T. ) ;
#15428=EDGE_CURVE ( 'NONE', #12125, #28052, #8597, .T. ) ;
#15433=CARTESIAN_POINT ( 'NONE',  ( 51.25000000000001421, 0.9938153758931693726, -1.589954715908409755 ) ) ;
#15434=ORIENTED_EDGE ( 'NONE', *, *, #12487, .T. ) ;
#15437=ORIENTED_EDGE ( 'NONE', *, *, #23209, .F. ) ;
#15454=VECTOR ( 'NONE', #20463, 1000.000000000000000 ) ;
#15455=DIRECTION ( 'NONE',  ( 0.000000000000000000, 1.000000000000000000, 0.000000000000000000 ) ) ;
#15460=AXIS2_PLACEMENT_3D ( 'NONE', #11269, #23800, #28708 ) ;
#15464=AXIS2_PLACEMENT_3D ( 'NONE', #30034, #6000, #6291 ) ;
#15471=CARTESIAN_POINT ( 'NONE',  ( 58.75000000000002842, -1.077297519403677128, 1.655311165517035166 ) ) ;
#15480=ORIENTED_EDGE ( 'NONE', *, *, #3003, .F. ) ;
#15484=CARTESIAN_POINT ( 'NONE',  ( 58.65266784251163301, 1.656109637136700785, -0.8793208749727724483 ) ) ;
#15485=AXIS2_PLACEMENT_3D ( 'NONE', #9195, #11570, #8850 ) ;
#15488=CARTESIAN_POINT ( 'NONE',  ( 52.10126625705173353, -0.5195911883732942105, 1.546252172343134834 ) ) ;
#15501=DIRECTION ( 'NONE',  ( -0.5633368246414944824, -0.8262273428075580517, 0.000000000000000000 ) ) ;
#15505=CIRCLE ( 'NONE', #14515, 1.875000000000001776 ) ;
#15519=AXIS2_PLACEMENT_3D ( 'NONE', #5609, #6080, #3225 ) ;
#15525=DIRECTION ( 'NONE',  ( 0.000000000000000000, 0.000000000000000000, 1.000000000000000000 ) ) ;
#15527=VECTOR ( 'NONE', #12344, 1000.000000000000000 ) ;
#15529=CIRCLE ( 'NONE', #5926, 0.1500000000000001887 ) ;
#15537=CIRCLE ( 'NONE', #3923, 0.1000000000000001027 ) ;
#15538=DIRECTION ( 'NONE',  ( 0.000000000000000000, 0.000000000000000000, -1.000000000000000000 ) ) ;
#15539=DIRECTION ( 'NONE',  ( 1.000000000000000000, 1.047444401652940007E-14, 0.000000000000000000 ) ) ;
#15542=DIRECTION ( 'NONE',  ( 1.000000000000000000, 1.047444401652940007E-14, 0.000000000000000000 ) ) ;
#15549=CARTESIAN_POINT ( 'NONE',  ( 51.45655683570191741, -0.9591657938390838467, -1.611094652690527873 ) ) ;
#15552=VERTEX_POINT ( 'NONE', #24606 ) ;
#15559=FACE_OUTER_BOUND ( 'NONE', #24995, .T. ) ;
#15565=SURFACE_STYLE_USAGE ( .BOTH. , #22236 ) ;
#15567=CIRCLE ( 'NONE', #20645, 0.1000000000000000056 ) ;
#15574=EDGE_CURVE ( 'NONE', #14364, #5594, #27601, .T. ) ;
#15578=TOROIDAL_SURFACE ( 'NONE', #12953, 1.975000000000001865, 0.1000000000000000056 ) ;
#15581=VECTOR ( 'NONE', #6877, 1000.000000000000000 ) ;
#15583=DIRECTION ( 'NONE',  ( -1.000000000000000000, -1.047444401652940007E-14, -0.000000000000000000 ) ) ;
#15588=CARTESIAN_POINT ( 'NONE',  ( 58.65266784251157617, 1.372094080477309186, -1.277991457600056391 ) ) ;
#15592=DIRECTION ( 'NONE',  ( 1.000000000000000000, 1.047444401652940007E-14, 0.000000000000000000 ) ) ;
#15595=EDGE_LOOP ( 'NONE', ( #25780, #17205, #4837, #16174 ) ) ;
#15603=VECTOR ( 'NONE', #12648, 1000.000000000000000 ) ;
#15604=DIRECTION ( 'NONE',  ( 0.000000000000000000, 0.000000000000000000, 1.000000000000000000 ) ) ;
#15605=ORIENTED_EDGE ( 'NONE', *, *, #20222, .T. ) ;
#15608=CARTESIAN_POINT ( 'NONE',  ( 60.75000000000001421, 0.5000000000006363798, 1.863080903344386030 ) ) ;
#15609=MANIFOLD_SOLID_BREP ( 'Stock-MAS-683-1', #16029 ) ;
#15619=CARTESIAN_POINT ( 'NONE',  ( 58.75000018803716983, 1.333992738916855325, 1.403930843797372541 ) ) ;
#15621=CARTESIAN_POINT ( 'NONE',  ( 58.72200959573710577, -0.5298027519206366387, 1.799185603788605148 ) ) ;
#15623=CARTESIAN_POINT ( 'NONE',  ( 58.75000000000002132, 6.153735859711025284E-13, 3.111507638930570854E-58 ) ) ;
#15627=CARTESIAN_POINT ( 'NONE',  ( 51.25000000000002842, -1.099999999999462963, -1.996089927833914146 ) ) ;
#15628=AXIS2_PLACEMENT_3D ( 'NONE', #11362, #18981, #30512 ) ;
#15639=CARTESIAN_POINT ( 'NONE',  ( 61.25000000000000711, 1.470078920828170821, -1.470078920826818125 ) ) ;
#15642=CARTESIAN_POINT ( 'NONE',  ( 61.16289782575152145, -0.6851579758920108842, -1.477831714898571347 ) ) ;
#15665=CARTESIAN_POINT ( 'NONE',  ( 58.74999999305998699, -1.929066554547878454, 0.02566444196692819688 ) ) ;
#15669=AXIS2_PLACEMENT_3D ( 'NONE', #27399, #6187, #30391 ) ;
#15690=CARTESIAN_POINT ( 'NONE',  ( 51.13996726386383784, 0.9386186536674969716, -1.439073407537156069 ) ) ;
#15696=CYLINDRICAL_SURFACE ( 'NONE', #19109, 0.2500000000000000000 ) ;
#15697=LINE ( 'NONE', #11091, #28079 ) ;
#15698=CARTESIAN_POINT ( 'NONE',  ( 51.25000000000001421, 1.100000000000534994, -1.001327244211404732 ) ) ;
#15699=DIRECTION ( 'NONE',  ( 0.000000000000000000, 0.000000000000000000, 1.000000000000000000 ) ) ;
#15703=DIRECTION ( 'NONE',  ( 0.000000000000000000, 0.000000000000000000, 1.000000000000000000 ) ) ;
#15706=CARTESIAN_POINT ( 'NONE',  ( 58.75000018595668649, 1.883137918660746202, 0.4528999722754235568 ) ) ;
#15707=CARTESIAN_POINT ( 'NONE',  ( 58.65000000000003411, -1.022750809560713181, -1.571497941946363497 ) ) ;
#15708=FACE_OUTER_BOUND ( 'NONE', #25517, .T. ) ;
#15727=CARTESIAN_POINT ( 'NONE',  ( 61.22059884411343234, 0.7794434480088445749, 1.429589005548685954 ) ) ;
#15731=ADVANCED_FACE ( 'NONE', ( #14287 ), #29010, .F. ) ;
#15733=CYLINDRICAL_SURFACE ( 'NONE', #4807, 0.1500000000000001887 ) ;
#15737=CARTESIAN_POINT ( 'NONE',  ( 58.74999981404334903, -1.734728236458829453, -0.9032433253517498928 ) ) ;
#15742=EDGE_CURVE ( 'NONE', #24661, #22181, #29233, .T. ) ;
#15744=DIRECTION ( 'NONE',  ( 1.000000000000000000, 1.047444401652940007E-14, 0.000000000000000000 ) ) ;
#15745=DIRECTION ( 'NONE',  ( 1.000000000000000000, 1.047444401652940007E-14, 0.000000000000000000 ) ) ;
#15757=CARTESIAN_POINT ( 'NONE',  ( 61.25000000000003553, -1.323060376181777631, 1.499837071478349326 ) ) ;
#15758=CARTESIAN_POINT ( 'NONE',  ( 58.75000000000001421, 0.6121634413844196931, -1.877732920580865272 ) ) ;
#15761=CARTESIAN_POINT ( 'NONE',  ( 52.20711756518984714, -0.7499999999994533262, 1.718465885608439825 ) ) ;
#15764=CARTESIAN_POINT ( 'NONE',  ( 58.65266784251148380, 1.277991457600490932, 1.372094080476860878 ) ) ;
#15769=CARTESIAN_POINT ( 'NONE',  ( 58.75000000000000000, 2.008165151418601191, 0.5380862305919300592 ) ) ;
#15794=DIRECTION ( 'NONE',  ( 1.000000000000000000, 1.047444401652940007E-14, 0.000000000000000000 ) ) ;
#15799=DIRECTION ( 'NONE',  ( 0.000000000000000000, 0.000000000000000000, 1.000000000000000000 ) ) ;
#15802=LINE ( 'NONE', #16424, #14493 ) ;
#15809=CARTESIAN_POINT ( 'NONE',  ( 58.65838214097815495, -1.874774200233337185, 0.03350837198770668934 ) ) ;
#15821=CARTESIAN_POINT ( 'NONE',  ( 58.75000000000000711, 1.077297519403823234, 1.655311165517741268 ) ) ;
#15838=AXIS2_PLACEMENT_3D ( 'NONE', #27376, #15030, #773 ) ;
#15845=CARTESIAN_POINT ( 'NONE',  ( 58.65266784251149801, 1.792820108340006602, 0.5492726012753877951 ) ) ;
#15847=DIRECTION ( 'NONE',  ( 1.000000000000000000, 1.047444401652940007E-14, -0.000000000000000000 ) ) ;
#15851=ORIENTED_EDGE ( 'NONE', *, *, #27559, .F. ) ;
#15852=CARTESIAN_POINT ( 'NONE',  ( 50.59602332238209499, 0.1408342061609076379, -0.8215393206232032286 ) ) ;
#15856=CARTESIAN_POINT ( 'NONE',  ( 51.24099374247646921, -1.086790822298242087, -1.208135181987622486 ) ) ;
#15859=EDGE_CURVE ( 'NONE', #6367, #7461, #3112, .T. ) ;
#15864=ADVANCED_FACE ( 'NONE', ( #17442 ), #5572, .F. ) ;
#15867=VERTEX_POINT ( 'NONE', #27407 ) ;
#15872=EDGE_CURVE ( 'NONE', #21960, #11981, #15066, .T. ) ;
#15874=CARTESIAN_POINT ( 'NONE',  ( 61.00000000000002842, -0.8666666666660278739, -1.374595900215364708 ) ) ;
#15880=DIRECTION ( 'NONE',  ( 1.000000000000000000, 1.047444401652940007E-14, 0.000000000000000000 ) ) ;
#15891=EDGE_CURVE ( 'NONE', #27521, #14166, #12968, .T. ) ;
#15892=FACE_OUTER_BOUND ( 'NONE', #28032, .T. ) ;
#15895=CARTESIAN_POINT ( 'NONE',  ( 51.25000000000002842, -0.7499999999994634292, 1.718465885608440269 ) ) ;
#15903=CARTESIAN_POINT ( 'NONE',  ( 51.31572262954149011, 1.002608958138273554, -1.395204572094392637 ) ) ;
#15910=CARTESIAN_POINT ( 'NONE',  ( 52.20711756518984714, -0.7499999999994533262, 1.718465885608439603 ) ) ;
#15916=AXIS2_PLACEMENT_3D ( 'NONE', #23220, #25739, #18467 ) ;
#15917=DIRECTION ( 'NONE',  ( 9.329605248950888974E-15, -1.000000000000000000, 0.000000000000000000 ) ) ;
#15918=ORIENTED_EDGE ( 'NONE', *, *, #19908, .F. ) ;
#15922=AXIS2_PLACEMENT_3D ( 'NONE', #3569, #8304, #17972 ) ;
#15924=CARTESIAN_POINT ( 'NONE',  ( 61.25000000000003553, -0.9999999999993586242, 1.586072192556190252 ) ) ;
#15929=ADVANCED_FACE ( 'NONE', ( #15369 ), #24722, .F. ) ;
#15930=B_SPLINE_CURVE_WITH_KNOTS ( 'NONE', 3,
 ( #28971, #16949, #24231, #20846, #10852, #27951 ),
 .UNSPECIFIED., .F., .F.,
 ( 4, 2, 4 ),
 ( 0.000000000000000000, 0.0001000270069604649562, 0.0002000540139209299123 ),
 .UNSPECIFIED. ) ;
#15937=ORIENTED_EDGE ( 'NONE', *, *, #7484, .T. ) ;
#15939=DIRECTION ( 'NONE',  ( 0.000000000000000000, 0.000000000000000000, 1.000000000000000000 ) ) ;
#15951=( BOUNDED_CURVE ( )  B_SPLINE_CURVE ( 3, ( #27575, #30269, #15856, #1288 ),
 .UNSPECIFIED., .F., .T. ) 
 B_SPLINE_CURVE_WITH_KNOTS ( ( 4, 4 ),
 ( 0.8272220676012502771, 0.8437250283369835957 ),
 .UNSPECIFIED. ) 
 CURVE ( )  GEOMETRIC_REPRESENTATION_ITEM ( )  RATIONAL_B_SPLINE_CURVE ( ( 1.000000000000000000, 0.9999773044860189586, 0.9999773044860189586, 1.000000000000000000 ) ) 
 REPRESENTATION_ITEM ( '' )  );
#15954=FACE_OUTER_BOUND ( 'NONE', #18876, .T. ) ;
#15958=ORIENTED_EDGE ( 'NONE', *, *, #17729, .T. ) ;
#15959=CARTESIAN_POINT ( 'NONE',  ( 58.66054497608050866, 0.5000000000006143974, -1.807104036850122109 ) ) ;
#15962=VERTEX_POINT ( 'NONE', #10020 ) ;
#15966=EDGE_CURVE ( 'NONE', #30566, #11854, #4389, .T. ) ;
#15969=CARTESIAN_POINT ( 'NONE',  ( 58.75000000000000711, 1.877732920581777432, -0.6121634413828938026 ) ) ;
#15983=AXIS2_PLACEMENT_3D ( 'NONE', #16182, #4138, #13725 ) ;
#15993=( GEOMETRIC_REPRESENTATION_CONTEXT ( 3 ) GLOBAL_UNCERTAINTY_ASSIGNED_CONTEXT ( ( #10746 ) ) GLOBAL_UNIT_ASSIGNED_CONTEXT ( ( #30587, #16354, #6693 ) ) REPRESENTATION_CONTEXT ( 'NONE', 'WORKASPACE' ) );
#16004=CARTESIAN_POINT ( 'NONE',  ( 58.72427158855717266, 1.822388627307728992, 0.4415141953931043806 ) ) ;
#16007=ORIENTED_EDGE ( 'NONE', *, *, #13390, .T. ) ;
#16012=ADVANCED_FACE ( 'NONE', ( #16286 ), #8431, .F. ) ;
#16019=CARTESIAN_POINT ( 'NONE',  ( 51.23644008536121675, 1.080112125196981410, -1.214076932077873039 ) ) ;
#16021=CIRCLE ( 'NONE', #24634, 0.09999999999999988065 ) ;
#16024=ORIENTED_EDGE ( 'NONE', *, *, #26043, .T. ) ;
#16027=VERTEX_POINT ( 'NONE', #1124 ) ;
#16029=CLOSED_SHELL ( 'NONE', ( #13105, #17637, #28536, #7296, #17786, #15864, #5037, #16796, #22012, #6728, #26848, #22163, #16610, #14153, #10774, #16954, #27871, #18136, #17941, #17632, #25251, #4508, #9278, #28956, #16440, #17307, #15929, #370, #15731, #2142, #18955, #12954, #20686, #16961, #19304, #25408, #30123, #28376, #13933, #1201, #25373, #443, #599, #23446, #25387, #30262, #14469, #15206, #21231, #30060, #24373, #29944, #10963, #17815, #30474, #5288, #19726, #16999, #20462, #5475, #12964, #11658, #25309, #23711, #21065, #6489, #23645, #7550, #21078, #2649, #14169, #14236, #18243, #30710, #1985, #2139, #24133, #28168, #18470, #12169, #939, #17809, #9312, #18025, #30096, #14994, #13488, #25803, #11798, #4585, #29633, #1908, #16012, #4853, #217, #24700, #30987, #15387, #835, #284, #11589, #25978, #906, #18317, #3668, #25410, #3284, #10753, #22769, #17879, #29337, #20638, #18416, #13749, #20832, #6475, #11211, #7327, #9093, #11730, #20418, #9049, #12748, #17749, #25947, #17686, #27981, #14321, #892, #26752, #16380, #24478, #923, #9776, #4911, #2503, #29937, #27303, #16050, #14266, #30198, #3290, #24425, #23566, #7895, #1114, #17844, #17362, #15077, #26418, #26783, #22200, #29000, #16199, #29973, #4643, #22220, #16229, #29882, #30890, #16109, #1725, #19149, #15407, #5309, #30671, #12227, #13458, #9611, #23850, #6215, #30503, #8745, #6415 ) ) ;
#16030=CIRCLE ( 'NONE', #17479, 0.1500000000000001887 ) ;
#16046=DIRECTION ( 'NONE',  ( 0.000000000000000000, 0.000000000000000000, 1.000000000000000000 ) ) ;
#16048=AXIS2_PLACEMENT_3D ( 'NONE', #19233, #18318, #4790 ) ;
#16050=ADVANCED_FACE ( 'NONE', ( #28469 ), #6771, .T. ) ;
#16051=DIRECTION ( 'NONE',  ( 0.000000000000000000, 0.000000000000000000, 1.000000000000000000 ) ) ;
#16052=VERTEX_POINT ( 'NONE', #15698 ) ;
#16060=CARTESIAN_POINT ( 'NONE',  ( 51.27141371434416328, 0.9996500697957936277, 1.586307688445277586 ) ) ;
#16065=CARTESIAN_POINT ( 'NONE',  ( 58.75000000000002842, -1.077297519403983106, -1.655311165516836436 ) ) ;
#16066=VERTEX_POINT ( 'NONE', #30083 ) ;
#16067=CARTESIAN_POINT ( 'NONE',  ( 58.72419296898096519, -1.645806614394166534, 0.8985315506029413202 ) ) ;
#16072=CIRCLE ( 'NONE', #29711, 0.2499999999999987788 ) ;
#16076=AXIS2_PLACEMENT_3D ( 'NONE', #4882, #23748, #2040 ) ;
#16081=CARTESIAN_POINT ( 'NONE',  ( 51.25879181974310939, -0.9981351195451134695, 1.403212705160382212 ) ) ;
#16085=DIRECTION ( 'NONE',  ( 1.000000000000000000, 1.047444401652940007E-14, 0.000000000000000000 ) ) ;
#16088=B_SPLINE_CURVE_WITH_KNOTS ( 'NONE', 3,
 ( #14557, #26430, #24222, #16786 ),
 .UNSPECIFIED., .F., .F.,
 ( 4, 4 ),
 ( 0.000000000000000000, 0.0001493943817025057165 ),
 .UNSPECIFIED. ) ;
#16093=PLANE ( 'NONE',  #20123 ) ;
#16094=CARTESIAN_POINT ( 'NONE',  ( 58.75000000000000711, 1.320082690053780983, 1.469015551797191010 ) ) ;
#16097=TOROIDAL_SURFACE ( 'NONE', #13543, 1.975000000000001865, 0.1000000000000000056 ) ;
#16098=EDGE_LOOP ( 'NONE', ( #21278, #16131, #29904, #14235 ) ) ;
#16099=CARTESIAN_POINT ( 'NONE',  ( 58.75000000000002132, 6.153735859711025284E-13, 3.111507638930570854E-58 ) ) ;
#16104=CARTESIAN_POINT ( 'NONE',  ( 58.75000000000000711, 1.077297519403823678, 1.655311165517741490 ) ) ;
#16107=ORIENTED_EDGE ( 'NONE', *, *, #10869, .T. ) ;
#16109=ADVANCED_FACE ( 'NONE', ( #19786 ), #20105, .T. ) ;
#16119=LINE ( 'NONE', #21202, #93 ) ;
#16121=CIRCLE ( 'NONE', #24217, 0.2500000000000000000 ) ;
#16123=AXIS2_PLACEMENT_3D ( 'NONE', #29750, #15333, #15501 ) ;
#16124=DIRECTION ( 'NONE',  ( 1.000000000000000000, 1.047444401652940007E-14, 0.000000000000000000 ) ) ;
#16131=ORIENTED_EDGE ( 'NONE', *, *, #19611, .F. ) ;
#16132=CARTESIAN_POINT ( 'NONE',  ( 58.75000000000000711, 1.749377236609743091, 0.8979909453705852140 ) ) ;
#16137=VERTEX_POINT ( 'NONE', #10118 ) ;
#16139=CARTESIAN_POINT ( 'NONE',  ( 51.25000000000001421, 1.100000000000534994, 1.001327244211404732 ) ) ;
#16141=EDGE_CURVE ( 'NONE', #27455, #6127, #3816, .T. ) ;
#16142=CARTESIAN_POINT ( 'NONE',  ( 51.01608411450972369, -0.7569233679470201981, -1.030722644926826526 ) ) ;
#16144=DIRECTION ( 'NONE',  ( 1.000000000000000000, 1.047444401652940007E-14, 0.000000000000000000 ) ) ;
#16154=CARTESIAN_POINT ( 'NONE',  ( 61.23787131559241459, 0.8905369330983690102, -1.779178344869518202 ) ) ;
#16160=EDGE_CURVE ( 'NONE', #23063, #2126, #30463, .T. ) ;
#16166=CARTESIAN_POINT ( 'NONE',  ( 61.25000000000002132, 6.415596960124259844E-13, 3.111507638930570854E-58 ) ) ;
#16167=DIRECTION ( 'NONE',  ( 1.000000000000000000, 1.047444401652940007E-14, 0.000000000000000000 ) ) ;
#16168=ORIENTED_EDGE ( 'NONE', *, *, #16650, .T. ) ;
#16169=CYLINDRICAL_SURFACE ( 'NONE', #1268, 2.000000000000000000 ) ;
#16171=CARTESIAN_POINT ( 'NONE',  ( 58.75000000000000000, 1.922185811755142915, 0.4146205000036791710 ) ) ;
#16174=ORIENTED_EDGE ( 'NONE', *, *, #5998, .F. ) ;
#16182=CARTESIAN_POINT ( 'NONE',  ( 58.65000000000004121, -1.932246131436418768, 0.4087173687851147208 ) ) ;
#16188=ORIENTED_EDGE ( 'NONE', *, *, #26976, .F. ) ;
#16197=CARTESIAN_POINT ( 'NONE',  ( 58.75000000000000711, 1.470078920828144620, -1.470078920826818125 ) ) ;
#16199=ADVANCED_FACE ( 'NONE', ( #19936 ), #30592, .T. ) ;
#16207=CARTESIAN_POINT ( 'NONE',  ( 58.72419296898085150, -1.601054456120828640, -0.9760445624807464471 ) ) ;
#16220=ORIENTED_EDGE ( 'NONE', *, *, #28100, .F. ) ;
#16221=ORIENTED_EDGE ( 'NONE', *, *, #3523, .F. ) ;
#16223=ORIENTED_EDGE ( 'NONE', *, *, #17523, .T. ) ;
#16224=CARTESIAN_POINT ( 'NONE',  ( 58.74999999999981526, -1.571497941946529142, 1.022750809560129648 ) ) ;
#16228=CARTESIAN_POINT ( 'NONE',  ( 58.66133336607577320, -1.875011749335998124, 0.03256983989574745858 ) ) ;
#16229=ADVANCED_FACE ( 'NONE', ( #26358 ), #5321, .T. ) ;
#16237=AXIS2_PLACEMENT_3D ( 'NONE', #5554, #30234, #30385 ) ;
#16238=DIRECTION ( 'NONE',  ( -0.000000000000000000, -0.000000000000000000, 1.000000000000000000 ) ) ;
#16240=CIRCLE ( 'NONE', #21824, 1.875000000000001776 ) ;
#16243=CARTESIAN_POINT ( 'NONE',  ( 58.66120520762600421, -0.4851925435080639004, -1.811135885493848408 ) ) ;
#16244=CARTESIAN_POINT ( 'NONE',  ( 58.65838214097809100, -0.9083679987361445995, 1.640356269755778751 ) ) ;
#16248=FACE_OUTER_BOUND ( 'NONE', #1663, .T. ) ;
#16258=EDGE_LOOP ( 'NONE', ( #24772, #13964, #12775, #9949 ) ) ;
#16261=ORIENTED_EDGE ( 'NONE', *, *, #2212, .F. ) ;
#16263=ORIENTED_EDGE ( 'NONE', *, *, #28388, .F. ) ;
#16264=CARTESIAN_POINT ( 'NONE',  ( 52.20711756518984004, -0.4999999999994533817, -1.807104036850122109 ) ) ;
#16266=ORIENTED_EDGE ( 'NONE', *, *, #18301, .F. ) ;
#16269=CARTESIAN_POINT ( 'NONE',  ( 52.13000000000001677, 0.5000000000005460077, -1.996089927833914146 ) ) ;
#16278=CARTESIAN_POINT ( 'NONE',  ( 61.09423418604053069, -0.6373668173463740150, -1.895722432252557432 ) ) ;
#16286=FACE_OUTER_BOUND ( 'NONE', #1640, .T. ) ;
#16291=CARTESIAN_POINT ( 'NONE',  ( 58.65838214097829706, 1.640356269756469310, 0.9083679987366242159 ) ) ;
#16314=CARTESIAN_POINT ( 'NONE',  ( 58.66107449606957402, -1.606832818401185747, -0.9668599424570839540 ) ) ;
#16319=CARTESIAN_POINT ( 'NONE',  ( 58.74999981196286569, -1.865248186429863564, -0.5877861523402161392 ) ) ;
#16323=CARTESIAN_POINT ( 'NONE',  ( 61.25000000000004263, -0.8718791990806975534, -1.626461527140063756 ) ) ;
#16328=DIRECTION ( 'NONE',  ( 1.000000000000000000, 1.018631342913014973E-14, 0.000000000000000000 ) ) ;
#16329=ORIENTED_EDGE ( 'NONE', *, *, #23521, .T. ) ;
#16330=EDGE_CURVE ( 'NONE', #21195, #24526, #4842, .T. ) ;
#16333=DIRECTION ( 'NONE',  ( 1.000000000000000000, 1.047444401652940007E-14, 0.000000000000000000 ) ) ;
#16335=DIRECTION ( 'NONE',  ( 1.000000000000000000, 1.047444401652940007E-14, 0.000000000000000000 ) ) ;
#16337=CARTESIAN_POINT ( 'NONE',  ( 58.64999999999999147, 1.872332544501737139, 0.09997921184905474157 ) ) ;
#16343=VERTEX_POINT ( 'NONE', #2456 ) ;
#16347=CIRCLE ( 'NONE', #23947, 0.1500000000000001887 ) ;
#16354=( NAMED_UNIT ( * ) PLANE_ANGLE_UNIT ( ) SI_UNIT ( $, .RADIAN. ) );
#16364=CARTESIAN_POINT ( 'NONE',  ( 58.75000000000002132, 6.153735859711025284E-13, 3.111507638930570854E-58 ) ) ;
#16371=ORIENTED_EDGE ( 'NONE', *, *, #4359, .F. ) ;
#16374=CARTESIAN_POINT ( 'NONE',  ( 58.72427158855736451, -1.600821037878293884, 0.9764256747731572261 ) ) ;
#16380=ADVANCED_FACE ( 'NONE', ( #2915 ), #223, .F. ) ;
#16383=ORIENTED_EDGE ( 'NONE', *, *, #27891, .T. ) ;
#16388=DIRECTION ( 'NONE',  ( 0.5633368246415177971, -0.8262273428075421755, 0.000000000000000000 ) ) ;
#16394=CARTESIAN_POINT ( 'NONE',  ( 58.75000000000002842, -0.8979909453704965072, 1.749377236608653297 ) ) ;
#16401=CARTESIAN_POINT ( 'NONE',  ( 51.14630318392405428, 0.9364487020640391846, 1.503522130792586342 ) ) ;
#16406=CARTESIAN_POINT ( 'NONE',  ( 58.75000000000002132, 6.153735859711025284E-13, 3.111507638930570854E-58 ) ) ;
#16407=ORIENTED_EDGE ( 'NONE', *, *, #771, .T. ) ;
#16408=CARTESIAN_POINT ( 'NONE',  ( 60.75000000000001421, 0.6500000000006362910, -1.489337100860648189 ) ) ;
#16419=CARTESIAN_POINT ( 'NONE',  ( 58.64999999999999147, 1.834410884276644449, -0.3880228184651526857 ) ) ;
#16423=CARTESIAN_POINT ( 'NONE',  ( 61.25000000000000711, 1.323060376182058961, -1.499837071477343242 ) ) ;
#16424=CARTESIAN_POINT ( 'NONE',  ( 52.20711756518984004, -0.4999999999994533817, -1.996089927833914146 ) ) ;
#16431=EDGE_LOOP ( 'NONE', ( #19872, #12533, #15386, #7866 ) ) ;
#16435=CARTESIAN_POINT ( 'NONE',  ( 58.75000000000002132, 6.153735859711025284E-13, 3.111507638930570854E-58 ) ) ;
#16439=VERTEX_POINT ( 'NONE', #8627 ) ;
#16440=ADVANCED_FACE ( 'NONE', ( #3258 ), #25260, .F. ) ;
#16441=CARTESIAN_POINT ( 'NONE',  ( 51.59739104186226655, 1.165722629542050415, 1.468576096419531352 ) ) ;
#16460=CARTESIAN_POINT ( 'NONE',  ( 58.65000000000001990, 6.143261415694495821E-13, 3.111507638930570854E-58 ) ) ;
#16462=CIRCLE ( 'NONE', #25034, 0.1499999999999999667 ) ;
#16465=PLANE ( 'NONE',  #13920 ) ;
#16467=CARTESIAN_POINT ( 'NONE',  ( 51.45655683570191741, -0.9591657938390835136, 1.468576096419531574 ) ) ;
#16469=B_SPLINE_CURVE_WITH_KNOTS ( 'NONE', 3,
 ( #31263, #6568, #21316, #16228, #25877, #1974 ),
 .UNSPECIFIED., .F., .F.,
 ( 4, 2, 4 ),
 ( 0.000000000000000000, 0.0001000270069600267081, 0.0002000540139200534162 ),
 .UNSPECIFIED. ) ;
#16473=CARTESIAN_POINT ( 'NONE',  ( 61.00000000000001421, 0.8666666666673054076, -1.374595900215364930 ) ) ;
#16476=ORIENTED_EDGE ( 'NONE', *, *, #62, .T. ) ;
#16483=AXIS2_PLACEMENT_3D ( 'NONE', #2996, #2686, #24518 ) ;
#16490=AXIS2_PLACEMENT_3D ( 'NONE', #23816, #60, #2436 ) ;
#16492=B_SPLINE_CURVE_WITH_KNOTS ( 'NONE', 3,
 ( #19428, #21819, #9764, #21351, #2316, #7383 ),
 .UNSPECIFIED., .F., .F.,
 ( 4, 2, 4 ),
 ( 0.000000000000000000, 0.0001000270069598671678, 0.0002000540139197343355 ),
 .UNSPECIFIED. ) ;
#16495=ORIENTED_EDGE ( 'NONE', *, *, #24105, .F. ) ;
#16503=CIRCLE ( 'NONE', #1818, 0.1500000000000001887 ) ;
#16508=DIRECTION ( 'NONE',  ( 1.000000000000000000, 1.047444401652940007E-14, -0.000000000000000000 ) ) ;
#16524=ORIENTED_EDGE ( 'NONE', *, *, #22731, .F. ) ;
#16526=DIRECTION ( 'NONE',  ( 1.000000000000000000, 1.047444401652940007E-14, 0.000000000000000000 ) ) ;
#16528=CIRCLE ( 'NONE', #27637, 1.875000000000001776 ) ;
#16538=ORIENTED_EDGE ( 'NONE', *, *, #12565, .T. ) ;
#16542=CYLINDRICAL_SURFACE ( 'NONE', #29817, 0.1500000000000001887 ) ;
#16552=VERTEX_POINT ( 'NONE', #19097 ) ;
#16555=CARTESIAN_POINT ( 'NONE',  ( 61.20026580823483187, 0.7453886133013672977, -1.660366360129213348 ) ) ;
#16559=DIRECTION ( 'NONE',  ( 1.000000000000000000, 1.047444401652940007E-14, 0.000000000000000000 ) ) ;
#16563=CARTESIAN_POINT ( 'NONE',  ( 58.65000000000004121, -1.782657835994308604, 0.5811678240972268927 ) ) ;
#16565=DIRECTION ( 'NONE',  ( 1.000000000000000000, 1.047444401652940007E-14, 0.000000000000000000 ) ) ;
#16566=CARTESIAN_POINT ( 'NONE',  ( 50.95599726996783829, 0.9532299437236954054, 1.316046228059489120 ) ) ;
#16574=EDGE_CURVE ( 'NONE', #15271, #28412, #4346, .T. ) ;
#16577=ORIENTED_EDGE ( 'NONE', *, *, #2933, .T. ) ;
#16583=ORIENTED_EDGE ( 'NONE', *, *, #25661, .F. ) ;
#16585=DIRECTION ( 'NONE',  ( 0.000000000000000000, -8.881784197001054122E-16, 1.000000000000000000 ) ) ;
#16586=VECTOR ( 'NONE', #22309, 1000.000000000000000 ) ;
#16591=ORIENTED_EDGE ( 'NONE', *, *, #15428, .F. ) ;
#16593=DIRECTION ( 'NONE',  ( 3.246618580117018983E-15, -0.3099561728520988102, -0.9507508458638782578 ) ) ;
#16607=CARTESIAN_POINT ( 'NONE',  ( 58.75000000000002132, -0.6373668173463985509, -1.895722432252557432 ) ) ;
#16610=ADVANCED_FACE ( 'NONE', ( #13997 ), #11305, .F. ) ;
#16613=CARTESIAN_POINT ( 'NONE',  ( 58.75000000000003553, -1.470078920827206925, -1.470078920827526892 ) ) ;
#16623=CARTESIAN_POINT ( 'NONE',  ( 58.65000000000001279, 0.8948927608039191073, -1.760622601996761460 ) ) ;
#16625=DIRECTION ( 'NONE',  ( 1.000000000000000000, 0.000000000000000000, -0.000000000000000000 ) ) ;
#16634=B_SPLINE_CURVE_WITH_KNOTS ( 'NONE', 3,
 ( #10127, #14571, #12489, #22016 ),
 .UNSPECIFIED., .F., .F.,
 ( 4, 4 ),
 ( 0.000000000000000000, 0.0003408895603972702908 ),
 .UNSPECIFIED. ) ;
#16641=ORIENTED_EDGE ( 'NONE', *, *, #20492, .T. ) ;
#16643=EDGE_CURVE ( 'NONE', #12544, #16052, #11485, .T. ) ;
#16650=EDGE_CURVE ( 'NONE', #30639, #17367, #8938, .T. ) ;
#16656=CARTESIAN_POINT ( 'NONE',  ( 58.66133336607637716, 0.9092995659220839411, -1.640092727267648876 ) ) ;
#16661=VERTEX_POINT ( 'NONE', #6576 ) ;
#16662=ORIENTED_EDGE ( 'NONE', *, *, #22032, .F. ) ;
#16663=CARTESIAN_POINT ( 'NONE',  ( 51.25834959657160539, -0.9980676081275761113, -1.403333189220955068 ) ) ;
#16669=CARTESIAN_POINT ( 'NONE',  ( 58.65844932252359456, 1.874781853997842251, 0.03312599131522728224 ) ) ;
#16677=AXIS2_PLACEMENT_3D ( 'NONE', #7456, #5219, #14867 ) ;
#16679=EDGE_CURVE ( 'NONE', #22168, #28767, #810, .T. ) ;
#16680=DIRECTION ( 'NONE',  ( -1.000000000000000000, -1.047444401652940007E-14, -0.000000000000000000 ) ) ;
#16694=DIRECTION ( 'NONE',  ( 1.000000000000000000, 1.047444401652940007E-14, 0.000000000000000000 ) ) ;
#16698=CIRCLE ( 'NONE', #3023, 0.1499999999999998557 ) ;
#16707=CIRCLE ( 'NONE', #3030, 0.09999999999999997780 ) ;
#16713=CARTESIAN_POINT ( 'NONE',  ( 61.25000000000004263, -1.895722432252919809, 0.6373668173470157239 ) ) ;
#16714=VERTEX_POINT ( 'NONE', #7664 ) ;
#16719=CARTESIAN_POINT ( 'NONE',  ( 58.74999999305997278, -0.9867593359911132067, -1.657788420845575983 ) ) ;
#16722=CARTESIAN_POINT ( 'NONE',  ( 58.65000000000001279, 0.5811678240991626776, -1.782657835994492457 ) ) ;
#16724=CARTESIAN_POINT ( 'NONE',  ( 58.65000076404083273, -0.5493821916573800035, -1.793020333199547123 ) ) ;
#16727=AXIS2_PLACEMENT_3D ( 'NONE', #7051, #30789, #14311 ) ;
#16728=CARTESIAN_POINT ( 'NONE',  ( 58.70142274306405028, -0.4999999999993853805, 1.816042500835558959 ) ) ;
#16731=DIRECTION ( 'NONE',  ( -1.000000000000000000, -1.018631342913014973E-14, -0.000000000000000000 ) ) ;
#16739=ORIENTED_EDGE ( 'NONE', *, *, #29024, .T. ) ;
#16746=EDGE_LOOP ( 'NONE', ( #1801, #14457, #12341, #14951 ) ) ;
#16770=CARTESIAN_POINT ( 'NONE',  ( 58.75000018595669360, 0.9248597378499668897, -1.701752411747084581 ) ) ;
#16771=CARTESIAN_POINT ( 'NONE',  ( 58.75000018803721247, -1.403930843796483696, 1.333992738917427978 ) ) ;
#16777=CARTESIAN_POINT ( 'NONE',  ( 58.66133336607565241, -1.302803168107663945, 1.348863877412472156 ) ) ;
#16778=EDGE_LOOP ( 'NONE', ( #7149, #20040, #26345, #6944 ) ) ;
#16786=CARTESIAN_POINT ( 'NONE',  ( 52.06628335902946247, -0.5434431642975682264, 1.794517909405659806 ) ) ;
#16796=ADVANCED_FACE ( 'NONE', ( #14479 ), #9742, .F. ) ;
#16797=CIRCLE ( 'NONE', #20838, 0.1499999999999999667 ) ;
#16803=CARTESIAN_POINT ( 'NONE',  ( 61.00000000000002842, -0.8666666666660278739, 1.374595900215364930 ) ) ;
#16806=CARTESIAN_POINT ( 'NONE',  ( 58.65838214097806258, -1.802220213625042700, 0.5175938701870494985 ) ) ;
#16816=ORIENTED_EDGE ( 'NONE', *, *, #11433, .F. ) ;
#16823=ORIENTED_EDGE ( 'NONE', *, *, #21609, .F. ) ;
#16827=EDGE_CURVE ( 'NONE', #25794, #1478, #29658, .T. ) ;
#16837=CIRCLE ( 'NONE', #9309, 2.000000000000000000 ) ;
#16839=CARTESIAN_POINT ( 'NONE',  ( 51.12687253673781385, -0.9194130538815391551, -1.491219977510798600 ) ) ;
#16847=DIRECTION ( 'NONE',  ( -1.000000000000000000, -1.018631342913014973E-14, -0.000000000000000000 ) ) ;
#16850=DIRECTION ( 'NONE',  ( 0.000000000000000000, 0.000000000000000000, 1.000000000000000000 ) ) ;
#16854=CARTESIAN_POINT ( 'NONE',  ( 60.88854248453741747, 0.6773709096947286845, -1.477839832418263999 ) ) ;
#16858=CARTESIAN_POINT ( 'NONE',  ( 61.25000000000004263, -1.666164585742961890, 1.106298139390331947 ) ) ;
#16868=CARTESIAN_POINT ( 'NONE',  ( 61.00000000000002132, 6.389410850082937196E-13, 3.111507638930570854E-58 ) ) ;
#16869=CARTESIAN_POINT ( 'NONE',  ( 58.66118217212513031, -0.9521303665436844366, -1.615348343402082110 ) ) ;
#16870=VERTEX_POINT ( 'NONE', #3837 ) ;
#16886=DIRECTION ( 'NONE',  ( 0.000000000000000000, 0.000000000000000000, 1.000000000000000000 ) ) ;
#16891=ORIENTED_EDGE ( 'NONE', *, *, #23699, .F. ) ;
#16916=ORIENTED_EDGE ( 'NONE', *, *, #26456, .F. ) ;
#16922=ORIENTED_EDGE ( 'NONE', *, *, #28236, .T. ) ;
#16923=DIRECTION ( 'NONE',  ( -0.000000000000000000, -0.000000000000000000, -1.000000000000000000 ) ) ;
#16924=CARTESIAN_POINT ( 'NONE',  ( 51.01608411450971658, 0.7569233679480920074, -1.030722644926826082 ) ) ;
#16926=CARTESIAN_POINT ( 'NONE',  ( 58.72200624034175576, 0.9185080301422264837, 1.634766674884828852 ) ) ;
#16939=TOROIDAL_SURFACE ( 'NONE', #2279, 1.975000000000001865, 0.1000000000000000056 ) ;
#16941=DIRECTION ( 'NONE',  ( 1.000000000000000000, 1.047444401652940007E-14, 0.000000000000000000 ) ) ;
#16944=AXIS2_PLACEMENT_3D ( 'NONE', #29104, #2352, #7419 ) ;
#16949=CARTESIAN_POINT ( 'NONE',  ( 58.64999999999999858, 1.278133834460348783, 1.372267738821557836 ) ) ;
#16951=CARTESIAN_POINT ( 'NONE',  ( 61.24179192282288398, -0.9092026280833716001, 1.724287941705032523 ) ) ;
#16954=ADVANCED_FACE ( 'NONE', ( #1013 ), #20655, .F. ) ;
#16961=ADVANCED_FACE ( 'NONE', ( #1763 ), #6843, .F. ) ;
#16965=CARTESIAN_POINT ( 'NONE',  ( 58.65000000000000568, 1.320082690054481755, -1.469015551796560182 ) ) ;
#16973=EDGE_CURVE ( 'NONE', #26116, #21148, #6882, .T. ) ;
#16988=CARTESIAN_POINT ( 'NONE',  ( 51.13341687362843402, -0.9248174436445972812, -1.495576127288424040 ) ) ;
#16993=AXIS2_PLACEMENT_3D ( 'NONE', #15761, #3143, #29739 ) ;
#16995=CARTESIAN_POINT ( 'NONE',  ( 51.24551381660811700, 1.093420264359095340, -1.202138525661323509 ) ) ;
#16997=EDGE_CURVE ( 'NONE', #704, #6604, #5350, .T. ) ;
#16999=ADVANCED_FACE ( 'NONE', ( #4151 ), #9231, .T. ) ;
#17004=EDGE_CURVE ( 'NONE', #624, #26230, #8892, .T. ) ;
#17031=EDGE_CURVE ( 'NONE', #8224, #11926, #4975, .T. ) ;
#17036=DIRECTION ( 'NONE',  ( 0.000000000000000000, 1.000000000000000000, 0.000000000000000000 ) ) ;
#17038=AXIS2_PLACEMENT_3D ( 'NONE', #26450, #2697, #19196 ) ;
#17039=CARTESIAN_POINT ( 'NONE',  ( 51.49777277048503521, 1.059151787769027298, 1.232523824083105346 ) ) ;
#17043=ORIENTED_EDGE ( 'NONE', *, *, #14412, .T. ) ;
#17049=AXIS2_PLACEMENT_3D ( 'NONE', #9848, #29008, #17437 ) ;
#17050=VECTOR ( 'NONE', #16559, 1000.000000000000000 ) ;
#17053=FACE_OUTER_BOUND ( 'NONE', #18864, .T. ) ;
#17060=ORIENTED_EDGE ( 'NONE', *, *, #18532, .F. ) ;
#17063=DIRECTION ( 'NONE',  ( -0.8023336663629152543, -0.5470456816110889076, -0.2387503090077617296 ) ) ;
#17065=AXIS2_PLACEMENT_3D ( 'NONE', #27955, #5254, #29629 ) ;
#17075=DIRECTION ( 'NONE',  ( 1.000000000000000000, 1.047444401652940007E-14, 0.000000000000000000 ) ) ;
#17079=CARTESIAN_POINT ( 'NONE',  ( 51.45655683570189609, 0.9591657938401617622, 1.196087371390568643 ) ) ;
#17080=AXIS2_PLACEMENT_3D ( 'NONE', #2355, #26745, #28806 ) ;
#17083=CARTESIAN_POINT ( 'NONE',  ( 50.25000000000000000, 1.470078920827345925, 1.470078920828533420 ) ) ;
#17089=DIRECTION ( 'NONE',  ( 0.000000000000000000, 1.000000000000000000, 0.000000000000000000 ) ) ;
#17090=DIRECTION ( 'NONE',  ( 0.000000000000000000, 0.000000000000000000, 1.000000000000000000 ) ) ;
#17109=CIRCLE ( 'NONE', #2454, 0.09999999999999997780 ) ;
#17110=EDGE_CURVE ( 'NONE', #10205, #12232, #803, .T. ) ;
#17112=CARTESIAN_POINT ( 'NONE',  ( 61.16862972101651508, 0.7079877303047974468, -1.871978752395131895 ) ) ;
#17117=CARTESIAN_POINT ( 'NONE',  ( 58.75000000000001421, 0.5380862305915415922, -2.008165151417984351 ) ) ;
#17118=DIRECTION ( 'NONE',  ( 0.000000000000000000, 0.5454670984329667016, -0.8381322357045577487 ) ) ;
#17121=CARTESIAN_POINT ( 'NONE',  ( 58.65000000000001279, 0.8495817349404606311, -1.671477153794393766 ) ) ;
#17122=ORIENTED_EDGE ( 'NONE', *, *, #935, .T. ) ;
#17123=CARTESIAN_POINT ( 'NONE',  ( 60.88048385701370080, 0.6732112958821407922, 1.479676701994273369 ) ) ;
#17129=DIRECTION ( 'NONE',  ( 0.000000000000000000, 0.000000000000000000, 1.000000000000000000 ) ) ;
#17131=( BOUNDED_CURVE ( )  B_SPLINE_CURVE ( 3, ( #3293, #29889, #18612, #22629 ),
 .UNSPECIFIED., .F., .T. ) 
 B_SPLINE_CURVE_WITH_KNOTS ( ( 4, 4 ),
 ( 4.050220903230332681, 4.465400561421049019 ),
 .UNSPECIFIED. ) 
 CURVE ( )  GEOMETRIC_REPRESENTATION_ITEM ( )  RATIONAL_B_SPLINE_CURVE ( ( 1.000000000000000000, 0.9856869983806462177, 0.9856869983806462177, 1.000000000000000000 ) ) 
 REPRESENTATION_ITEM ( '' )  );
#17133=CARTESIAN_POINT ( 'NONE',  ( 61.25000000000001421, 0.5000000000006414869, -1.807104036850122109 ) ) ;
#17137=ORIENTED_EDGE ( 'NONE', *, *, #25663, .F. ) ;
#17138=CARTESIAN_POINT ( 'NONE',  ( 58.65000038048067665, -1.383507098107042088, -1.265626441015408998 ) ) ;
#17150=CARTESIAN_POINT ( 'NONE',  ( 51.98855675296391610, 0.7791495708613139781, 1.432971607104406520 ) ) ;
#17156=CARTESIAN_POINT ( 'NONE',  ( 58.65000000000003411, -1.278133834460056795, -1.372267738820685423 ) ) ;
#17163=ORIENTED_EDGE ( 'NONE', *, *, #27008, .F. ) ;
#17170=ORIENTED_EDGE ( 'NONE', *, *, #27843, .T. ) ;
#17183=CARTESIAN_POINT ( 'NONE',  ( 58.75000018595671492, -1.011330950598887224, -1.651828233788867450 ) ) ;
#17188=CARTESIAN_POINT ( 'NONE',  ( 58.74154451056424620, -1.017012227664021662, 1.575232816092780652 ) ) ;
#17192=CARTESIAN_POINT ( 'NONE',  ( 61.25000000000003553, -0.9885922787754447549, -1.658880815145630239 ) ) ;
#17193=ORIENTED_EDGE ( 'NONE', *, *, #2038, .F. ) ;
#17194=CONICAL_SURFACE ( 'NONE', #4025, 1.875000000000001776, 0.7853981633974510546 ) ;
#17196=EDGE_LOOP ( 'NONE', ( #20743, #16641, #1332, #10602, #18559, #22272 ) ) ;
#17205=ORIENTED_EDGE ( 'NONE', *, *, #182, .F. ) ;
#17211=CARTESIAN_POINT ( 'NONE',  ( 51.23644008536124517, -1.080112125195908046, 1.214076932077873039 ) ) ;
#17219=DIRECTION ( 'NONE',  ( 0.5633368246415177971, -0.8262273428075421755, 0.000000000000000000 ) ) ;
#17222=DIRECTION ( 'NONE',  ( 1.000000000000000000, 1.047444401652940007E-14, -0.000000000000000000 ) ) ;
#17224=DIRECTION ( 'NONE',  ( 1.000000000000000000, 1.047444401652940007E-14, 0.000000000000000000 ) ) ;
#17225=CARTESIAN_POINT ( 'NONE',  ( 51.44193764627956256, -0.9752197701239264660, -1.304631266258929889 ) ) ;
#17231=CYLINDRICAL_SURFACE ( 'NONE', #1154, 0.2500000000000000000 ) ;
#17245=DIRECTION ( 'NONE',  ( 1.000000000000000000, 1.047444401652940007E-14, 0.000000000000000000 ) ) ;
#17248=DIRECTION ( 'NONE',  ( 2.468478480535042241E-12, -0.05332224631830475431, -0.9985773570673281974 ) ) ;
#17252=CARTESIAN_POINT ( 'NONE',  ( 58.65000000000001990, 6.143261415694495821E-13, 3.111507638930570854E-58 ) ) ;
#17256=CARTESIAN_POINT ( 'NONE',  ( 61.24919886530821600, -0.9685650917400145943, 1.667277206152059987 ) ) ;
#17260=CARTESIAN_POINT ( 'NONE',  ( 58.74999981196287280, -1.909245389981207408, 0.4235863532959572852 ) ) ;
#17262=DIRECTION ( 'NONE',  ( 1.000000000000000000, 1.047444401652940007E-14, 0.000000000000000000 ) ) ;
#17264=CARTESIAN_POINT ( 'NONE',  ( 58.69321565534372809, -0.4999999999993854916, -1.812725888577163103 ) ) ;
#17268=CARTESIAN_POINT ( 'NONE',  ( 51.98855675296393031, -0.7791495708602242942, -1.432971607104406297 ) ) ;
#17277=ORIENTED_EDGE ( 'NONE', *, *, #7380, .F. ) ;
#17279=CARTESIAN_POINT ( 'NONE',  ( 58.65266784251151222, -1.277991457600138991, -1.372094080476043310 ) ) ;
#17282=CIRCLE ( 'NONE', #17792, 0.2500000000000000000 ) ;
#17288=CARTESIAN_POINT ( 'NONE',  ( 58.66107449606936086, -1.819875603893454485, 0.4525291603558602715 ) ) ;
#17292=CARTESIAN_POINT ( 'NONE',  ( 58.65000000000001990, 6.143261415694495821E-13, 3.111507638930570854E-58 ) ) ;
#17299=DIRECTION ( 'NONE',  ( 1.000000000000000000, 1.047444401652940007E-14, 0.000000000000000000 ) ) ;
#17307=ADVANCED_FACE ( 'NONE', ( #20150 ), #16465, .F. ) ;
#17310=ORIENTED_EDGE ( 'NONE', *, *, #3638, .T. ) ;
#17311=CARTESIAN_POINT ( 'NONE',  ( 58.65817410504309493, -0.5270377936596636337, -1.799623063671780487 ) ) ;
#17313=CARTESIAN_POINT ( 'NONE',  ( 51.41939584733315627, 0.9814691331449714173, -1.432192464238639884 ) ) ;
#17315=ORIENTED_EDGE ( 'NONE', *, *, #9699, .F. ) ;
#17323=CARTESIAN_POINT ( 'NONE',  ( 58.75000000000003553, -0.8495817349395312634, -1.671477153794241888 ) ) ;
#17330=CARTESIAN_POINT ( 'NONE',  ( 58.66107449606985114, 1.874988011599642235, 0.03390886286986791870 ) ) ;
#17333=EDGE_LOOP ( 'NONE', ( #25986, #5740, #1316, #19147 ) ) ;
#17334=EDGE_CURVE ( 'NONE', #22781, #11615, #3342, .T. ) ;
#17335=VERTEX_POINT ( 'NONE', #6333 ) ;
#17343=ORIENTED_EDGE ( 'NONE', *, *, #7894, .F. ) ;
#17346=ORIENTED_EDGE ( 'NONE', *, *, #27872, .F. ) ;
#17362=ADVANCED_FACE ( 'NONE', ( #26121 ), #25649, .T. ) ;
#17363=ORIENTED_EDGE ( 'NONE', *, *, #10907, .T. ) ;
#17367=VERTEX_POINT ( 'NONE', #9347 ) ;
#17369=VERTEX_POINT ( 'NONE', #30392 ) ;
#17388=DIRECTION ( 'NONE',  ( 0.000000000000000000, 0.000000000000000000, 1.000000000000000000 ) ) ;
#17399=DIRECTION ( 'NONE',  ( 8.778969181338835100E-15, -0.8381322357048270888, -0.5454670984325526994 ) ) ;
#17403=CARTESIAN_POINT ( 'NONE',  ( 58.75000000000003553, -1.469015551795940233, -1.320082690053872465 ) ) ;
#17404=DIRECTION ( 'NONE',  ( 0.000000000000000000, 0.000000000000000000, 1.000000000000000000 ) ) ;
#17409=CARTESIAN_POINT ( 'NONE',  ( 61.00000000000001421, 0.8666666666673055186, 1.374595900215364930 ) ) ;
#17412=DIRECTION ( 'NONE',  ( 0.000000000000000000, 0.000000000000000000, 1.000000000000000000 ) ) ;
#17414=ORIENTED_EDGE ( 'NONE', *, *, #27046, .F. ) ;
#17418=CARTESIAN_POINT ( 'NONE',  ( 52.06628335902944826, 0.5434431642986600197, 1.718465885608439381 ) ) ;
#17437=DIRECTION ( 'NONE',  ( 0.000000000000000000, -0.9783524716136640098, -0.2069455031824436186 ) ) ;
#17440=( BOUNDED_SURFACE ( )  B_SPLINE_SURFACE ( 3, 2, ( 
 ( #882, #30149, #27317 ),
 ( #17507, #8008, #5630 ),
 ( #24782, #3091, #15280 ),
 ( #3247, #30784, #23350 ),
 ( #1633, #4330, #28084 ),
 ( #4173, #30453, #9097 ),
 ( #13669, #20975, #23676 ),
 ( #6874, #13812, #3870 ) ),
 .UNSPECIFIED., .F., .F., .T. ) 
 B_SPLINE_SURFACE_WITH_KNOTS ( ( 4, 2, 2, 4 ),
 ( 3, 3 ),
 ( 0.001762834131042899420, 0.001945267826973971163, 0.002127701522905042688, 0.002492568914767185739 ),
 ( 0.000000000000000000, 1.000000000000000000 ),
 .UNSPECIFIED. ) 
 GEOMETRIC_REPRESENTATION_ITEM ( )  RATIONAL_B_SPLINE_SURFACE ( (
 ( 1.000000000000000000, 0.8699658093904929501, 1.000000000000000000),
 ( 1.000000000000000000, 0.8851796357839230023, 1.000000000000000000),
 ( 1.000000000000000000, 0.8977447492167212051, 1.000000000000000000),
 ( 1.000000000000000000, 0.9127836411835494879, 1.000000000000000000),
 ( 1.000000000000000000, 0.9151168517135812586, 1.000000000000000000),
 ( 1.000000000000000000, 0.9045976586032165034, 1.000000000000000000),
 ( 1.000000000000000000, 0.8745315534097246601, 1.000000000000000000),
 ( 1.000000000000000000, 0.8388746406931713029, 1.000000000000000000) ) ) 
 REPRESENTATION_ITEM ( '' )  SURFACE ( )  );
#17442=FACE_OUTER_BOUND ( 'NONE', #19577, .T. ) ;
#17446=ORIENTED_EDGE ( 'NONE', *, *, #30368, .T. ) ;
#17456=ORIENTED_EDGE ( 'NONE', *, *, #27046, .T. ) ;
#17462=ORIENTED_EDGE ( 'NONE', *, *, #28147, .F. ) ;
#17465=EDGE_LOOP ( 'NONE', ( #22888, #8466, #3286, #22712 ) ) ;
#17467=ORIENTED_EDGE ( 'NONE', *, *, #6157, .F. ) ;
#17468=PRODUCT_DEFINITION ( 'UNKNOWN', '', #19727, #10442 ) ;
#17469=CARTESIAN_POINT ( 'NONE',  ( 58.75000000000002132, 6.153735859711025284E-13, 3.111507638930570854E-58 ) ) ;
#17472=ORIENTED_EDGE ( 'NONE', *, *, #25702, .F. ) ;
#17479=AXIS2_PLACEMENT_3D ( 'NONE', #26365, #14892, #5568 ) ;
#17484=CIRCLE ( 'NONE', #15464, 1.975000000000001865 ) ;
#17486=CYLINDRICAL_SURFACE ( 'NONE', #21510, 0.1499999999999999667 ) ;
#17490=CARTESIAN_POINT ( 'NONE',  ( 61.24312156765952864, -0.9166010152742726236, -1.712896921565310260 ) ) ;
#17496=ORIENTED_EDGE ( 'NONE', *, *, #21865, .T. ) ;
#17507=CARTESIAN_POINT ( 'NONE',  ( 51.55144386500324316, 1.037443573995146862, -1.251214392908886142 ) ) ;
#17519=CARTESIAN_POINT ( 'NONE',  ( 58.75000000000002132, -0.5380862305903304499, -1.858165151418244010 ) ) ;
#17520=CIRCLE ( 'NONE', #7902, 0.1500000000000001887 ) ;
#17521=CARTESIAN_POINT ( 'NONE',  ( 50.25000000000004263, -1.800471618824803111, 1.039502773796719959 ) ) ;
#17522=CARTESIAN_POINT ( 'NONE',  ( 51.23644008536121675, 1.080112125196981410, -1.214076932077873039 ) ) ;
#17523=EDGE_CURVE ( 'NONE', #11981, #28401, #14944, .T. ) ;
#17525=MECHANICAL_DESIGN_GEOMETRIC_PRESENTATION_REPRESENTATION('',(#7908),#15993);
#17527=FACE_OUTER_BOUND ( 'NONE', #16258, .T. ) ;
#17529=AXIS2_PLACEMENT_3D ( 'NONE', #16460, #13905, #30873 ) ;
#17531=CARTESIAN_POINT ( 'NONE',  ( 51.11922224407864945, -0.9310536428529800901, 1.338077479437885131 ) ) ;
#17536=ORIENTED_EDGE ( 'NONE', *, *, #27308, .F. ) ;
#17540=CARTESIAN_POINT ( 'NONE',  ( 51.45655683570191741, -0.9591657938390834026, 1.611094652690528095 ) ) ;
#17541=FACE_OUTER_BOUND ( 'NONE', #19538, .T. ) ;
#17550=DIRECTION ( 'NONE',  ( 1.000000000000000000, 1.047444401652940007E-14, -0.000000000000000000 ) ) ;
#17551=DIRECTION ( 'NONE',  ( 1.000000000000000000, 1.047444401652940007E-14, 0.000000000000000000 ) ) ;
#17559=TOROIDAL_SURFACE ( 'NONE', #30175, 1.975000000000001865, 0.1000000000000000056 ) ;
#17560=CIRCLE ( 'NONE', #21630, 0.8749999999999990008 ) ;
#17564=EDGE_CURVE ( 'NONE', #833, #17335, #14895, .T. ) ;
#17570=DIRECTION ( 'NONE',  ( 0.000000000000000000, 0.000000000000000000, 1.000000000000000000 ) ) ;
#17579=ORIENTED_EDGE ( 'NONE', *, *, #13333, .T. ) ;
#17585=ORIENTED_EDGE ( 'NONE', *, *, #1858, .F. ) ;
#17592=AXIS2_PLACEMENT_3D ( 'NONE', #1072, #1211, #30028 ) ;
#17596=CARTESIAN_POINT ( 'NONE',  ( 58.75000000000003553, -1.320082690053552499, -1.469015551796290175 ) ) ;
#17599=ORIENTED_EDGE ( 'NONE', *, *, #28131, .T. ) ;
#17603=B_SPLINE_CURVE_WITH_KNOTS ( 'NONE', 3,
 ( #13992, #31269, #2455, #9594 ),
 .UNSPECIFIED., .F., .F.,
 ( 4, 4 ),
 ( 1.084202172485504434E-19, 0.0001494103359351852626 ),
 .UNSPECIFIED. ) ;
#17612=DIRECTION ( 'NONE',  ( 1.000000000000000000, 1.047444401652940007E-14, 0.000000000000000000 ) ) ;
#17617=B_SPLINE_CURVE_WITH_KNOTS ( 'NONE', 3,
 ( #15608, #3573, #13521, #27790, #22892, #1337 ),
 .UNSPECIFIED., .F., .F.,
 ( 4, 2, 4 ),
 ( 0.000000000000000000, 0.0001917282624435965362, 0.0003834565248871930725 ),
 .UNSPECIFIED. ) ;
#17628=VERTEX_POINT ( 'NONE', #20537 ) ;
#17632=ADVANCED_FACE ( 'NONE', ( #5970 ), #10849, .F. ) ;
#17637=ADVANCED_FACE ( 'NONE', ( #1192 ), #8488, .F. ) ;
#17638=DIRECTION ( 'NONE',  ( 0.000000000000000000, 0.000000000000000000, 1.000000000000000000 ) ) ;
#17644=( BOUNDED_SURFACE ( )  B_SPLINE_SURFACE ( 3, 2, ( 
 ( #25521, #25377, #3679 ),
 ( #1300, #24899, #3386 ),
 ( #5919, #30428, #3834 ),
 ( #3220, #848, #10514 ) ),
 .UNSPECIFIED., .F., .F., .T. ) 
 B_SPLINE_SURFACE_WITH_KNOTS ( ( 4, 4 ),
 ( 3, 3 ),
 ( 0.0002753388251024970943, 0.0003797131536038330507 ),
 ( 0.000000000000000000, 1.000000000000000000 ),
 .UNSPECIFIED. ) 
 GEOMETRIC_REPRESENTATION_ITEM ( )  RATIONAL_B_SPLINE_SURFACE ( (
 ( 1.000000000000000000, 0.8543839308486376183, 1.000000000000000000),
 ( 1.000000000000000000, 0.8547349261770162965, 1.000000000000000000),
 ( 1.000000000000000000, 0.7665921203079560931, 1.000000000000000000),
 ( 1.000000000000000000, 0.7071067811865480168, 1.000000000000000000) ) ) 
 REPRESENTATION_ITEM ( '' )  SURFACE ( )  );
#17646=CYLINDRICAL_SURFACE ( 'NONE', #6163, 0.1500000000000003830 ) ;
#17647=DIRECTION ( 'NONE',  ( 1.000000000000000000, 1.047444401652940007E-14, 0.000000000000000000 ) ) ;
#17648=DIRECTION ( 'NONE',  ( 1.000000000000000000, 1.047444401652940007E-14, 0.000000000000000000 ) ) ;
#17652=FACE_OUTER_BOUND ( 'NONE', #7339, .T. ) ;
#17655=CARTESIAN_POINT ( 'NONE',  ( 58.66118217212537900, 1.313877211064007344, -1.337770226786318295 ) ) ;
#17667=ORIENTED_EDGE ( 'NONE', *, *, #10619, .T. ) ;
#17674=CARTESIAN_POINT ( 'NONE',  ( 58.75000000000000711, 1.895722432252915368, 0.6373668173479852816 ) ) ;
#17676=DIRECTION ( 'NONE',  ( 0.000000000000000000, 1.000000000000000000, 0.000000000000000000 ) ) ;
#17686=ADVANCED_FACE ( 'NONE', ( #18786 ), #9363, .F. ) ;
#17696=VERTEX_POINT ( 'NONE', #12119 ) ;
#17697=DIRECTION ( 'NONE',  ( 0.000000000000000000, 0.000000000000000000, 1.000000000000000000 ) ) ;
#17699=APPLICATION_CONTEXT ( 'automotive_design' ) ;
#17708=EDGE_CURVE ( 'NONE', #10186, #29981, #13868, .T. ) ;
#17714=CARTESIAN_POINT ( 'NONE',  ( 61.25000000000000000, 1.996089927834556965, -0.1249999999989956784 ) ) ;
#17718=CARTESIAN_POINT ( 'NONE',  ( 58.65844932252359456, 1.640171707773803167, -0.9087029769942892576 ) ) ;
#17729=EDGE_CURVE ( 'NONE', #11854, #30900, #21204, .T. ) ;
#17732=AXIS2_PLACEMENT_3D ( 'NONE', #2605, #27284, #10043 ) ;
#17734=ORIENTED_EDGE ( 'NONE', *, *, #19332, .T. ) ;
#17742=ORIENTED_EDGE ( 'NONE', *, *, #28982, .F. ) ;
#17749=ADVANCED_FACE ( 'NONE', ( #21473 ), #8971, .F. ) ;
#17765=CARTESIAN_POINT ( 'NONE',  ( 58.65000038048068376, -1.830965513784331034, -0.4043111005671602420 ) ) ;
#17768=CARTESIAN_POINT ( 'NONE',  ( 58.75000000000002132, 6.153735859711025284E-13, 3.111507638930570854E-58 ) ) ;
#17773=EDGE_CURVE ( 'NONE', #30639, #29589, #10054, .T. ) ;
#17777=CARTESIAN_POINT ( 'NONE',  ( 58.75000000000002132, 6.153735859711025284E-13, 3.111507638930570854E-58 ) ) ;
#17786=ADVANCED_FACE ( 'NONE', ( #17652 ), #17486, .F. ) ;
#17790=SHAPE_REPRESENTATION_RELATIONSHIP ( 'NONE' , 'NONE' ,  #9258, #27074 ) ;
#17792=AXIS2_PLACEMENT_3D ( 'NONE', #30429, #18418, #28055 ) ;
#17795=CARTESIAN_POINT ( 'NONE',  ( 50.59602332238209499, -0.1408342061598471806, -0.8215393206232035617 ) ) ;
#17796=ORIENTED_EDGE ( 'NONE', *, *, #24105, .T. ) ;
#17799=ORIENTED_EDGE ( 'NONE', *, *, #22179, .T. ) ;
#17806=B_SPLINE_CURVE_WITH_KNOTS ( 'NONE', 3,
 ( #7813, #26836, #27139, #24310 ),
 .UNSPECIFIED., .F., .F.,
 ( 4, 4 ),
 ( 0.000000000000000000, 0.0001493943817025111917 ),
 .UNSPECIFIED. ) ;
#17809=ADVANCED_FACE ( 'NONE', ( #3073 ), #12261, .F. ) ;
#17813=CARTESIAN_POINT ( 'NONE',  ( 58.72204580543383656, 1.309860786662855325, -1.341784641882255436 ) ) ;
#17815=ADVANCED_FACE ( 'NONE', ( #5610 ), #9745, .T. ) ;
#17837=CARTESIAN_POINT ( 'NONE',  ( 58.75000000000002132, 6.153735859711025284E-13, 3.111507638930570854E-58 ) ) ;
#17840=DIRECTION ( 'NONE',  ( 1.000000000000000000, 1.047444401652940007E-14, 0.000000000000000000 ) ) ;
#17844=ADVANCED_FACE ( 'NONE', ( #19407 ), #29049, .F. ) ;
#17846=CARTESIAN_POINT ( 'NONE',  ( 51.31757909864148104, -1.004435980685438157, 1.391945786376508343 ) ) ;
#17847=AXIS2_PLACEMENT_3D ( 'NONE', #28903, #233, #9895 ) ;
#17849=DIRECTION ( 'NONE',  ( 9.329605248950888974E-15, -1.000000000000000000, 0.000000000000000000 ) ) ;
#17852=DIRECTION ( 'NONE',  ( 2.471142467734912792E-12, -0.3099561728516428416, -0.9507508458640269167 ) ) ;
#17854=CARTESIAN_POINT ( 'NONE',  ( 51.78416995154975666, -0.8999235898776962728, 1.360374659026170496 ) ) ;
#17856=CARTESIAN_POINT ( 'NONE',  ( 61.25000000000003553, -0.8813478542982779995, 1.623476567772350387 ) ) ;
#17860=EDGE_CURVE ( 'NONE', #12058, #27852, #4988, .T. ) ;
#17866=EDGE_LOOP ( 'NONE', ( #30871, #30144, #28069, #3456 ) ) ;
#17871=DIRECTION ( 'NONE',  ( -1.000000000000000000, -1.047444401652940007E-14, -0.000000000000000000 ) ) ;
#17879=ADVANCED_FACE ( 'NONE', ( #21946 ), #16939, .F. ) ;
#17885=VERTEX_POINT ( 'NONE', #14789 ) ;
#17886=CARTESIAN_POINT ( 'NONE',  ( 52.06628335902946247, -0.5434431642975682264, 1.794517909405659806 ) ) ;
#17893=FACE_OUTER_BOUND ( 'NONE', #29927, .T. ) ;
#17902=VERTEX_POINT ( 'NONE', #22552 ) ;
#17924=CARTESIAN_POINT ( 'NONE',  ( 58.75000000000002842, -0.8948927608041769011, 1.760622601996005177 ) ) ;
#17934=CARTESIAN_POINT ( 'NONE',  ( 58.65000000000000568, 1.656314228059722282, -0.8794134543718038488 ) ) ;
#17938=VERTEX_POINT ( 'NONE', #15874 ) ;
#17941=ADVANCED_FACE ( 'NONE', ( #13323 ), #20660, .F. ) ;
#17951=DIRECTION ( 'NONE',  ( 1.000000000000000000, 1.047444401652940007E-14, 0.000000000000000000 ) ) ;
#17958=CARTESIAN_POINT ( 'NONE',  ( 58.74999981196283727, 1.441661833136088866, -1.321459237640081330 ) ) ;
#17961=ORIENTED_EDGE ( 'NONE', *, *, #14412, .F. ) ;
#17970=EDGE_LOOP ( 'NONE', ( #2707, #30844, #9211, #12934 ) ) ;
#17972=DIRECTION ( 'NONE',  ( 0.000000000000000000, 0.9507508458636236837, 0.3099561728528797966 ) ) ;
#17976=ORIENTED_EDGE ( 'NONE', *, *, #20650, .T. ) ;
#17998=CARTESIAN_POINT ( 'NONE',  ( 51.45655683570191741, -0.9591657938390837357, 1.468576096419531574 ) ) ;
#18000=CARTESIAN_POINT ( 'NONE',  ( 50.25000000000002842, -0.8897917884445627479, 1.791164585743103999 ) ) ;
#18004=DIRECTION ( 'NONE',  ( 0.000000000000000000, 0.000000000000000000, 1.000000000000000000 ) ) ;
#18005=ORIENTED_EDGE ( 'NONE', *, *, #24815, .T. ) ;
#18006=VECTOR ( 'NONE', #756, 1000.000000000000000 ) ;
#18007=( BOUNDED_SURFACE ( )  B_SPLINE_SURFACE ( 3, 2, ( 
 ( #1472, #23480, #4008 ),
 ( #18900, #21294, #1952 ),
 ( #15737, #20664, #26003 ),
 ( #6231, #4312, #3690 ),
 ( #9241, #13796, #8601 ),
 ( #1773, #20807, #6085 ),
 ( #13961, #16207, #28392 ),
 ( #8903, #3849, #28238 ),
 ( #13498, #23334, #23660 ),
 ( #11448, #25855, #18428 ) ),
 .UNSPECIFIED., .F., .F., .F. ) 
 B_SPLINE_SURFACE_WITH_KNOTS ( ( 4, 2, 2, 2, 4 ),
 ( 3, 3 ),
 ( 0.0001706658715699256265, 0.0002229276920781272985, 0.0002751895125863289705, 0.0003274513330945306154, 0.0003797131536027322602 ),
 ( 0.000000000000000000, 1.000000000000000000 ),
 .UNSPECIFIED. ) 
 GEOMETRIC_REPRESENTATION_ITEM ( )  RATIONAL_B_SPLINE_SURFACE ( (
 ( 1.000000000000000000, 0.7071067811873685827, 1.000000000000000000),
 ( 1.000000000000000000, 0.7375607040707305995, 1.000000000000000000),
 ( 1.000000000000000000, 0.7730431127433396998, 1.000000000000000000),
 ( 1.000000000000000000, 0.8321012486978203171, 1.000000000000000000),
 ( 1.000000000000000000, 0.8541932017396182131, 1.000000000000000000),
 ( 1.000000000000000000, 0.8545723906043213303, 1.000000000000000000),
 ( 1.000000000000000000, 0.8327032135035172811, 1.000000000000000000),
 ( 1.000000000000000000, 0.7734559727056840028, 1.000000000000000000),
 ( 1.000000000000000000, 0.7377766653993875767, 1.000000000000000000),
 ( 1.000000000000000000, 0.7071067811865514585, 1.000000000000000000) ) ) 
 REPRESENTATION_ITEM ( '' )  SURFACE ( )  );
#18010=CARTESIAN_POINT ( 'NONE',  ( 61.22030551133047993, -0.7785732690188782446, 1.430137637026189790 ) ) ;
#18024=CARTESIAN_POINT ( 'NONE',  ( 58.75000000000000711, 1.749295403806236049, -0.8980135333475087744 ) ) ;
#18025=ADVANCED_FACE ( 'NONE', ( #10810 ), #15733, .F. ) ;
#18035=CIRCLE ( 'NONE', #19056, 0.1500000000000001887 ) ;
#18039=B_SPLINE_CURVE_WITH_KNOTS ( 'NONE', 3,
 ( #22615, #2804, #7573, #5503, #15156, #24494 ),
 .UNSPECIFIED., .F., .F.,
 ( 4, 2, 4 ),
 ( 0.000000000000000000, 0.0001000270069603039115, 0.0002000540139206078230 ),
 .UNSPECIFIED. ) ;
#18043=VECTOR ( 'NONE', #18551, 1000.000000000000000 ) ;
#18045=VECTOR ( 'NONE', #22063, 1000.000000000000000 ) ;
#18053=DIRECTION ( 'NONE',  ( 0.000000000000000000, 0.000000000000000000, 1.000000000000000000 ) ) ;
#18054=CARTESIAN_POINT ( 'NONE',  ( 61.25000000000000711, 1.470078920828170821, -1.470078920826818125 ) ) ;
#18055=DIRECTION ( 'NONE',  ( 1.000000000000000000, 1.047444401652940007E-14, -0.000000000000000000 ) ) ;
#18070=B_SPLINE_CURVE_WITH_KNOTS ( 'NONE', 3,
 ( #8859, #4596, #20921, #30551, #11240, #16803 ),
 .UNSPECIFIED., .F., .F.,
 ( 4, 2, 4 ),
 ( 0.000000000000000000, 0.0001966045864160470319, 0.0003932091728320940638 ),
 .UNSPECIFIED. ) ;
#18074=ORIENTED_EDGE ( 'NONE', *, *, #17773, .F. ) ;
#18077=CARTESIAN_POINT ( 'NONE',  ( 51.14630318392405428, 0.9364487020640391846, 1.503522130792586342 ) ) ;
#18082=VECTOR ( 'NONE', #22681, 1000.000000000000000 ) ;
#18083=CARTESIAN_POINT ( 'NONE',  ( 51.64837794009019234, 0.8283786772117797126, 1.688958810662478660 ) ) ;
#18091=CARTESIAN_POINT ( 'NONE',  ( 58.75000000000002842, -1.039502773796971091, 1.800471618824829756 ) ) ;
#18095=DIRECTION ( 'NONE',  ( 1.000000000000000000, 1.047444401652940007E-14, 0.000000000000000000 ) ) ;
#18100=AXIS2_PLACEMENT_3D ( 'NONE', #4716, #5044, #19461 ) ;
#18108=( LENGTH_UNIT ( ) NAMED_UNIT ( * ) SI_UNIT ( .MILLI., .METRE. ) );
#18111=EDGE_CURVE ( 'NONE', #29960, #8275, #2299, .T. ) ;
#18130=DIRECTION ( 'NONE',  ( -0.8023336663629263565, 0.5470456816110726983, 0.2387503090077608969 ) ) ;
#18136=ADVANCED_FACE ( 'NONE', ( #28863 ), #18585, .T. ) ;
#18137=CARTESIAN_POINT ( 'NONE',  ( 51.25000000000001421, 5.368152558471320595E-13, 3.111507638930570854E-58 ) ) ;
#18139=ORIENTED_EDGE ( 'NONE', *, *, #26822, .T. ) ;
#18141=CARTESIAN_POINT ( 'NONE',  ( 61.25000000000001421, 0.8666666666673039643, -1.374595900215358268 ) ) ;
#18156=CARTESIAN_POINT ( 'NONE',  ( 52.06628335902944826, 0.5434431642986583544, -1.996089927833914146 ) ) ;
#18163=CARTESIAN_POINT ( 'NONE',  ( 58.74999981196283727, 1.321459237640902007, 1.441661833135547965 ) ) ;
#18166=CARTESIAN_POINT ( 'NONE',  ( 50.25000000000002842, -0.6373668173464875908, -1.895722432252557432 ) ) ;
#18168=DIRECTION ( 'NONE',  ( 1.000000000000000000, 1.047444401652940007E-14, 0.000000000000000000 ) ) ;
#18169=CARTESIAN_POINT ( 'NONE',  ( 50.25000000000000000, 1.791164585742626159, 0.8897917884450912140 ) ) ;
#18171=CARTESIAN_POINT ( 'NONE',  ( 58.75000000000002132, 6.153735859711025284E-13, 3.111507638930570854E-58 ) ) ;
#18179=DIRECTION ( 'NONE',  ( 1.000000000000000000, 1.047444401652940007E-14, 0.000000000000000000 ) ) ;
#18183=DIRECTION ( 'NONE',  ( -1.000000000000000000, -1.047444401652940007E-14, -0.000000000000000000 ) ) ;
#18197=DIRECTION ( 'NONE',  ( 1.000000000000000000, 1.047444401652940007E-14, 0.000000000000000000 ) ) ;
#18199=ORIENTED_EDGE ( 'NONE', *, *, #31253, .T. ) ;
#18212=CIRCLE ( 'NONE', #25265, 1.975000000000001865 ) ;
#18217=CARTESIAN_POINT ( 'NONE',  ( 58.65000000000000568, 0.8495817349404608532, -1.671477153794393766 ) ) ;
#18223=CARTESIAN_POINT ( 'NONE',  ( 50.25000000000001421, 0.6373668173465375508, 1.895722432253563516 ) ) ;
#18229=EDGE_CURVE ( 'NONE', #20284, #26116, #26548, .T. ) ;
#18234=CARTESIAN_POINT ( 'NONE',  ( 51.15394434968253279, 0.9591183795348902086, -1.387856512383046637 ) ) ;
#18238=LINE ( 'NONE', #8097, #18082 ) ;
#18239=DIRECTION ( 'NONE',  ( 0.000000000000000000, 0.000000000000000000, 1.000000000000000000 ) ) ;
#18242=DIRECTION ( 'NONE',  ( 1.000000000000000000, 1.047444401652940007E-14, 0.000000000000000000 ) ) ;
#18243=ADVANCED_FACE ( 'NONE', ( #27875 ), #3183, .F. ) ;
#18245=DIRECTION ( 'NONE',  ( -1.000000000000000000, -1.047444401652940007E-14, -0.000000000000000000 ) ) ;
#18249=DIRECTION ( 'NONE',  ( 1.000000000000000000, 1.047444401652940007E-14, 0.000000000000000000 ) ) ;
#18251=DIRECTION ( 'NONE',  ( -1.000000000000000000, -1.047444401652940007E-14, -0.000000000000000000 ) ) ;
#18256=CARTESIAN_POINT ( 'NONE',  ( 61.25000000000002132, 6.415596960124259844E-13, 3.111507638930570854E-58 ) ) ;
#18268=DIRECTION ( 'NONE',  ( 0.000000000000000000, 0.000000000000000000, 1.000000000000000000 ) ) ;
#18276=DIRECTION ( 'NONE',  ( 1.000000000000000000, 1.018631342913014973E-14, 0.000000000000000000 ) ) ;
#18284=ORIENTED_EDGE ( 'NONE', *, *, #18537, .T. ) ;
#18293=CARTESIAN_POINT ( 'NONE',  ( 58.74999999305997989, -1.657788420846199706, 0.9867593359912983919 ) ) ;
#18298=DIRECTION ( 'NONE',  ( 1.000000000000000000, 1.047444401652940007E-14, 0.000000000000000000 ) ) ;
#18301=EDGE_CURVE ( 'NONE', #21983, #29950, #15697, .T. ) ;
#18304=AXIS2_PLACEMENT_3D ( 'NONE', #6686, #6221, #30758 ) ;
#18305=CARTESIAN_POINT ( 'NONE',  ( 51.23644008536122385, 1.080112125196981854, 1.214076932077872817 ) ) ;
#18307=DIRECTION ( 'NONE',  ( 0.000000000000000000, 0.8914544820235111855, -0.4531102586349080030 ) ) ;
#18311=LINE ( 'NONE', #18169, #8952 ) ;
#18313=EDGE_CURVE ( 'NONE', #4452, #22781, #27552, .T. ) ;
#18317=ADVANCED_FACE ( 'NONE', ( #20153 ), #9807, .F. ) ;
#18318=DIRECTION ( 'NONE',  ( 2.459994892347944311E-12, 0.6683962987616191009, -0.7438053426816511049 ) ) ;
#18319=ORIENTED_EDGE ( 'NONE', *, *, #9215, .F. ) ;
#18323=ORIENTED_EDGE ( 'NONE', *, *, #6312, .F. ) ;
#18326=CARTESIAN_POINT ( 'NONE',  ( 50.50000000000001421, 0.7375000000005331735, 3.111507638930570854E-58 ) ) ;
#18328=ORIENTED_EDGE ( 'NONE', *, *, #4402, .T. ) ;
#18338=B_SPLINE_CURVE_WITH_KNOTS ( 'NONE', 3,
 ( #2164, #28924, #18814, #28458 ),
 .UNSPECIFIED., .F., .F.,
 ( 4, 4 ),
 ( 8.741117365843378158E-19, 2.862003379457683788E-05 ),
 .UNSPECIFIED. ) ;
#18340=CARTESIAN_POINT ( 'NONE',  ( 58.66118217212532215, 1.806736155628216656, -0.5016043952913777915 ) ) ;
#18352=CARTESIAN_POINT ( 'NONE',  ( 58.65844932252321797, -1.874781853996629666, -0.03312599131424567855 ) ) ;
#18355=CARTESIAN_POINT ( 'NONE',  ( 58.65000038048027164, 1.663933463836820170, 0.8644232797869607632 ) ) ;
#18364=DIRECTION ( 'NONE',  ( 1.000000000000000000, 1.047444401652940007E-14, 0.000000000000000000 ) ) ;
#18366=ORIENTED_EDGE ( 'NONE', *, *, #25559, .F. ) ;
#18369=FACE_OUTER_BOUND ( 'NONE', #14953, .T. ) ;
#18372=B_SPLINE_CURVE_WITH_KNOTS ( 'NONE', 3,
 ( #6496, #6331, #18698, #8693, #23764, #8847, #31022, #13600, #23289, #1574, #18540, #16154, #4112 ),
 .UNSPECIFIED., .F., .F.,
 ( 4, 3, 3, 3, 4 ),
 ( 0.000000000000000000, 4.969793434218336409E-05, 9.932084631986548421E-05, 0.0001499488332825157780, 0.0001857305951757664718 ),
 .UNSPECIFIED. ) ;
#18383=FACE_OUTER_BOUND ( 'NONE', #26710, .T. ) ;
#18387=DIRECTION ( 'NONE',  ( 1.000000000000000000, 1.047444401652940007E-14, 0.000000000000000000 ) ) ;
#18393=CARTESIAN_POINT ( 'NONE',  ( 58.72200624034154259, 1.805437858156837549, 0.5064713447814576108 ) ) ;
#18403=CARTESIAN_POINT ( 'NONE',  ( 51.25000000000001421, 5.368159983410797313E-13, 3.111507638930570854E-58 ) ) ;
#18404=ORIENTED_EDGE ( 'NONE', *, *, #12165, .T. ) ;
#18409=DIRECTION ( 'NONE',  ( -1.000000000000000000, -1.047444401652940007E-14, -0.000000000000000000 ) ) ;
#18411=CIRCLE ( 'NONE', #8776, 0.1500000000000001887 ) ;
#18416=ADVANCED_FACE ( 'NONE', ( #18383 ), #6844, .F. ) ;
#18418=DIRECTION ( 'NONE',  ( 1.000000000000000000, 1.047444401652940007E-14, 0.000000000000000000 ) ) ;
#18420=VECTOR ( 'NONE', #26253, 1000.000000000000000 ) ;
#18428=CARTESIAN_POINT ( 'NONE',  ( 58.65000000000003411, -1.571497941946114585, -1.022750809560766250 ) ) ;
#18437=CARTESIAN_POINT ( 'NONE',  ( 51.31572262954152563, 1.002608958138273554, 1.584424273060082378 ) ) ;
#18438=AXIS2_PLACEMENT_3D ( 'NONE', #21543, #31185, #19177 ) ;
#18439=DIRECTION ( 'NONE',  ( 0.000000000000000000, 0.000000000000000000, 1.000000000000000000 ) ) ;
#18446=CARTESIAN_POINT ( 'NONE',  ( 61.09423418603945777, 0.6373668173466511266, 1.895722432253563516 ) ) ;
#18467=DIRECTION ( 'NONE',  ( 0.000000000000000000, 0.000000000000000000, 1.000000000000000000 ) ) ;
#18470=ADVANCED_FACE ( 'NONE', ( #2832 ), #15023, .F. ) ;
#18471=DIRECTION ( 'NONE',  ( 1.000000000000000000, 1.047444401652940007E-14, 0.000000000000000000 ) ) ;
#18472=( BOUNDED_SURFACE ( )  B_SPLINE_SURFACE ( 3, 2, ( 
 ( #14562, #24227, #10230 ),
 ( #29527, #20991, #3579 ),
 ( #9111, #13685, #8483 ),
 ( #23366, #20696, #30164 ),
 ( #13532, #6114, #28267 ),
 ( #8770, #3717, #30320 ),
 ( #15619, #18780, #27801 ),
 ( #18163, #5965, #15764 ),
 ( #8628, #11306, #11486 ),
 ( #18626, #3882, #30467 ) ),
 .UNSPECIFIED., .F., .F., .T. ) 
 B_SPLINE_SURFACE_WITH_KNOTS ( ( 4, 2, 2, 2, 4 ),
 ( 3, 3 ),
 ( 0.0001706658715694011708, 0.0002229276920777971318, 0.0002751895125861931199, 0.0003274513330945891081, 0.0003797131536029850962 ),
 ( 0.000000000000000000, 1.000000000000000000 ),
 .UNSPECIFIED. ) 
 GEOMETRIC_REPRESENTATION_ITEM ( )  RATIONAL_B_SPLINE_SURFACE ( (
 ( 1.000000000000000000, 0.7071067811865441310, 1.000000000000000000),
 ( 1.000000000000000000, 0.7375607040700675743, 1.000000000000000000),
 ( 1.000000000000000000, 0.7730431127425798632, 1.000000000000000000),
 ( 1.000000000000000000, 0.8321012486979311173, 1.000000000000000000),
 ( 1.000000000000000000, 0.8541932017400215571, 1.000000000000000000),
 ( 1.000000000000000000, 0.8545723906050046725, 1.000000000000000000),
 ( 1.000000000000000000, 0.8327032135041435579, 1.000000000000000000),
 ( 1.000000000000000000, 0.7734559727060076328, 1.000000000000000000),
 ( 1.000000000000000000, 0.7377766653995073698, 1.000000000000000000),
 ( 1.000000000000000000, 0.7071067811865465735, 1.000000000000000000) ) ) 
 REPRESENTATION_ITEM ( '' )  SURFACE ( )  );
#18476=CARTESIAN_POINT ( 'NONE',  ( 58.75000000000002132, 6.153735859711025284E-13, 3.111507638930570854E-58 ) ) ;
#18479=CIRCLE ( 'NONE', #11892, 1.875000000000001776 ) ;
#18481=FACE_OUTER_BOUND ( 'NONE', #30412, .T. ) ;
#18490=CIRCLE ( 'NONE', #23048, 0.09999999999999989453 ) ;
#18492=FACE_OUTER_BOUND ( 'NONE', #24453, .T. ) ;
#18493=CARTESIAN_POINT ( 'NONE',  ( 51.14630318392407560, -0.9364487020629673752, -1.503522130792586564 ) ) ;
#18500=CARTESIAN_POINT ( 'NONE',  ( 61.05467743520237178, -0.5998170657512601478, -1.862568116882888480 ) ) ;
#18501=AXIS2_PLACEMENT_3D ( 'NONE', #19904, #18168, #27810 ) ;
#18509=DIRECTION ( 'NONE',  ( 0.7071067811865455743, 7.319954787623226069E-15, -0.7071067811865493491 ) ) ;
#18511=CARTESIAN_POINT ( 'NONE',  ( 58.66122797211851747, 1.615588400947291392, 0.9517229765820476306 ) ) ;
#18513=DIRECTION ( 'NONE',  ( 0.000000000000000000, 0.000000000000000000, 1.000000000000000000 ) ) ;
#18515=DIRECTION ( 'NONE',  ( 1.000000000000000000, 1.047444401652940007E-14, 0.000000000000000000 ) ) ;
#18519=ORIENTED_EDGE ( 'NONE', *, *, #10405, .T. ) ;
#18525=VERTEX_POINT ( 'NONE', #22174 ) ;
#18532=EDGE_CURVE ( 'NONE', #15307, #22261, #23057, .T. ) ;
#18534=CARTESIAN_POINT ( 'NONE',  ( 51.84772254680353143, 0.6924618999072380543, -1.653428777428159968 ) ) ;
#18536=CARTESIAN_POINT ( 'NONE',  ( 51.24099374247646921, -1.086790822298242087, 1.208135181987622486 ) ) ;
#18537=EDGE_CURVE ( 'NONE', #14302, #15552, #8372, .T. ) ;
#18538=ORIENTED_EDGE ( 'NONE', *, *, #21037, .T. ) ;
#18540=CARTESIAN_POINT ( 'NONE',  ( 61.23837541685294639, 0.8927489269151840379, -1.767200183692393844 ) ) ;
#18547=AXIS2_PLACEMENT_3D ( 'NONE', #3348, #12679, #19686 ) ;
#18551=DIRECTION ( 'NONE',  ( 1.000000000000000000, 1.047444401652940007E-14, 0.000000000000000000 ) ) ;
#18555=CARTESIAN_POINT ( 'NONE',  ( 58.64999999999999147, 1.782657835994909901, 0.5811678240991509092 ) ) ;
#18559=ORIENTED_EDGE ( 'NONE', *, *, #21654, .F. ) ;
#18561=DIRECTION ( 'NONE',  ( -0.000000000000000000, -0.000000000000000000, -1.000000000000000000 ) ) ;
#18562=ORIENTED_EDGE ( 'NONE', *, *, #17334, .T. ) ;
#18563=EDGE_CURVE ( 'NONE', #21195, #24661, #14943, .T. ) ;
#18564=DIRECTION ( 'NONE',  ( 0.000000000000000000, 0.000000000000000000, 1.000000000000000000 ) ) ;
#18567=CARTESIAN_POINT ( 'NONE',  ( 58.65000045311409593, 1.873226731664826117, 0.08323357347720464205 ) ) ;
#18569=AXIS2_PLACEMENT_3D ( 'NONE', #9323, #14367, #26562 ) ;
#18575=ORIENTED_EDGE ( 'NONE', *, *, #3647, .F. ) ;
#18585=PLANE ( 'NONE',  #13394 ) ;
#18595=CARTESIAN_POINT ( 'NONE',  ( 50.59602332238209499, -0.1408342061598474859, 1.212874140286674285 ) ) ;
#18608=VERTEX_POINT ( 'NONE', #22801 ) ;
#18611=CARTESIAN_POINT ( 'NONE',  ( 58.65000000000003411, -1.571497941946663923, 1.022750809559922036 ) ) ;
#18612=CARTESIAN_POINT ( 'NONE',  ( 50.93312545610844211, -0.6352506689584648258, 1.438808137080897165 ) ) ;
#18613=ORIENTED_EDGE ( 'NONE', *, *, #25043, .F. ) ;
#18618=ORIENTED_EDGE ( 'NONE', *, *, #30350, .F. ) ;
#18626=CARTESIAN_POINT ( 'NONE',  ( 58.75000000000000711, 1.320082690053780983, 1.469015551797190788 ) ) ;
#18628=CARTESIAN_POINT ( 'NONE',  ( 58.75000000000003553, -1.499837071478441031, 1.323060376181713016 ) ) ;
#18630=DIRECTION ( 'NONE',  ( 0.000000000000000000, 0.000000000000000000, -1.000000000000000000 ) ) ;
#18633=CARTESIAN_POINT ( 'NONE',  ( 61.23793632918122398, -0.8908246368665424519, -1.774550402278997518 ) ) ;
#18643=ORIENTED_EDGE ( 'NONE', *, *, #12677, .T. ) ;
#18645=DIRECTION ( 'NONE',  ( 1.000000000000000000, 1.047444401652940007E-14, 0.000000000000000000 ) ) ;
#18649=DIRECTION ( 'NONE',  ( 0.000000000000000000, -1.000000000000000000, 0.000000000000000000 ) ) ;
#18654=CARTESIAN_POINT ( 'NONE',  ( 51.25000000000002842, -1.099999999999462963, -1.996089927833914146 ) ) ;
#18660=CARTESIAN_POINT ( 'NONE',  ( 58.75000000000002132, 6.153735859711025284E-13, 3.111507638930570854E-58 ) ) ;
#18667=CARTESIAN_POINT ( 'NONE',  ( 51.23644008536122385, 1.080112125196981854, 1.214076932077872817 ) ) ;
#18674=FACE_OUTER_BOUND ( 'NONE', #24548, .T. ) ;
#18676=CARTESIAN_POINT ( 'NONE',  ( 58.65844932252308297, -1.349094575298446008, 1.302247349114806552 ) ) ;
#18677=ORIENTED_EDGE ( 'NONE', *, *, #3852, .F. ) ;
#18690=CARTESIAN_POINT ( 'NONE',  ( 50.59602332238209499, 0.1408342061609074158, -1.212874140286673841 ) ) ;
#18696=( BOUNDED_SURFACE ( )  B_SPLINE_SURFACE ( 3, 2, ( 
 ( #9983, #9818, #2551 ),
 ( #7144, #14254, #11731 ),
 ( #24383, #2693, #21878 ),
 ( #12332, #310, #16806 ),
 ( #21562, #9533, #7451 ),
 ( #28833, #4912, #29292 ),
 ( #165, #19, #7604 ),
 ( #17260, #26903, #5214 ),
 ( #2067, #6993, #21728 ),
 ( #12199, #9357, #14403 ) ),
 .UNSPECIFIED., .F., .F., .F. ) 
 B_SPLINE_SURFACE_WITH_KNOTS ( ( 4, 2, 2, 2, 4 ),
 ( 3, 3 ),
 ( 0.0001706658715701054685, 0.0002229276920781130141, 0.0002751895125861205868, 0.0003274513330941281053, 0.0003797131536021356780 ),
 ( 0.000000000000000000, 1.000000000000000000 ),
 .UNSPECIFIED. ) 
 GEOMETRIC_REPRESENTATION_ITEM ( )  RATIONAL_B_SPLINE_SURFACE ( (
 ( 1.000000000000000000, 0.7071067811873459341, 1.000000000000000000),
 ( 1.000000000000000000, 0.7375607040706478879, 1.000000000000000000),
 ( 1.000000000000000000, 0.7730431127430092975, 1.000000000000000000),
 ( 1.000000000000000000, 0.8321012486969630029, 1.000000000000000000),
 ( 1.000000000000000000, 0.8541932017383955245, 1.000000000000000000),
 ( 1.000000000000000000, 0.8545723906030464612, 1.000000000000000000),
 ( 1.000000000000000000, 0.8327032135025188575, 1.000000000000000000),
 ( 1.000000000000000000, 0.7734559727053201827, 1.000000000000000000),
 ( 1.000000000000000000, 0.7377766653992472445, 1.000000000000000000),
 ( 1.000000000000000000, 0.7071067811865522357, 1.000000000000000000) ) ) 
 REPRESENTATION_ITEM ( '' )  SURFACE ( )  );
#18698=CARTESIAN_POINT ( 'NONE',  ( 61.24919886530818758, 0.9685650917412264027, -1.667277206150558966 ) ) ;
#18705=AXIS2_PLACEMENT_3D ( 'NONE', #3958, #3645, #30244 ) ;
#18706=CARTESIAN_POINT ( 'NONE',  ( 50.93312545610843500, -0.6352506689584650479, -1.438808137080897165 ) ) ;
#18707=CARTESIAN_POINT ( 'NONE',  ( 58.65844932252326061, -1.802326573993413561, -0.5172264997589001156 ) ) ;
#18709=CIRCLE ( 'NONE', #19219, 1.875000000000001776 ) ;
#18714=CARTESIAN_POINT ( 'NONE',  ( 61.25000000000000000, 1.800471618824466935, 1.039502773797588597 ) ) ;
#18718=CARTESIAN_POINT ( 'NONE',  ( 51.25000000000001421, 0.9938153758931693726, 1.589954715908409755 ) ) ;
#18726=CARTESIAN_POINT ( 'NONE',  ( 58.65838214097842496, 1.874774200234571087, -0.03350837198745684753 ) ) ;
#18729=AXIS2_PLACEMENT_3D ( 'NONE', #26844, #406, #5293 ) ;
#18732=ORIENTED_EDGE ( 'NONE', *, *, #29449, .F. ) ;
#18740=FACE_OUTER_BOUND ( 'NONE', #5723, .T. ) ;
#18743=CARTESIAN_POINT ( 'NONE',  ( 61.19881854997407800, 0.7436933986918214945, 1.660788881864679212 ) ) ;
#18758=CYLINDRICAL_SURFACE ( 'NONE', #19561, 2.000000000000000000 ) ;
#18772=ORIENTED_EDGE ( 'NONE', *, *, #23699, .T. ) ;
#18774=DIRECTION ( 'NONE',  ( 0.000000000000000000, -1.000000000000000000, 0.000000000000000000 ) ) ;
#18778=DIRECTION ( 'NONE',  ( 1.000000000000000000, 1.047444401652940007E-14, 0.000000000000000000 ) ) ;
#18780=CARTESIAN_POINT ( 'NONE',  ( 58.72419296898077334, 1.293880926823876676, 1.357170036000481916 ) ) ;
#18786=FACE_OUTER_BOUND ( 'NONE', #15595, .T. ) ;
#18792=ORIENTED_EDGE ( 'NONE', *, *, #23122, .T. ) ;
#18796=ORIENTED_EDGE ( 'NONE', *, *, #10028, .F. ) ;
#18801=ORIENTED_EDGE ( 'NONE', *, *, #9337, .F. ) ;
#18803=DIRECTION ( 'NONE',  ( 0.000000000000000000, 0.000000000000000000, 1.000000000000000000 ) ) ;
#18811=CARTESIAN_POINT ( 'NONE',  ( 58.72427158855716556, 1.798991944512857710, -0.5288318043120886491 ) ) ;
#18814=CARTESIAN_POINT ( 'NONE',  ( 51.13341687362767374, 0.9248174436480008920, -1.495576127286106560 ) ) ;
#18829=VERTEX_POINT ( 'NONE', #8667 ) ;
#18831=CARTESIAN_POINT ( 'NONE',  ( 58.64999999999999858, 1.571497941946486065, 1.022750809562083640 ) ) ;
#18834=AXIS2_PLACEMENT_3D ( 'NONE', #16269, #13716, #15939 ) ;
#18835=CARTESIAN_POINT ( 'NONE',  ( 58.75000018803717694, 1.010830333487790167, -1.651902078982614208 ) ) ;
#18842=CARTESIAN_POINT ( 'NONE',  ( 61.09423418604048095, 0.6373668173476213505, -1.895722432252298084 ) ) ;
#18850=AXIS2_PLACEMENT_3D ( 'NONE', #997, #13467, #28650 ) ;
#18852=VERTEX_POINT ( 'NONE', #16607 ) ;
#18853=EDGE_CURVE ( 'NONE', #19651, #19672, #14458, .T. ) ;
#18864=EDGE_LOOP ( 'NONE', ( #24315, #18, #18139, #19710 ) ) ;
#18866=CARTESIAN_POINT ( 'NONE',  ( 61.23770293222996486, -0.8897917884435792013, -1.791164585742600179 ) ) ;
#18867=CARTESIAN_POINT ( 'NONE',  ( 51.45655683570191741, -0.9591657938390835136, 1.518428463906027037 ) ) ;
#18876=EDGE_LOOP ( 'NONE', ( #16007, #6455, #19735, #19325, #20966, #1620 ) ) ;
#18878=ORIENTED_EDGE ( 'NONE', *, *, #4131, .F. ) ;
#18884=ORIENTED_EDGE ( 'NONE', *, *, #25955, .F. ) ;
#18885=EDGE_CURVE ( 'NONE', #6477, #26303, #20762, .T. ) ;
#18890=CIRCLE ( 'NONE', #3698, 0.1000000000000001166 ) ;
#18893=CIRCLE ( 'NONE', #7748, 2.000000000000000000 ) ;
#18894=CARTESIAN_POINT ( 'NONE',  ( 50.25000000000000711, 1.323060376181234510, 1.499837071479058981 ) ) ;
#18900=CARTESIAN_POINT ( 'NONE',  ( 58.75000000000003553, -1.749377236608634645, -0.8979909453698914357 ) ) ;
#18901=EDGE_CURVE ( 'NONE', #27318, #26116, #4854, .T. ) ;
#18903=CARTESIAN_POINT ( 'NONE',  ( 61.05375305192653457, -0.5989395831096625544, 1.861793349153599397 ) ) ;
#18909=ORIENTED_EDGE ( 'NONE', *, *, #6982, .F. ) ;
#18911=AXIS2_PLACEMENT_3D ( 'NONE', #16099, #23531, #18004 ) ;
#18920=CARTESIAN_POINT ( 'NONE',  ( 58.75000018595672202, -1.651828233789423450, 1.011330950598698042 ) ) ;
#18928=B_SPLINE_CURVE_WITH_KNOTS ( 'NONE', 3,
 ( #22687, #1266, #29786, #15371, #25195, #10934 ),
 .UNSPECIFIED., .F., .F.,
 ( 4, 2, 4 ),
 ( 0.000000000000000000, 0.0001000270069610021377, 0.0002000540139220042754 ),
 .UNSPECIFIED. ) ;
#18934=B_SPLINE_CURVE_WITH_KNOTS ( 'NONE', 3,
 ( #1143, #17934, #30415, #29805, #10795, #25680 ),
 .UNSPECIFIED., .F., .F.,
 ( 4, 2, 4 ),
 ( 0.000000000000000000, 0.0001000270069610654009, 0.0002000540139221308018 ),
 .UNSPECIFIED. ) ;
#18940=CARTESIAN_POINT ( 'NONE',  ( 58.74999981196285859, -1.050519579371408829, 1.649561145038723531 ) ) ;
#18952=FACE_OUTER_BOUND ( 'NONE', #27102, .T. ) ;
#18954=VERTEX_POINT ( 'NONE', #21684 ) ;
#18955=ADVANCED_FACE ( 'NONE', ( #14528 ), #124, .F. ) ;
#18964=ORIENTED_EDGE ( 'NONE', *, *, #22731, .T. ) ;
#18966=CARTESIAN_POINT ( 'NONE',  ( 58.64999999999999147, 1.782657835995388629, -0.5811678240976841936 ) ) ;
#18973=CARTESIAN_POINT ( 'NONE',  ( 58.65000000000001279, 0.5811678240972328879, 1.782657835995121287 ) ) ;
#18977=CARTESIAN_POINT ( 'NONE',  ( 58.75000000000003553, -1.800471618824714071, 1.039502773796719959 ) ) ;
#18978=AXIS2_PLACEMENT_3D ( 'NONE', #9094, #14620, #1965 ) ;
#18979=ORIENTED_EDGE ( 'NONE', *, *, #19459, .F. ) ;
#18981=DIRECTION ( 'NONE',  ( -0.8262273428075540549, 0.5633368246415005887, 0.000000000000000000 ) ) ;
#18982=DIRECTION ( 'NONE',  ( 0.000000000000000000, 0.000000000000000000, 1.000000000000000000 ) ) ;
#18987=DIRECTION ( 'NONE',  ( 0.7542528389311764503, -0.5142632992712440343, 0.4082106245394847011 ) ) ;
#18988=DIRECTION ( 'NONE',  ( -1.000000000000000000, -1.018631342913014973E-14, -0.000000000000000000 ) ) ;
#18989=DIRECTION ( 'NONE',  ( 0.000000000000000000, 0.000000000000000000, 1.000000000000000000 ) ) ;
#18993=DIRECTION ( 'NONE',  ( 1.000000000000000000, 1.047444401652940007E-14, -0.000000000000000000 ) ) ;
#18997=CARTESIAN_POINT ( 'NONE',  ( 58.75000018595670070, 1.011330950599250711, 1.651828233789864875 ) ) ;
#18999=ORIENTED_EDGE ( 'NONE', *, *, #3174, .T. ) ;
#19008=EDGE_LOOP ( 'NONE', ( #23378, #11320, #16524, #4995 ) ) ;
#19019=DIRECTION ( 'NONE',  ( 1.000000000000000000, 1.047444401652940007E-14, 0.000000000000000000 ) ) ;
#19029=ORIENTED_EDGE ( 'NONE', *, *, #4397, .F. ) ;
#19037=CARTESIAN_POINT ( 'NONE',  ( 58.72419296898063124, 1.874576113084453821, 0.04475215827456610618 ) ) ;
#19040=CIRCLE ( 'NONE', #5360, 2.000000000000000000 ) ;
#19043=EDGE_LOOP ( 'NONE', ( #5337, #12238, #1433, #14375, #6051, #22382 ) ) ;
#19051=CARTESIAN_POINT ( 'NONE',  ( 58.75000000000002132, 6.153735859711025284E-13, 3.111507638930570854E-58 ) ) ;
#19056=AXIS2_PLACEMENT_3D ( 'NONE', #30325, #1509, #3886 ) ;
#19071=CIRCLE ( 'NONE', #27641, 2.000000000000000000 ) ;
#19072=EDGE_LOOP ( 'NONE', ( #9680, #22673, #16816, #28495 ) ) ;
#19078=ORIENTED_EDGE ( 'NONE', *, *, #182, .T. ) ;
#19097=CARTESIAN_POINT ( 'NONE',  ( 51.23644008536124517, -1.080112125195908046, 1.214076932077873039 ) ) ;
#19100=CIRCLE ( 'NONE', #17065, 0.2500000000000002776 ) ;
#19102=CARTESIAN_POINT ( 'NONE',  ( 58.75000006180463430, -0.5511536957112744828, -1.849318015437667828 ) ) ;
#19103=DIRECTION ( 'NONE',  ( 0.000000000000000000, 1.000000000000000000, 0.000000000000000000 ) ) ;
#19105=DIRECTION ( 'NONE',  ( 1.000000000000000000, 1.047444401652940007E-14, 0.000000000000000000 ) ) ;
#19106=CARTESIAN_POINT ( 'NONE',  ( 58.65000000000003411, -1.671477153793470949, 0.8495817349404535257 ) ) ;
#19109=AXIS2_PLACEMENT_3D ( 'NONE', #8555, #15538, #805 ) ;
#19111=ORIENTED_EDGE ( 'NONE', *, *, #3445, .F. ) ;
#19123=ORIENTED_EDGE ( 'NONE', *, *, #16643, .F. ) ;
#19125=CIRCLE ( 'NONE', #31239, 0.1500000000000000777 ) ;
#19128=CIRCLE ( 'NONE', #24655, 0.1000000000000000611 ) ;
#19129=VERTEX_POINT ( 'NONE', #8491 ) ;
#19132=VERTEX_POINT ( 'NONE', #22435 ) ;
#19141=B_SPLINE_CURVE_WITH_KNOTS ( 'NONE', 3,
 ( #19956, #27232, #5544, #12804 ),
 .UNSPECIFIED., .F., .F.,
 ( 4, 4 ),
 ( 2.168404344971008627E-19, 0.0001476506082772709844 ),
 .UNSPECIFIED. ) ;
#19143=CARTESIAN_POINT ( 'NONE',  ( 58.75000000000001421, 0.6373668173475968146, -1.895722432252298084 ) ) ;
#19145=AXIS2_PLACEMENT_3D ( 'NONE', #6452, #27670, #25291 ) ;
#19147=ORIENTED_EDGE ( 'NONE', *, *, #30200, .F. ) ;
#19149=ADVANCED_FACE ( 'NONE', ( #29865 ), #26364, .T. ) ;
#19151=DIRECTION ( 'NONE',  ( 1.000000000000000000, 1.047444401652940007E-14, 0.000000000000000000 ) ) ;
#19159=CARTESIAN_POINT ( 'NONE',  ( 58.65263613458535019, 0.8791532451977436269, -1.656197658588938193 ) ) ;
#19166=CARTESIAN_POINT ( 'NONE',  ( 58.66054497608116947, -0.4999999999856035160, 1.807104036853935503 ) ) ;
#19167=CARTESIAN_POINT ( 'NONE',  ( 58.75000000000000711, 0.8948927608033926395, 1.760622601997029690 ) ) ;
#19170=CARTESIAN_POINT ( 'NONE',  ( 61.24141714606658127, 0.9075239022126483368, 1.727282253938982270 ) ) ;
#19177=DIRECTION ( 'NONE',  ( 0.000000000000000000, 0.7438053426813423519, 0.6683962987619627150 ) ) ;
#19178=ORIENTED_EDGE ( 'NONE', *, *, #28214, .T. ) ;
#19183=EDGE_CURVE ( 'NONE', #4826, #26557, #19261, .T. ) ;
#19188=EDGE_CURVE ( 'NONE', #22535, #4925, #6590, .T. ) ;
#19192=VERTEX_POINT ( 'NONE', #6269 ) ;
#19194=CARTESIAN_POINT ( 'NONE',  ( 58.66107449606997903, 0.9668599424584182200, -1.606832818401373375 ) ) ;
#19196=DIRECTION ( 'NONE',  ( 0.000000000000000000, 0.000000000000000000, 1.000000000000000000 ) ) ;
#19199=VERTEX_POINT ( 'NONE', #2426 ) ;
#19219=AXIS2_PLACEMENT_3D ( 'NONE', #11293, #23496, #6406 ) ;
#19226=FACE_OUTER_BOUND ( 'NONE', #9204, .T. ) ;
#19229=( BOUNDED_SURFACE ( )  B_SPLINE_SURFACE ( 3, 2, ( 
 ( #1931, #21419, #21110 ),
 ( #30904, #30749, #11592 ),
 ( #9055, #21274, #9219 ),
 ( #2081, #26151, #18726 ),
 ( #28522, #25831, #11744 ),
 ( #6829, #31221, #14111 ),
 ( #13775, #19037, #16669 ),
 ( #9547, #28845, #7158 ),
 ( #8876, #28371, #18567 ),
 ( #23312, #23937, #16337 ) ),
 .UNSPECIFIED., .F., .F., .F. ) 
 B_SPLINE_SURFACE_WITH_KNOTS ( ( 4, 2, 2, 2, 4 ),
 ( 3, 3 ),
 ( 0.0001706658715691949555, 0.0002229276920778155090, 0.0002751895125864360354, 0.0003274513330950565618, 0.0003797131536036770882 ),
 ( 0.000000000000000000, 1.000000000000000000 ),
 .UNSPECIFIED. ) 
 GEOMETRIC_REPRESENTATION_ITEM ( )  RATIONAL_B_SPLINE_SURFACE ( (
 ( 1.000000000000000000, 0.7071067811865214825, 1.000000000000000000),
 ( 1.000000000000000000, 0.7375607040702809591, 1.000000000000000000),
 ( 1.000000000000000000, 0.7730431127428194493, 1.000000000000000000),
 ( 1.000000000000000000, 0.8321012486990639889, 1.000000000000000000),
 ( 1.000000000000000000, 0.8541932017412365852, 1.000000000000000000),
 ( 1.000000000000000000, 0.8545723906067121955, 1.000000000000000000),
 ( 1.000000000000000000, 0.8327032135054380779, 1.000000000000000000),
 ( 1.000000000000000000, 0.7734559727063156087, 1.000000000000000000),
 ( 1.000000000000000000, 0.7377766653997859247, 1.000000000000000000),
 ( 1.000000000000000000, 0.7071067811865229258, 1.000000000000000000) ) ) 
 REPRESENTATION_ITEM ( '' )  SURFACE ( )  );
#19233=CARTESIAN_POINT ( 'NONE',  ( 58.64999999999992042, -1.469015551795658681, -1.320082690054208419 ) ) ;
#19239=CARTESIAN_POINT ( 'NONE',  ( 60.87284881435257944, 0.5000000998574327671, -1.554802432719798011 ) ) ;
#19241=ORIENTED_EDGE ( 'NONE', *, *, #14452, .F. ) ;
#19249=CARTESIAN_POINT ( 'NONE',  ( 58.65000000000001990, 6.143261415694495821E-13, 3.111507638930570854E-58 ) ) ;
#19256=CARTESIAN_POINT ( 'NONE',  ( 58.74154451056421067, -0.8556855217782239897, -1.668374833163418947 ) ) ;
#19261=B_SPLINE_CURVE_WITH_KNOTS ( 'NONE', 3,
 ( #30475, #4052, #28278, #20847 ),
 .UNSPECIFIED., .F., .F.,
 ( 4, 4 ),
 ( 0.000000000000000000, 0.0002184312136277828859 ),
 .UNSPECIFIED. ) ;
#19263=CARTESIAN_POINT ( 'NONE',  ( 58.65000038048066955, -0.8644232797868882656, 1.663933463835922666 ) ) ;
#19269=ORIENTED_EDGE ( 'NONE', *, *, #10358, .F. ) ;
#19271=CARTESIAN_POINT ( 'NONE',  ( 58.66595318830225381, 0.5000000000006145084, -1.807217177072659275 ) ) ;
#19273=PLANE ( 'NONE',  #25847 ) ;
#19286=EDGE_CURVE ( 'NONE', #29981, #6604, #11500, .T. ) ;
#19288=AXIS2_PLACEMENT_3D ( 'NONE', #17469, #24894, #528 ) ;
#19299=VERTEX_POINT ( 'NONE', #8953 ) ;
#19304=ADVANCED_FACE ( 'NONE', ( #19226 ), #28867, .F. ) ;
#19313=DIRECTION ( 'NONE',  ( 0.000000000000000000, 0.000000000000000000, 1.000000000000000000 ) ) ;
#19321=AXIS2_PLACEMENT_3D ( 'NONE', #12282, #9632, #11992 ) ;
#19322=DIRECTION ( 'NONE',  ( -0.7542528389311653481, -0.5142632992712595774, -0.4082106245394850341 ) ) ;
#19325=ORIENTED_EDGE ( 'NONE', *, *, #18301, .T. ) ;
#19326=EDGE_CURVE ( 'NONE', #28946, #12544, #20907, .T. ) ;
#19332=EDGE_CURVE ( 'NONE', #10573, #29731, #2833, .T. ) ;
#19337=DIRECTION ( 'NONE',  ( 5.585208838990483560E-16, -0.05332224631853142716, -0.9985773570673159849 ) ) ;
#19338=CARTESIAN_POINT ( 'NONE',  ( 58.75000000000002132, -0.6121634413829184496, -1.877732920580952980 ) ) ;
#19342=LINE ( 'NONE', #21406, #675 ) ;
#19344=CARTESIAN_POINT ( 'NONE',  ( 58.75000000000000711, 1.039502773797200019, -1.800471618823823450 ) ) ;
#19345=CARTESIAN_POINT ( 'NONE',  ( 52.06628335902946247, -0.5434431642975677823, -1.718465885608440713 ) ) ;
#19354=ORIENTED_EDGE ( 'NONE', *, *, #7132, .F. ) ;
#19356=PLANE ( 'NONE',  #4084 ) ;
#19361=ORIENTED_EDGE ( 'NONE', *, *, #17564, .T. ) ;
#19364=ORIENTED_EDGE ( 'NONE', *, *, #15227, .T. ) ;
#19375=VERTEX_POINT ( 'NONE', #26647 ) ;
#19388=EDGE_CURVE ( 'NONE', #26655, #7417, #16503, .T. ) ;
#19390=EDGE_LOOP ( 'NONE', ( #3630, #28746, #30100, #1138, #28253, #5802, #17799, #8727 ) ) ;
#19394=EDGE_LOOP ( 'NONE', ( #27420, #22198, #10320, #20042, #8302, #28417 ) ) ;
#19402=CARTESIAN_POINT ( 'NONE',  ( 58.65000000000002700, -1.022750809560353469, -1.571497941946597976 ) ) ;
#19403=CARTESIAN_POINT ( 'NONE',  ( 58.75000000000002132, 6.153735859711025284E-13, 3.111507638930570854E-58 ) ) ;
#19407=FACE_OUTER_BOUND ( 'NONE', #2184, .T. ) ;
#19408=CARTESIAN_POINT ( 'NONE',  ( 51.55144386500324316, 1.037443573995146862, 1.251214392908886142 ) ) ;
#19412=EDGE_LOOP ( 'NONE', ( #19702, #8685, #5807, #4502, #16220 ) ) ;
#19414=VERTEX_POINT ( 'NONE', #2583 ) ;
#19417=DIRECTION ( 'NONE',  ( 1.047444401652940007E-14, -1.000000000000000000, 0.000000000000000000 ) ) ;
#19423=CARTESIAN_POINT ( 'NONE',  ( 60.97408713704741956, 0.7545809820805179369, -1.439897579195099864 ) ) ;
#19428=CARTESIAN_POINT ( 'NONE',  ( 58.65000000000003411, -1.671477153793470949, 0.8495817349404535257 ) ) ;
#19429=EDGE_CURVE ( 'NONE', #29589, #1037, #14755, .T. ) ;
#19430=ORIENTED_EDGE ( 'NONE', *, *, #23787, .T. ) ;
#19432=DIRECTION ( 'NONE',  ( 0.000000000000000000, 0.000000000000000000, 1.000000000000000000 ) ) ;
#19442=DIRECTION ( 'NONE',  ( 1.000000000000000000, 1.047444401652940007E-14, 0.000000000000000000 ) ) ;
#19443=ORIENTED_EDGE ( 'NONE', *, *, #5015, .T. ) ;
#19447=CARTESIAN_POINT ( 'NONE',  ( 58.65000000000000568, 1.253243060178336643, -1.394635017528379928 ) ) ;
#19455=CARTESIAN_POINT ( 'NONE',  ( 58.75000000000000711, 1.077297519405725712, -1.655311165516502703 ) ) ;
#19458=CARTESIAN_POINT ( 'NONE',  ( 51.59739104186227365, 1.010292945603182169, -1.272765950230260401 ) ) ;
#19459=EDGE_CURVE ( 'NONE', #2526, #28401, #8404, .T. ) ;
#19461=DIRECTION ( 'NONE',  ( 0.000000000000000000, -0.4531102586355347794, 0.8914544820231926625 ) ) ;
#19463=ORIENTED_EDGE ( 'NONE', *, *, #23340, .T. ) ;
#19468=CARTESIAN_POINT ( 'NONE',  ( 60.75000000000002842, -0.4999999999993638977, 1.718465885608440047 ) ) ;
#19469=LINE ( 'NONE', #2819, #7861 ) ;
#19475=CARTESIAN_POINT ( 'NONE',  ( 61.21684424624501730, 0.7974861228896987786, -1.837019011344032782 ) ) ;
#19483=CARTESIAN_POINT ( 'NONE',  ( 51.25000000000002842, -0.6499999999994634514, -1.489337100860647967 ) ) ;
#19484=CYLINDRICAL_SURFACE ( 'NONE', #5395, 2.000000000000000000 ) ;
#19486=CARTESIAN_POINT ( 'NONE',  ( 58.64999999999999858, 0.9947034709632315286, -1.589751505945539378 ) ) ;
#19495=TOROIDAL_SURFACE ( 'NONE', #5833, 1.975000000000001865, 0.1000000000000000056 ) ;
#19504=ORIENTED_EDGE ( 'NONE', *, *, #7021, .F. ) ;
#19507=CARTESIAN_POINT ( 'NONE',  ( 58.75000000000003553, -1.457351493771257722, -1.320164791809644411 ) ) ;
#19514=CARTESIAN_POINT ( 'NONE',  ( 61.00000000000003553, -0.9999999999993611777, -1.586072192556190252 ) ) ;
#19533=EDGE_CURVE ( 'NONE', #6367, #28516, #14996, .T. ) ;
#19538=EDGE_LOOP ( 'NONE', ( #17462, #18319, #8495, #13943, #7333, #1883, #6206, #6313, #31004, #20596, #12765, #10565 ) ) ;
#19544=ORIENTED_EDGE ( 'NONE', *, *, #2933, .F. ) ;
#19561=AXIS2_PLACEMENT_3D ( 'NONE', #9248, #28552, #16850 ) ;
#19564=CARTESIAN_POINT ( 'NONE',  ( 50.25000000000002842, -1.039502773796191937, -1.800471618824325493 ) ) ;
#19568=DIRECTION ( 'NONE',  ( 1.000000000000000000, 1.047444401652940007E-14, 0.000000000000000000 ) ) ;
#19569=B_SPLINE_CURVE_WITH_KNOTS ( 'NONE', 3,
 ( #10211, #24005, #21811, #19880 ),
 .UNSPECIFIED., .F., .F.,
 ( 4, 4 ),
 ( 1.084202172485504434E-19, 0.0001521069361438105792 ),
 .UNSPECIFIED. ) ;
#19573=CARTESIAN_POINT ( 'NONE',  ( 51.19148447764911225, 0.9872860527330414859, 1.295557643792421443 ) ) ;
#19574=EDGE_CURVE ( 'NONE', #26557, #18608, #16528, .T. ) ;
#19576=CARTESIAN_POINT ( 'NONE',  ( 58.75000000000002132, 6.153735859711025284E-13, 3.111507638930570854E-58 ) ) ;
#19577=EDGE_LOOP ( 'NONE', ( #19241, #8721, #27501, #25871, #5693, #14988 ) ) ;
#19583=CIRCLE ( 'NONE', #6939, 0.09999999999999997780 ) ;
#19586=DIRECTION ( 'NONE',  ( 0.000000000000000000, 0.000000000000000000, 1.000000000000000000 ) ) ;
#19587=CYLINDRICAL_SURFACE ( 'NONE', #2863, 0.2500000000000000000 ) ;
#19591=EDGE_LOOP ( 'NONE', ( #5120, #27274, #27060, #29097, #13668, #9320 ) ) ;
#19593=DIRECTION ( 'NONE',  ( 0.000000000000000000, 0.000000000000000000, 1.000000000000000000 ) ) ;
#19597=DIRECTION ( 'NONE',  ( 0.5633368246415185743, -0.8262273428075417314, 0.000000000000000000 ) ) ;
#19600=AXIS2_PLACEMENT_3D ( 'NONE', #30971, #9289, #21488 ) ;
#19611=EDGE_CURVE ( 'NONE', #6604, #21318, #18070, .T. ) ;
#19624=LINE ( 'NONE', #24353, #7087 ) ;
#19630=FACE_OUTER_BOUND ( 'NONE', #25349, .T. ) ;
#19649=DIRECTION ( 'NONE',  ( 0.000000000000000000, 0.000000000000000000, 1.000000000000000000 ) ) ;
#19651=VERTEX_POINT ( 'NONE', #13759 ) ;
#19656=CARTESIAN_POINT ( 'NONE',  ( 58.75000000000004263, -2.008165151418373373, -0.5380862305909229759 ) ) ;
#19658=ORIENTED_EDGE ( 'NONE', *, *, #19286, .F. ) ;
#19661=CARTESIAN_POINT ( 'NONE',  ( 51.14630318392407560, -0.9364487020629673752, -1.503522130792586564 ) ) ;
#19664=ORIENTED_EDGE ( 'NONE', *, *, #14286, .T. ) ;
#19672=VERTEX_POINT ( 'NONE', #16473 ) ;
#19681=CARTESIAN_POINT ( 'NONE',  ( 50.59602332238209499, -0.1408342061598477080, -1.212874140286674507 ) ) ;
#19684=( BOUNDED_CURVE ( )  B_SPLINE_CURVE ( 3, ( #20903, #18534, #13029, #11383 ),
 .UNSPECIFIED., .F., .T. ) 
 B_SPLINE_CURVE_WITH_KNOTS ( ( 4, 4 ),
 ( 1.982313172862385064, 2.241731514487932397 ),
 .UNSPECIFIED. ) 
 CURVE ( )  GEOMETRIC_REPRESENTATION_ITEM ( )  RATIONAL_B_SPLINE_CURVE ( ( 1.000000000000000000, 0.9943997021150919879, 0.9943997021150919879, 1.000000000000000000 ) ) 
 REPRESENTATION_ITEM ( '' )  );
#19686=DIRECTION ( 'NONE',  ( 0.000000000000000000, 0.000000000000000000, 1.000000000000000000 ) ) ;
#19697=ORIENTED_EDGE ( 'NONE', *, *, #24833, .F. ) ;
#19699=EDGE_CURVE ( 'NONE', #20276, #19192, #23445, .T. ) ;
#19702=ORIENTED_EDGE ( 'NONE', *, *, #16141, .T. ) ;
#19703=ORIENTED_EDGE ( 'NONE', *, *, #9189, .F. ) ;
#19710=ORIENTED_EDGE ( 'NONE', *, *, #29139, .F. ) ;
#19719=CARTESIAN_POINT ( 'NONE',  ( 58.65263613458539993, -0.9947326234269614487, -1.589467873454827984 ) ) ;
#19722=( BOUNDED_SURFACE ( )  B_SPLINE_SURFACE ( 3, 2, ( 
 ( #20382, #24939, #30003 ),
 ( #8320, #15621, #13219 ),
 ( #4350, #1649, #1352 ),
 ( #21172, #28269, #14003 ) ),
 .UNSPECIFIED., .F., .F., .F. ) 
 B_SPLINE_SURFACE_WITH_KNOTS ( ( 4, 4 ),
 ( 3, 3 ),
 ( 0.0002753388251011180433, 0.0003797131536021330217 ),
 ( 0.000000000000000000, 1.000000000000000000 ),
 .UNSPECIFIED. ) 
 GEOMETRIC_REPRESENTATION_ITEM ( )  RATIONAL_B_SPLINE_SURFACE ( (
 ( 1.000000000000000000, 0.8543839308450231762, 1.000000000000000000),
 ( 1.000000000000000000, 0.8547349261747320126, 1.000000000000000000),
 ( 1.000000000000000000, 0.7665921203078746027, 1.000000000000000000),
 ( 1.000000000000000000, 0.7071067811865738850, 1.000000000000000000) ) ) 
 REPRESENTATION_ITEM ( '' )  SURFACE ( )  );
#19723=CIRCLE ( 'NONE', #5030, 0.09999999999999990841 ) ;
#19724=CARTESIAN_POINT ( 'NONE',  ( 52.20711756518984004, -0.4999999999994533817, -1.996089927833914146 ) ) ;
#19726=ADVANCED_FACE ( 'NONE', ( #24688 ), #19484, .T. ) ;
#19727=PRODUCT_DEFINITION_FORMATION_WITH_SPECIFIED_SOURCE ( 'ANY', '', #22213, .NOT_KNOWN. ) ;
#19732=CARTESIAN_POINT ( 'NONE',  ( 61.24141714606679443, -0.9075239022123753330, -1.727282253937962198 ) ) ;
#19735=ORIENTED_EDGE ( 'NONE', *, *, #6511, .F. ) ;
#19745=FACE_OUTER_BOUND ( 'NONE', #13921, .T. ) ;
#19757=AXIS2_PLACEMENT_3D ( 'NONE', #26025, #9262, #26199 ) ;
#19758=CARTESIAN_POINT ( 'NONE',  ( 58.75000000000000000, 2.008165151418861427, -0.5380862305899540843 ) ) ;
#19772=ORIENTED_EDGE ( 'NONE', *, *, #26582, .T. ) ;
#19781=EDGE_CURVE ( 'NONE', #25278, #27496, #25098, .T. ) ;
#19786=FACE_OUTER_BOUND ( 'NONE', #26810, .T. ) ;
#19787=ORIENTED_EDGE ( 'NONE', *, *, #7979, .T. ) ;
#19791=DIRECTION ( 'NONE',  ( 0.000000000000000000, 0.5454670984325526994, -0.8381322357048270888 ) ) ;
#19793=CARTESIAN_POINT ( 'NONE',  ( 61.25000000000000000, 2.079005547593442582, 1.004182178118534636E-12 ) ) ;
#19794=DIRECTION ( 'NONE',  ( 1.000000000000000000, 1.047444401652940007E-14, 0.000000000000000000 ) ) ;
#19795=VERTEX_POINT ( 'NONE', #16423 ) ;
#19796=DIRECTION ( 'NONE',  ( 1.000000000000000000, 1.047444401652940007E-14, 0.000000000000000000 ) ) ;
#19798=CARTESIAN_POINT ( 'NONE',  ( 52.06628335902946247, -0.5434431642975682264, -1.794517909405659806 ) ) ;
#19799=DIRECTION ( 'NONE',  ( -1.000000000000000000, -1.047444401652940007E-14, -0.000000000000000000 ) ) ;
#19805=CARTESIAN_POINT ( 'NONE',  ( 51.23017468167498123, -0.9889849352709336738, -1.419511492616531978 ) ) ;
#19807=CARTESIAN_POINT ( 'NONE',  ( 51.50435016707358926, 0.9265794315412906323, 1.339215852266870010 ) ) ;
#19828=DIRECTION ( 'NONE',  ( 1.000000000000000000, 1.047444401652940007E-14, 0.000000000000000000 ) ) ;
#19833=EDGE_LOOP ( 'NONE', ( #18613, #3202, #23973, #18677, #17742, #24656 ) ) ;
#19841=VERTEX_POINT ( 'NONE', #4852 ) ;
#19842=CARTESIAN_POINT ( 'NONE',  ( 58.75000000000002132, 6.153735859711025284E-13, 3.111507638930570854E-58 ) ) ;
#19851=ORIENTED_EDGE ( 'NONE', *, *, #21686, .F. ) ;
#19857=ORIENTED_EDGE ( 'NONE', *, *, #27876, .T. ) ;
#19862=AXIS2_PLACEMENT_3D ( 'NONE', #12311, #17245, #7262 ) ;
#19872=ORIENTED_EDGE ( 'NONE', *, *, #1533, .T. ) ;
#19875=ORIENTED_EDGE ( 'NONE', *, *, #26237, .T. ) ;
#19876=CARTESIAN_POINT ( 'NONE',  ( 60.75000000000002842, -0.4999999999993638977, -1.863080903343643069 ) ) ;
#19877=CIRCLE ( 'NONE', #4699, 2.000000000000000000 ) ;
#19880=CARTESIAN_POINT ( 'NONE',  ( 51.31572262954152563, 1.002608958138273554, -1.584424273060082378 ) ) ;
#19895=CARTESIAN_POINT ( 'NONE',  ( 58.65000000000001990, 6.143261415694495821E-13, 3.111507638930570854E-58 ) ) ;
#19901=DIRECTION ( 'NONE',  ( -1.000000000000000000, -1.047444401652940007E-14, -0.000000000000000000 ) ) ;
#19904=CARTESIAN_POINT ( 'NONE',  ( 58.75000000000000711, 1.470078920828144620, -1.470078920826818125 ) ) ;
#19906=CARTESIAN_POINT ( 'NONE',  ( 51.31802667458096323, -1.005866567096536546, 1.281163073955422504 ) ) ;
#19908=EDGE_CURVE ( 'NONE', #26840, #29149, #3553, .T. ) ;
#19922=CARTESIAN_POINT ( 'NONE',  ( 61.25000000000003553, -0.8666666666660259866, -1.374595900215366040 ) ) ;
#19924=ORIENTED_EDGE ( 'NONE', *, *, #7359, .T. ) ;
#19925=DIRECTION ( 'NONE',  ( 8.450433050631136626E-15, -0.6683962987616075546, -0.7438053426816615410 ) ) ;
#19932=CARTESIAN_POINT ( 'NONE',  ( 58.65263613458534309, 1.589467873455502778, -0.9947326234274815882 ) ) ;
#19934=CARTESIAN_POINT ( 'NONE',  ( 58.65000000000001990, 6.143261415694495821E-13, 3.111507638930570854E-58 ) ) ;
#19935=LINE ( 'NONE', #12317, #22479 ) ;
#19936=FACE_OUTER_BOUND ( 'NONE', #24462, .T. ) ;
#19944=CARTESIAN_POINT ( 'NONE',  ( 58.75000000000001421, 0.4991218602018681061, 1.863314270026655395 ) ) ;
#19948=UNCERTAINTY_MEASURE_WITH_UNIT (LENGTH_MEASURE( 1.000000000000000082E-05 ), #5741, 'distance_accuracy_value', 'NONE');
#19956=CARTESIAN_POINT ( 'NONE',  ( 51.25000000000002842, -0.9938153758920951208, 1.589954715908409977 ) ) ;
#19965=CARTESIAN_POINT ( 'NONE',  ( 58.75000018595672913, -1.404395290251533313, -1.333791840693540731 ) ) ;
#19966=CIRCLE ( 'NONE', #15413, 0.2500000000000002776 ) ;
#19971=PLANE ( 'NONE',  #15669 ) ;
#19978=CARTESIAN_POINT ( 'NONE',  ( 51.25000000000001421, 0.9938153758931693726, -1.589954715908409755 ) ) ;
#19984=CARTESIAN_POINT ( 'NONE',  ( 58.64999999999999858, 1.834410884276644227, -0.3880228184651523526 ) ) ;
#20000=PRESENTATION_STYLE_ASSIGNMENT (( #15565 ) ) ;
#20028=EDGE_CURVE ( 'NONE', #29149, #30150, #24116, .T. ) ;
#20040=ORIENTED_EDGE ( 'NONE', *, *, #4106, .T. ) ;
#20041=AXIS2_PLACEMENT_3D ( 'NONE', #24026, #19442, #31307 ) ;
#20042=ORIENTED_EDGE ( 'NONE', *, *, #20443, .F. ) ;
#20050=ORIENTED_EDGE ( 'NONE', *, *, #4817, .F. ) ;
#20053=( BOUNDED_SURFACE ( )  B_SPLINE_SURFACE ( 3, 2, ( 
 ( #5276, #14929, #19402 ),
 ( #12256, #7205, #24301 ),
 ( #12401, #21941, #19719 ),
 ( #17183, #385, #14783 ),
 ( #16719, #11952, #16869 ),
 ( #7056, #26967, #21637 ),
 ( #9741, #31271, #7521 ),
 ( #2754, #29044, #9596 ),
 ( #11792, #19256, #4663 ),
 ( #2130, #17323, #9428 ) ),
 .UNSPECIFIED., .F., .F., .F. ) 
 B_SPLINE_SURFACE_WITH_KNOTS ( ( 4, 2, 2, 2, 4 ),
 ( 3, 3 ),
 ( 0.0001706658715697745971, 0.0002229276920781411762, 0.0002751895125865077554, 0.0003274513330948743074, 0.0003797131536032408595 ),
 ( 0.000000000000000000, 1.000000000000000000 ),
 .UNSPECIFIED. ) 
 GEOMETRIC_REPRESENTATION_ITEM ( )  RATIONAL_B_SPLINE_SURFACE ( (
 ( 1.000000000000000000, 0.7071067811873460451, 1.000000000000000000),
 ( 1.000000000000000000, 0.7375607040709752926, 1.000000000000000000),
 ( 1.000000000000000000, 0.7730431127433748939, 1.000000000000000000),
 ( 1.000000000000000000, 0.8321012486987983126, 1.000000000000000000),
 ( 1.000000000000000000, 0.8541932017406910216, 1.000000000000000000),
 ( 1.000000000000000000, 0.8545723906054343288, 1.000000000000000000),
 ( 1.000000000000000000, 0.8327032135043206384, 1.000000000000000000),
 ( 1.000000000000000000, 0.7734559727060463796, 1.000000000000000000),
 ( 1.000000000000000000, 0.7377766653994621837, 1.000000000000000000),
 ( 1.000000000000000000, 0.7071067811865494601, 1.000000000000000000) ) ) 
 REPRESENTATION_ITEM ( '' )  SURFACE ( )  );
#20054=CARTESIAN_POINT ( 'NONE',  ( 51.15394434968256121, -0.9591183795338193985, 1.387856512383045970 ) ) ;
#20057=AXIS2_PLACEMENT_3D ( 'NONE', #18403, #25364, #20328 ) ;
#20065=AXIS2_PLACEMENT_3D ( 'NONE', #8600, #18276, #22725 ) ;
#20066=DIRECTION ( 'NONE',  ( 0.000000000000000000, 0.000000000000000000, 1.000000000000000000 ) ) ;
#20076=DIRECTION ( 'NONE',  ( 0.000000000000000000, 0.000000000000000000, 1.000000000000000000 ) ) ;
#20082=DIRECTION ( 'NONE',  ( 0.000000000000000000, 0.000000000000000000, 1.000000000000000000 ) ) ;
#20090=CARTESIAN_POINT ( 'NONE',  ( 61.25000000000004263, -2.079005547593161918, 1.932245437381540134E-15 ) ) ;
#20093=ORIENTED_EDGE ( 'NONE', *, *, #11052, .F. ) ;
#20096=ORIENTED_EDGE ( 'NONE', *, *, #2038, .T. ) ;
#20105=SPHERICAL_SURFACE ( 'NONE', #16993, 0.2500000000000000000 ) ;
#20110=CIRCLE ( 'NONE', #24150, 0.1500000000000002720 ) ;
#20113=VECTOR ( 'NONE', #18095, 1000.000000000000000 ) ;
#20121=AXIS2_PLACEMENT_3D ( 'NONE', #22622, #8970, #21349 ) ;
#20123=AXIS2_PLACEMENT_3D ( 'NONE', #1054, #5972, #25271 ) ;
#20125=CIRCLE ( 'NONE', #9424, 1.875000000000001776 ) ;
#20127=LINE ( 'NONE', #8221, #8426 ) ;
#20136=CYLINDRICAL_SURFACE ( 'NONE', #26070, 0.2500000000000000000 ) ;
#20138=CYLINDRICAL_SURFACE ( 'NONE', #16237, 2.000000000000000000 ) ;
#20141=CARTESIAN_POINT ( 'NONE',  ( 58.72200624034179839, -1.310319377726872903, -1.341335979947030799 ) ) ;
#20142=AXIS2_PLACEMENT_3D ( 'NONE', #2393, #12338, #22186 ) ;
#20144=ORIENTED_EDGE ( 'NONE', *, *, #12487, .F. ) ;
#20149=FACE_OUTER_BOUND ( 'NONE', #996, .T. ) ;
#20150=FACE_OUTER_BOUND ( 'NONE', #24821, .T. ) ;
#20153=FACE_OUTER_BOUND ( 'NONE', #14186, .T. ) ;
#20157=CARTESIAN_POINT ( 'NONE',  ( 58.75000000000000711, 1.655311165517640459, -1.077297519404308179 ) ) ;
#20166=DIRECTION ( 'NONE',  ( 1.000000000000000000, 1.047444401652940007E-14, 0.000000000000000000 ) ) ;
#20174=EDGE_LOOP ( 'NONE', ( #2840, #8507, #9059, #28994, #6570, #12276 ) ) ;
#20175=( NAMED_UNIT ( * ) SI_UNIT ( $, .STERADIAN. ) SOLID_ANGLE_UNIT ( ) );
#20177=B_SPLINE_CURVE_WITH_KNOTS ( 'NONE', 3,
 ( #18690, #9513, #23593, #28813 ),
 .UNSPECIFIED., .F., .F.,
 ( 4, 4 ),
 ( 3.909146525865938448E-19, 0.0001543670095910078732 ),
 .UNSPECIFIED. ) ;
#20188=( BOUNDED_SURFACE ( )  B_SPLINE_SURFACE ( 3, 2, ( 
 ( #31050, #181, #9837 ),
 ( #19507, #29153, #17138 ),
 ( #23635, #24400, #12812 ),
 ( #19965, #10005, #29600 ),
 ( #24709, #29925, #22495 ),
 ( #5556, #20141, #22671 ),
 ( #20295, #7923, #10460 ),
 ( #29770, #8235, #17279 ),
 ( #5391, #22201, #12663 ),
 ( #17596, #22344, #5088 ) ),
 .UNSPECIFIED., .F., .F., .F. ) 
 B_SPLINE_SURFACE_WITH_KNOTS ( ( 4, 2, 2, 2, 4 ),
 ( 3, 3 ),
 ( 0.0001706658715698512231, 0.0002229276920781348066, 0.0002751895125864183629, 0.0003274513330947019193, 0.0003797131536029854757 ),
 ( 0.000000000000000000, 1.000000000000000000 ),
 .UNSPECIFIED. ) 
 GEOMETRIC_REPRESENTATION_ITEM ( )  RATIONAL_B_SPLINE_SURFACE ( (
 ( 1.000000000000000000, 0.7071067811873473774, 1.000000000000000000),
 ( 1.000000000000000000, 0.7375607040707745643, 1.000000000000000000),
 ( 1.000000000000000000, 0.7730431127434318483, 1.000000000000000000),
 ( 1.000000000000000000, 0.8321012486982067857, 1.000000000000000000),
 ( 1.000000000000000000, 0.8541932017400749588, 1.000000000000000000),
 ( 1.000000000000000000, 0.8545723906049677021, 1.000000000000000000),
 ( 1.000000000000000000, 0.8327032135039394989, 1.000000000000000000),
 ( 1.000000000000000000, 0.7734559727058835099, 1.000000000000000000),
 ( 1.000000000000000000, 0.7377766653993951262, 1.000000000000000000),
 ( 1.000000000000000000, 0.7071067811865511255, 1.000000000000000000) ) ) 
 REPRESENTATION_ITEM ( '' )  SURFACE ( )  );
#20190=CARTESIAN_POINT ( 'NONE',  ( 60.82068433953624265, 0.6500001811784626993, 1.489337021788162296 ) ) ;
#20191=CARTESIAN_POINT ( 'NONE',  ( 50.25000000000002842, -0.5380862305914007049, 2.008165151418990213 ) ) ;
#20193=DIRECTION ( 'NONE',  ( 0.000000000000000000, 0.000000000000000000, 1.000000000000000000 ) ) ;
#20199=CARTESIAN_POINT ( 'NONE',  ( 58.75000000000000711, 1.253243060178337753, -1.394635017528379040 ) ) ;
#20216=VERTEX_POINT ( 'NONE', #4784 ) ;
#20221=CARTESIAN_POINT ( 'NONE',  ( 58.65000000000003411, -1.253243060177392953, -1.394635017528123910 ) ) ;
#20222=EDGE_CURVE ( 'NONE', #1083, #23320, #4810, .T. ) ;
#20230=CARTESIAN_POINT ( 'NONE',  ( 58.75000000000000711, 1.666164585743217463, -1.106298139389324975 ) ) ;
#20235=CARTESIAN_POINT ( 'NONE',  ( 51.44193764627956256, -0.9752197701239264660, 1.304631266258929889 ) ) ;
#20237=DIRECTION ( 'NONE',  ( 1.000000000000000000, 1.047444401652940007E-14, 0.000000000000000000 ) ) ;
#20246=CARTESIAN_POINT ( 'NONE',  ( 61.25000000000000711, 1.666164585742400117, 1.106298139391003632 ) ) ;
#20248=ORIENTED_EDGE ( 'NONE', *, *, #29535, .T. ) ;
#20249=CARTESIAN_POINT ( 'NONE',  ( 51.59739104186229497, -1.165722629540969058, -1.468576096419531574 ) ) ;
#20273=CARTESIAN_POINT ( 'NONE',  ( 58.74999999999981526, -1.872332544500615370, 0.09997921184705542419 ) ) ;
#20276=VERTEX_POINT ( 'NONE', #5106 ) ;
#20283=EDGE_CURVE ( 'NONE', #28852, #22920, #29177, .T. ) ;
#20284=VERTEX_POINT ( 'NONE', #7494 ) ;
#20295=CARTESIAN_POINT ( 'NONE',  ( 58.75000018803720536, -1.333992738916506271, -1.403930843796631578 ) ) ;
#20312=DIRECTION ( 'NONE',  ( 1.000000000000000000, 1.047444401652940007E-14, 0.000000000000000000 ) ) ;
#20316=CARTESIAN_POINT ( 'NONE',  ( 51.25000000000002842, -0.9938153758920951208, -1.589954715908409977 ) ) ;
#20317=CARTESIAN_POINT ( 'NONE',  ( 58.66107449606974455, -0.9081280691412084716, -1.640741681270376340 ) ) ;
#20319=EDGE_CURVE ( 'NONE', #7544, #21318, #29114, .T. ) ;
#20328=DIRECTION ( 'NONE',  ( 9.329605248950888974E-15, -1.000000000000000000, 0.000000000000000000 ) ) ;
#20330=SURFACE_STYLE_FILL_AREA ( #29642 ) ;
#20336=CARTESIAN_POINT ( 'NONE',  ( 58.75000000000000711, 1.106298139389943147, 1.666164585743605375 ) ) ;
#20337=EDGE_CURVE ( 'NONE', #2793, #17885, #3321, .T. ) ;
#20339=ORIENTED_EDGE ( 'NONE', *, *, #30815, .T. ) ;
#20342=DIRECTION ( 'NONE',  ( 1.000000000000000000, 1.047444401652940007E-14, 0.000000000000000000 ) ) ;
#20343=LINE ( 'NONE', #29969, #12724 ) ;
#20348=CARTESIAN_POINT ( 'NONE',  ( 51.41935677334221566, 0.9814903265946437472, 1.432156770616830554 ) ) ;
#20351=CARTESIAN_POINT ( 'NONE',  ( 58.74160516400052501, 1.258299259017965355, -1.390091577294809699 ) ) ;
#20356=DIRECTION ( 'NONE',  ( 0.000000000000000000, 0.000000000000000000, 1.000000000000000000 ) ) ;
#20367=ORIENTED_EDGE ( 'NONE', *, *, #3426, .T. ) ;
#20382=CARTESIAN_POINT ( 'NONE',  ( 58.75000000000002132, -0.4991259882252805924, 1.863313159666098562 ) ) ;
#20388=VECTOR ( 'NONE', #15745, 1000.000000000000000 ) ;
#20390=CARTESIAN_POINT ( 'NONE',  ( 50.55256015243839585, -0.05146993878536944289, 0.7900664826958423426 ) ) ;
#20392=VERTEX_POINT ( 'NONE', #19984 ) ;
#20393=EDGE_CURVE ( 'NONE', #24580, #7153, #22983, .T. ) ;
#20394=CARTESIAN_POINT ( 'NONE',  ( 51.12687253673779253, 0.9194130538826112975, -1.491219977510798378 ) ) ;
#20396=FACE_OUTER_BOUND ( 'NONE', #29907, .T. ) ;
#20397=FACE_OUTER_BOUND ( 'NONE', #2085, .T. ) ;
#20398=CARTESIAN_POINT ( 'NONE',  ( 60.75000000000003553, -0.4999999999993604560, 1.718465885608478239 ) ) ;
#20403=ORIENTED_EDGE ( 'NONE', *, *, #4535, .T. ) ;
#20409=CARTESIAN_POINT ( 'NONE',  ( 58.74160516400047527, 1.575205926126477696, -1.017053542743697303 ) ) ;
#20412=DIRECTION ( 'NONE',  ( 0.000000000000000000, -1.000000000000000000, 0.000000000000000000 ) ) ;
#20416=ORIENTED_EDGE ( 'NONE', *, *, #26582, .F. ) ;
#20418=ADVANCED_FACE ( 'NONE', ( #22840 ), #19495, .F. ) ;
#20423=CARTESIAN_POINT ( 'NONE',  ( 58.74999981404336324, -1.953940384111413575, 0.08513245267583949283 ) ) ;
#20428=EDGE_LOOP ( 'NONE', ( #10678, #20780, #12877 ) ) ;
#20434=VERTEX_POINT ( 'NONE', #18866 ) ;
#20443=EDGE_CURVE ( 'NONE', #31166, #4296, #23448, .T. ) ;
#20449=DIRECTION ( 'NONE',  ( 1.000000000000000000, 1.047444401652940007E-14, 0.000000000000000000 ) ) ;
#20450=VECTOR ( 'NONE', #16923, 1000.000000000000000 ) ;
#20452=EDGE_CURVE ( 'NONE', #7041, #30150, #27882, .T. ) ;
#20454=CARTESIAN_POINT ( 'NONE',  ( 58.65263613458537151, -1.827305695290488030, -0.4205413283053403006 ) ) ;
#20455=AXIS2_PLACEMENT_3D ( 'NONE', #20731, #24973, #15799 ) ;
#20456=CIRCLE ( 'NONE', #13344, 0.1500000000000000777 ) ;
#20457=DIRECTION ( 'NONE',  ( -1.387778780781445676E-14, 1.000000000000000000, 0.000000000000000000 ) ) ;
#20462=ADVANCED_FACE ( 'NONE', ( #9039 ), #16169, .T. ) ;
#20463=DIRECTION ( 'NONE',  ( 1.000000000000000000, 1.047444401652940007E-14, 0.000000000000000000 ) ) ;
#20475=AXIS2_PLACEMENT_3D ( 'NONE', #11978, #21665, #16585 ) ;
#20479=CARTESIAN_POINT ( 'NONE',  ( 51.49472959044964426, 1.070956530528826889, -1.224612562803248483 ) ) ;
#20483=VERTEX_POINT ( 'NONE', #9206 ) ;
#20485=ORIENTED_EDGE ( 'NONE', *, *, #23340, .F. ) ;
#20488=CARTESIAN_POINT ( 'NONE',  ( 61.00000000000001421, 0.8666666666673057406, 1.374595900215364930 ) ) ;
#20492=EDGE_CURVE ( 'NONE', #11981, #22245, #16347, .T. ) ;
#20493=AXIS2_PLACEMENT_3D ( 'NONE', #15623, #3584, #22904 ) ;
#20495=EDGE_CURVE ( 'NONE', #22739, #6559, #26960, .T. ) ;
#20502=CARTESIAN_POINT ( 'NONE',  ( 58.65000038048046349, 1.265626441015807568, -1.383507098107855438 ) ) ;
#20508=CARTESIAN_POINT ( 'NONE',  ( 58.66107449606931823, -0.9668599424569509493, 1.606832818401507490 ) ) ;
#20524=DIRECTION ( 'NONE',  ( 0.000000000000000000, 0.000000000000000000, 1.000000000000000000 ) ) ;
#20530=EDGE_CURVE ( 'NONE', #28052, #21195, #13037, .T. ) ;
#20532=EDGE_CURVE ( 'NONE', #1037, #28412, #14230, .T. ) ;
#20537=CARTESIAN_POINT ( 'NONE',  ( 51.14630318392407560, -0.9364487020629673752, -1.503522130792586564 ) ) ;
#20542=CARTESIAN_POINT ( 'NONE',  ( 51.40674769956039114, -0.9873535814794003329, 1.422142864483648461 ) ) ;
#20546=AXIS2_PLACEMENT_3D ( 'NONE', #1943, #11754, #11436 ) ;
#20550=( BOUNDED_SURFACE ( )  B_SPLINE_SURFACE ( 3, 2, ( 
 ( #24651, #270, #2964 ),
 ( #7855, #29540, #2657 ),
 ( #7565, #17225, #12609 ),
 ( #15147, #5805, #23485 ),
 ( #10708, #9245, #28397 ),
 ( #22605, #30013, #6551 ),
 ( #11616, #13656, #30771 ),
 ( #24947, #13965, #25860 ) ),
 .UNSPECIFIED., .F., .F., .F. ) 
 B_SPLINE_SURFACE_WITH_KNOTS ( ( 4, 2, 2, 4 ),
 ( 3, 3 ),
 ( 0.001762834131042892915, 0.001945267826973966826, 0.002127701522905040520, 0.002492568914767187907 ),
 ( 0.000000000000000000, 1.000000000000000000 ),
 .UNSPECIFIED. ) 
 GEOMETRIC_REPRESENTATION_ITEM ( )  RATIONAL_B_SPLINE_SURFACE ( (
 ( 1.000000000000000000, 0.8699658093904940603, 1.000000000000000000),
 ( 1.000000000000000000, 0.8851796357839156748, 1.000000000000000000),
 ( 1.000000000000000000, 0.8977447492167196508, 1.000000000000000000),
 ( 1.000000000000000000, 0.9127836411835481556, 1.000000000000000000),
 ( 1.000000000000000000, 0.9151168517135812586, 1.000000000000000000),
 ( 1.000000000000000000, 0.9045976586032163924, 1.000000000000000000),
 ( 1.000000000000000000, 0.8745315534097299892, 1.000000000000000000),
 ( 1.000000000000000000, 0.8388746406931726352, 1.000000000000000000) ) ) 
 REPRESENTATION_ITEM ( '' )  SURFACE ( )  );
#20555=CARTESIAN_POINT ( 'NONE',  ( 58.75000000000000711, 1.960427193528545109, 0.3958853607757182314 ) ) ;
#20556=ORIENTED_EDGE ( 'NONE', *, *, #28959, .F. ) ;
#20569=AXIS2_PLACEMENT_3D ( 'NONE', #28064, #10983, #858 ) ;
#20574=CIRCLE ( 'NONE', #27125, 2.000000000000000000 ) ;
#20584=CARTESIAN_POINT ( 'NONE',  ( 58.73371041428939066, -1.873417296527896792, -0.08026432063101406056 ) ) ;
#20587=EDGE_CURVE ( 'NONE', #24526, #585, #19342, .T. ) ;
#20588=CARTESIAN_POINT ( 'NONE',  ( 58.73371041428912775, 1.582294810367057547, 1.006219588949640364 ) ) ;
#20596=ORIENTED_EDGE ( 'NONE', *, *, #8315, .T. ) ;
#20608=ORIENTED_EDGE ( 'NONE', *, *, #22984, .T. ) ;
#20614=CARTESIAN_POINT ( 'NONE',  ( 58.75000000000003553, -1.996089927834302724, 0.1250000000000018041 ) ) ;
#20633=DIRECTION ( 'NONE',  ( 0.000000000000000000, 0.000000000000000000, 1.000000000000000000 ) ) ;
#20638=ADVANCED_FACE ( 'NONE', ( #4742 ), #18696, .F. ) ;
#20645=AXIS2_PLACEMENT_3D ( 'NONE', #10368, #6102, #22273 ) ;
#20647=ORIENTED_EDGE ( 'NONE', *, *, #3003, .T. ) ;
#20650=EDGE_CURVE ( 'NONE', #27496, #20928, #2532, .T. ) ;
#20654=CARTESIAN_POINT ( 'NONE',  ( 58.64999999999999858, 1.656030381686821151, 0.8799718970829721876 ) ) ;
#20655=PLANE ( 'NONE',  #7397 ) ;
#20660=CYLINDRICAL_SURFACE ( 'NONE', #25000, 1.625000000000000222 ) ;
#20662=CARTESIAN_POINT ( 'NONE',  ( 50.93312545610842790, 0.6352506689595308620, 1.438808137080896055 ) ) ;
#20663=FACE_OUTER_BOUND ( 'NONE', #19390, .T. ) ;
#20664=CARTESIAN_POINT ( 'NONE',  ( 58.73379417893117704, -1.662624490946059241, -0.8670685180647094148 ) ) ;
#20671=ORIENTED_EDGE ( 'NONE', *, *, #11865, .F. ) ;
#20686=ADVANCED_FACE ( 'NONE', ( #10601 ), #3154, .F. ) ;
#20687=CARTESIAN_POINT ( 'NONE',  ( 61.25000000000002132, 6.415596960124259844E-13, 3.111507638930570854E-58 ) ) ;
#20693=CARTESIAN_POINT ( 'NONE',  ( 51.32247534403771994, -1.004558583830394314, 1.391720660572748791 ) ) ;
#20696=CARTESIAN_POINT ( 'NONE',  ( 58.72427158855725793, 1.357477749119627264, 1.293556822995691302 ) ) ;
#20697=CARTESIAN_POINT ( 'NONE',  ( 51.59739104186227365, 1.010292945603182169, 1.272765950230260401 ) ) ;
#20711=CIRCLE ( 'NONE', #986, 0.1000000000000000472 ) ;
#20716=ORIENTED_EDGE ( 'NONE', *, *, #10120, .F. ) ;
#20731=CARTESIAN_POINT ( 'NONE',  ( 61.25000000000001421, 1.039502773796357360, 1.800471618825331355 ) ) ;
#20738=LINE ( 'NONE', #30848, #7961 ) ;
#20743=ORIENTED_EDGE ( 'NONE', *, *, #15872, .T. ) ;
#20749=VERTEX_POINT ( 'NONE', #22180 ) ;
#20762=B_SPLINE_CURVE_WITH_KNOTS ( 'NONE', 3,
 ( #1397, #23731, #13400, #2023 ),
 .UNSPECIFIED., .F., .F.,
 ( 4, 4 ),
 ( 0.000000000000000000, 0.0003111614939246246819 ),
 .UNSPECIFIED. ) ;
#20769=CARTESIAN_POINT ( 'NONE',  ( 61.25000000000004263, -1.470078920827180724, -1.470078920827526892 ) ) ;
#20770=CARTESIAN_POINT ( 'NONE',  ( 58.75000000000000000, 2.079005547593415937, 1.004182178118534636E-12 ) ) ;
#20775=VERTEX_POINT ( 'NONE', #27695 ) ;
#20777=DIRECTION ( 'NONE',  ( 2.461451434200951079E-12, 0.4531102586349436967, -0.8914544820234930889 ) ) ;
#20780=ORIENTED_EDGE ( 'NONE', *, *, #8075, .T. ) ;
#20786=ORIENTED_EDGE ( 'NONE', *, *, #23921, .T. ) ;
#20787=CARTESIAN_POINT ( 'NONE',  ( 58.75000000000003553, -1.960427193528316847, -0.3958853607747112036 ) ) ;
#20795=CARTESIAN_POINT ( 'NONE',  ( 58.65000000000001990, 6.143261415694495821E-13, 3.111507638930570854E-58 ) ) ;
#20797=ORIENTED_EDGE ( 'NONE', *, *, #28892, .T. ) ;
#20799=CARTESIAN_POINT ( 'NONE',  ( 58.66107449606971613, 1.606832818401695340, 0.9668599424582843271 ) ) ;
#20802=CARTESIAN_POINT ( 'NONE',  ( 58.75000000000002132, 6.153735859711025284E-13, 3.111507638930570854E-58 ) ) ;
#20807=CARTESIAN_POINT ( 'NONE',  ( 58.72200624034172023, -1.612834625124900834, -0.9564954546388050316 ) ) ;
#20812=CARTESIAN_POINT ( 'NONE',  ( 58.75000000000000711, 1.077297519405726156, -1.655311165516502925 ) ) ;
#20813=EDGE_CURVE ( 'NONE', #4204, #25278, #27978, .T. ) ;
#20823=ORIENTED_EDGE ( 'NONE', *, *, #19699, .F. ) ;
#20824=FACE_OUTER_BOUND ( 'NONE', #27023, .T. ) ;
#20829=LINE ( 'NONE', #18156, #13145 ) ;
#20832=ADVANCED_FACE ( 'NONE', ( #7901 ), #275, .F. ) ;
#20838=AXIS2_PLACEMENT_3D ( 'NONE', #25730, #5132, #22093 ) ;
#20841=DIRECTION ( 'NONE',  ( 0.000000000000000000, 0.000000000000000000, 1.000000000000000000 ) ) ;
#20846=CARTESIAN_POINT ( 'NONE',  ( 58.66133336607601478, 1.348863877412731505, 1.302803168108652931 ) ) ;
#20847=CARTESIAN_POINT ( 'NONE',  ( 51.25000000000002842, -0.9938153758920951208, 1.589954715908409977 ) ) ;
#20849=CARTESIAN_POINT ( 'NONE',  ( 51.25000000000001421, 5.368159983410797313E-13, 3.111507638930570854E-58 ) ) ;
#20850=ORIENTED_EDGE ( 'NONE', *, *, #3019, .T. ) ;
#20851=EDGE_LOOP ( 'NONE', ( #24964, #27281, #5856, #28042, #28773, #2483 ) ) ;
#20865=ORIENTED_EDGE ( 'NONE', *, *, #30363, .F. ) ;
#20871=CARTESIAN_POINT ( 'NONE',  ( 58.72419296898058860, 1.822284191843672074, -0.4419487341008165315 ) ) ;
#20875=CARTESIAN_POINT ( 'NONE',  ( 60.94140446606686368, -0.5380862305903196807, -1.858165151418244010 ) ) ;
#20885=ORIENTED_EDGE ( 'NONE', *, *, #28637, .F. ) ;
#20886=CARTESIAN_POINT ( 'NONE',  ( 58.75000018595668649, 1.701752411747378568, 0.9248597378506533406 ) ) ;
#20890=CARTESIAN_POINT ( 'NONE',  ( 58.65000045311413857, -1.383426348886330537, 1.265716300432485841 ) ) ;
#20892=ORIENTED_EDGE ( 'NONE', *, *, #13911, .F. ) ;
#20893=CARTESIAN_POINT ( 'NONE',  ( 50.25000000000002842, -0.5380862305904318132, -2.008165151418244143 ) ) ;
#20899=AXIS2_PLACEMENT_3D ( 'NONE', #917, #10570, #24659 ) ;
#20903=CARTESIAN_POINT ( 'NONE',  ( 52.06628335902944826, 0.5434431642986583544, -1.718465885608440269 ) ) ;
#20907=( BOUNDED_CURVE ( )  B_SPLINE_CURVE ( 3, ( #7324, #26799, #16995, #10162 ),
 .UNSPECIFIED., .F., .T. ) 
 B_SPLINE_CURVE_WITH_KNOTS ( ( 4, 4 ),
 ( 5.439460278842601859, 5.455963239578337287 ),
 .UNSPECIFIED. ) 
 CURVE ( )  GEOMETRIC_REPRESENTATION_ITEM ( )  RATIONAL_B_SPLINE_CURVE ( ( 1.000000000000000000, 0.9999773044860189586, 0.9999773044860189586, 1.000000000000000000 ) ) 
 REPRESENTATION_ITEM ( '' )  );
#20909=CARTESIAN_POINT ( 'NONE',  ( 51.25000000000001421, 0.9938153758931693726, 1.589954715908409755 ) ) ;
#20910=DIRECTION ( 'NONE',  ( 1.000000000000000000, 1.047444401652940007E-14, -0.000000000000000000 ) ) ;
#20915=CARTESIAN_POINT ( 'NONE',  ( 58.65266784251149801, -1.792820108339197027, -0.5492726012740126729 ) ) ;
#20921=CARTESIAN_POINT ( 'NONE',  ( 60.87997700083089114, -0.6727827007652724678, 1.479885446458161669 ) ) ;
#20922=ORIENTED_EDGE ( 'NONE', *, *, #5161, .T. ) ;
#20923=CARTESIAN_POINT ( 'NONE',  ( 51.25000000000001421, 5.368152558471320595E-13, 1.875000000000001776 ) ) ;
#20924=CARTESIAN_POINT ( 'NONE',  ( 58.75000000000002842, -1.039502773796089796, -1.650471618824325359 ) ) ;
#20928=VERTEX_POINT ( 'NONE', #14687 ) ;
#20934=CARTESIAN_POINT ( 'NONE',  ( 58.75000000000000000, 2.079005547593415937, 1.004182178118534636E-12 ) ) ;
#20944=VECTOR ( 'NONE', #18561, 1000.000000000000000 ) ;
#20950=AXIS2_PLACEMENT_3D ( 'NONE', #12449, #17224, #28629 ) ;
#20953=DIRECTION ( 'NONE',  ( 0.000000000000000000, 0.000000000000000000, 1.000000000000000000 ) ) ;
#20963=CARTESIAN_POINT ( 'NONE',  ( 61.25000000000002132, 6.415596960124259844E-13, 3.111507638930570854E-58 ) ) ;
#20966=ORIENTED_EDGE ( 'NONE', *, *, #3445, .T. ) ;
#20967=CARTESIAN_POINT ( 'NONE',  ( 51.29331479884403677, 1.002608958138274442, 1.584424273060084376 ) ) ;
#20968=CIRCLE ( 'NONE', #18438, 0.1000000000000000333 ) ;
#20972=ORIENTED_EDGE ( 'NONE', *, *, #24547, .F. ) ;
#20974=ORIENTED_EDGE ( 'NONE', *, *, #18853, .T. ) ;
#20975=CARTESIAN_POINT ( 'NONE',  ( 51.11922224408084503, 0.9310536428531384079, -1.338077479438677830 ) ) ;
#20980=AXIS2_PLACEMENT_3D ( 'NONE', #6094, #15744, #25394 ) ;
#20984=ORIENTED_EDGE ( 'NONE', *, *, #23356, .F. ) ;
#20990=CARTESIAN_POINT ( 'NONE',  ( 51.25000000000001421, 1.100000000000537215, -1.996089927833914146 ) ) ;
#20991=CARTESIAN_POINT ( 'NONE',  ( 58.74160516400055343, 1.390091577294495062, 1.258299259018362815 ) ) ;
#21000=DIRECTION ( 'NONE',  ( 0.000000000000000000, 0.000000000000000000, 1.000000000000000000 ) ) ;
#21002=ORIENTED_EDGE ( 'NONE', *, *, #18313, .T. ) ;
#21008=EDGE_LOOP ( 'NONE', ( #7785, #30276, #22440, #15437, #24139, #25 ) ) ;
#21019=EDGE_LOOP ( 'NONE', ( #22235, #9716, #12072, #25826 ) ) ;
#21037=EDGE_CURVE ( 'NONE', #31243, #15189, #18890, .T. ) ;
#21041=AXIS2_PLACEMENT_3D ( 'NONE', #17837, #27471, #25097 ) ;
#21051=CARTESIAN_POINT ( 'NONE',  ( 58.65263613458531466, 1.656197658589030342, 0.8791532451981106666 ) ) ;
#21052=ORIENTED_EDGE ( 'NONE', *, *, #8987, .T. ) ;
#21054=CARTESIAN_POINT ( 'NONE',  ( 58.66118217212467556, -1.313877211063203987, 1.337770226785896854 ) ) ;
#21065=ADVANCED_FACE ( 'NONE', ( #5808 ), #26870, .F. ) ;
#21078=ADVANCED_FACE ( 'NONE', ( #1061 ), #22441, .F. ) ;
#21086=DIRECTION ( 'NONE',  ( 0.000000000000000000, 0.000000000000000000, 1.000000000000000000 ) ) ;
#21087=CARTESIAN_POINT ( 'NONE',  ( 58.75000000000004263, -1.782657835994226003, -0.5811678240974800236 ) ) ;
#21094=CARTESIAN_POINT ( 'NONE',  ( 60.88446240048057945, -0.4999999999993621769, -1.718465885608439603 ) ) ;
#21095=AXIS2_PLACEMENT_3D ( 'NONE', #1767, #19828, #12362 ) ;
#21110=CARTESIAN_POINT ( 'NONE',  ( 58.64999999999999147, 1.872332544501833507, -0.09997921184724641031 ) ) ;
#21111=EDGE_LOOP ( 'NONE', ( #18328, #798, #698, #5767, #28509, #16221 ) ) ;
#21116=CIRCLE ( 'NONE', #3912, 2.000000000000000000 ) ;
#21127=CARTESIAN_POINT ( 'NONE',  ( 51.59739104186229497, -1.010292945602101256, -1.272765950230260623 ) ) ;
#21136=CARTESIAN_POINT ( 'NONE',  ( 50.56948141424500420, -0.1019060742254479235, 1.190674082256532262 ) ) ;
#21137=CARTESIAN_POINT ( 'NONE',  ( 60.99772080470438596, -0.5608984830164329694, 1.857935446186627093 ) ) ;
#21148=VERTEX_POINT ( 'NONE', #12612 ) ;
#21150=ORIENTED_EDGE ( 'NONE', *, *, #23059, .T. ) ;
#21152=CARTESIAN_POINT ( 'NONE',  ( 58.65000045311390409, -1.663878723406634785, 0.8645309767543464252 ) ) ;
#21155=DIRECTION ( 'NONE',  ( 0.000000000000000000, 0.000000000000000000, 1.000000000000000000 ) ) ;
#21156=CARTESIAN_POINT ( 'NONE',  ( 52.20711756518983293, 0.5000000000005468959, 1.807104036850122109 ) ) ;
#21159=VERTEX_POINT ( 'NONE', #20394 ) ;
#21162=CIRCLE ( 'NONE', #5455, 1.487500000000000933 ) ;
#21170=EDGE_CURVE ( 'NONE', #10512, #24580, #31028, .T. ) ;
#21171=DIRECTION ( 'NONE',  ( 0.000000000000000000, 0.8914544820233750722, 0.4531102586351760109 ) ) ;
#21172=CARTESIAN_POINT ( 'NONE',  ( 58.75000000000002132, -0.6121634413826990695, 1.877732920581024700 ) ) ;
#21173=CARTESIAN_POINT ( 'NONE',  ( 58.72200907981793705, -0.5299537992501781591, -1.799145225589202424 ) ) ;
#21181=CIRCLE ( 'NONE', #26218, 1.875000000000001776 ) ;
#21184=ORIENTED_EDGE ( 'NONE', *, *, #6438, .F. ) ;
#21195=VERTEX_POINT ( 'NONE', #11179 ) ;
#21200=CARTESIAN_POINT ( 'NONE',  ( 58.75000000000000000, 1.932246131438033254, -0.4087173687832941216 ) ) ;
#21202=CARTESIAN_POINT ( 'NONE',  ( 50.25000000000001421, 0.5380862305914526633, -1.858165151417984218 ) ) ;
#21204=B_SPLINE_CURVE_WITH_KNOTS ( 'NONE', 3,
 ( #26512, #30629, #28270, #13830, #4520, #11801 ),
 .UNSPECIFIED., .F., .F.,
 ( 4, 2, 4 ),
 ( 0.000000000000000000, 0.0001000270069601567446, 0.0002000540139203134892 ),
 .UNSPECIFIED. ) ;
#21208=EDGE_CURVE ( 'NONE', #28852, #624, #25964, .T. ) ;
#21214=CARTESIAN_POINT ( 'NONE',  ( 58.65000000000001990, 6.143261415694495821E-13, 3.111507638930570854E-58 ) ) ;
#21222=CARTESIAN_POINT ( 'NONE',  ( 58.75000000694006275, 0.9860766835998435731, -1.658042653847561887 ) ) ;
#21223=CARTESIAN_POINT ( 'NONE',  ( 58.72427158855744267, -1.293556822995290512, 1.357477749118862542 ) ) ;
#21227=EDGE_CURVE ( 'NONE', #7031, #19651, #13314, .T. ) ;
#21230=CARTESIAN_POINT ( 'NONE',  ( 58.75000000000000711, 0.8980135333485337323, 1.749295403805501525 ) ) ;
#21231=ADVANCED_FACE ( 'NONE', ( #4055 ), #6439, .T. ) ;
#21232=ORIENTED_EDGE ( 'NONE', *, *, #25559, .T. ) ;
#21236=DIRECTION ( 'NONE',  ( 1.000000000000000000, 1.047444401652940007E-14, 0.000000000000000000 ) ) ;
#21245=CARTESIAN_POINT ( 'NONE',  ( 58.75000000000002132, -0.6373668173473671095, 1.895722432253304168 ) ) ;
#21248=CIRCLE ( 'NONE', #25781, 0.1500000000000001887 ) ;
#21252=EDGE_CURVE ( 'NONE', #28206, #24348, #5142, .T. ) ;
#21264=ORIENTED_EDGE ( 'NONE', *, *, #7852, .F. ) ;
#21270=EDGE_CURVE ( 'NONE', #10008, #4687, #212, .T. ) ;
#21271=FACE_OUTER_BOUND ( 'NONE', #5627, .T. ) ;
#21274=CARTESIAN_POINT ( 'NONE',  ( 58.73379417893114152, 1.873409305146914283, -0.08040888200754815751 ) ) ;
#21278=ORIENTED_EDGE ( 'NONE', *, *, #20319, .T. ) ;
#21286=CARTESIAN_POINT ( 'NONE',  ( 58.75000000000002132, 6.153735859711025284E-13, 3.111507638930570854E-58 ) ) ;
#21294=CARTESIAN_POINT ( 'NONE',  ( 58.74160516400029763, -1.668397168087478510, -0.8556415768453068393 ) ) ;
#21299=CARTESIAN_POINT ( 'NONE',  ( 50.59602332238209499, -0.1408342061598474859, 0.8215393206232036727 ) ) ;
#21303=B_SPLINE_CURVE_WITH_KNOTS ( 'NONE', 3,
 ( #5113, #24571, #10491, #5730, #5423, #15381 ),
 .UNSPECIFIED., .F., .F.,
 ( 4, 2, 4 ),
 ( 0.000000000000000000, 0.0003974125641964876884, 0.0007948251283929753767 ),
 .UNSPECIFIED. ) ;
#21305=CARTESIAN_POINT ( 'NONE',  ( 58.75000000000002132, -0.5380862305903428844, -2.008165151418244143 ) ) ;
#21306=CARTESIAN_POINT ( 'NONE',  ( 60.82166330297963697, 0.6500000603371848262, -1.489337074527656180 ) ) ;
#21309=ORIENTED_EDGE ( 'NONE', *, *, #24815, .F. ) ;
#21312=CARTESIAN_POINT ( 'NONE',  ( 58.65263613458529335, -1.589467873454749158, 0.9947326234267183098 ) ) ;
#21316=CARTESIAN_POINT ( 'NONE',  ( 58.66107449606942481, -1.874988011598432092, -0.03390886286852046877 ) ) ;
#21318=VERTEX_POINT ( 'NONE', #21484 ) ;
#21322=DIRECTION ( 'NONE',  ( 5.713464585390589802E-15, -0.5454670984325608041, -0.8381322357048218707 ) ) ;
#21325=DIRECTION ( 'NONE',  ( -0.8262273428075421755, -0.5633368246415177971, 0.000000000000000000 ) ) ;
#21329=CARTESIAN_POINT ( 'NONE',  ( 58.72419296898096519, -0.9760445624805118570, 1.601054456121152381 ) ) ;
#21334=CARTESIAN_POINT ( 'NONE',  ( 61.25000000000002132, 6.415596960124259844E-13, 3.111507638930570854E-58 ) ) ;
#21337=CIRCLE ( 'NONE', #11710, 1.875000000000001776 ) ;
#21339=VERTEX_POINT ( 'NONE', #29797 ) ;
#21342=CYLINDRICAL_SURFACE ( 'NONE', #19600, 0.1499999999999999667 ) ;
#21349=DIRECTION ( 'NONE',  ( 0.000000000000000000, -1.065814103640152803E-14, 1.000000000000000000 ) ) ;
#21351=CARTESIAN_POINT ( 'NONE',  ( 58.66133336607565241, -1.607522887371482856, 0.9657121834149411388 ) ) ;
#21355=CARTESIAN_POINT ( 'NONE',  ( 58.73379417893106336, 1.788763080992656462, -0.5625430232385030260 ) ) ;
#21371=CARTESIAN_POINT ( 'NONE',  ( 51.25000000000001421, 5.365856345722919090E-13, -1.875000000000001776 ) ) ;
#21375=DIRECTION ( 'NONE',  ( 0.5633368246414944824, 0.8262273428075580517, 0.000000000000000000 ) ) ;
#21380=CYLINDRICAL_SURFACE ( 'NONE', #16944, 0.2500000000000000000 ) ;
#21383=CARTESIAN_POINT ( 'NONE',  ( 58.75000000000003553, -1.800471618824212694, -1.039502773796582069 ) ) ;
#21384=CARTESIAN_POINT ( 'NONE',  ( 58.66118217212486030, 0.9521303665439819763, 1.615348343402630560 ) ) ;
#21385=ORIENTED_EDGE ( 'NONE', *, *, #14326, .T. ) ;
#21391=AXIS2_PLACEMENT_3D ( 'NONE', #21334, #28434, #11804 ) ;
#21403=CARTESIAN_POINT ( 'NONE',  ( 50.25000000000001421, 0.5000000000005263567, 1.863080903344386030 ) ) ;
#21405=ORIENTED_EDGE ( 'NONE', *, *, #3546, .T. ) ;
#21406=CARTESIAN_POINT ( 'NONE',  ( 52.13000000000001677, 0.5000000000005460077, 1.718465885608440491 ) ) ;
#21407=AXIS2_PLACEMENT_3D ( 'NONE', #19576, #2297, #2466 ) ;
#21412=ORIENTED_EDGE ( 'NONE', *, *, #31187, .T. ) ;
#21417=DIRECTION ( 'NONE',  ( 1.000000000000000000, 1.047444401652940007E-14, 0.000000000000000000 ) ) ;
#21419=CARTESIAN_POINT ( 'NONE',  ( 58.74999999999999289, 1.872332544501826845, -0.09997921184724604948 ) ) ;
#21432=DIRECTION ( 'NONE',  ( 0.000000000000000000, 0.000000000000000000, 1.000000000000000000 ) ) ;
#21434=EDGE_CURVE ( 'NONE', #27455, #20775, #11252, .T. ) ;
#21439=VERTEX_POINT ( 'NONE', #13618 ) ;
#21442=ORIENTED_EDGE ( 'NONE', *, *, #6157, .T. ) ;
#21458=EDGE_LOOP ( 'NONE', ( #27465, #8752, #23495, #1629, #25359, #3821, #6495 ) ) ;
#21463=ORIENTED_EDGE ( 'NONE', *, *, #29611, .T. ) ;
#21471=CARTESIAN_POINT ( 'NONE',  ( 61.25000000000001421, 0.5000000000006414869, 1.807104036850122109 ) ) ;
#21473=FACE_OUTER_BOUND ( 'NONE', #11543, .T. ) ;
#21481=ORIENTED_EDGE ( 'NONE', *, *, #2115, .F. ) ;
#21483=ORIENTED_EDGE ( 'NONE', *, *, #29061, .F. ) ;
#21484=CARTESIAN_POINT ( 'NONE',  ( 61.00000000000002842, -0.8666666666660278739, 1.374595900215364930 ) ) ;
#21485=ORIENTED_EDGE ( 'NONE', *, *, #18229, .F. ) ;
#21488=DIRECTION ( 'NONE',  ( 0.000000000000000000, 0.000000000000000000, 1.000000000000000000 ) ) ;
#21490=VERTEX_POINT ( 'NONE', #1443 ) ;
#21491=ORIENTED_EDGE ( 'NONE', *, *, #5923, .T. ) ;
#21493=CYLINDRICAL_SURFACE ( 'NONE', #5966, 0.2500000000000000000 ) ;
#21510=AXIS2_PLACEMENT_3D ( 'NONE', #26973, #5457, #5281 ) ;
#21511=DIRECTION ( 'NONE',  ( 0.000000000000000000, 1.000000000000000000, 0.000000000000000000 ) ) ;
#21512=EDGE_CURVE ( 'NONE', #8618, #36, #23784, .T. ) ;
#21534=CARTESIAN_POINT ( 'NONE',  ( 61.23883361641895817, 0.8947175514080812908, 1.757895546655339869 ) ) ;
#21543=CARTESIAN_POINT ( 'NONE',  ( 58.65000000000000568, 1.469015551796266195, 1.320082690054878549 ) ) ;
#21546=AXIS2_PLACEMENT_3D ( 'NONE', #27797, #12785, #8057 ) ;
#21555=CARTESIAN_POINT ( 'NONE',  ( 58.75000000000004263, -1.871930101356778842, -0.6019471833004125250 ) ) ;
#21558=DIRECTION ( 'NONE',  ( -1.000000000000000000, -1.047444401652940007E-14, -0.000000000000000000 ) ) ;
#21562=CARTESIAN_POINT ( 'NONE',  ( 58.74999999305998699, -1.856692759305439644, 0.5240691109004367298 ) ) ;
#21568=VERTEX_POINT ( 'NONE', #11889 ) ;
#21570=CARTESIAN_POINT ( 'NONE',  ( 51.16322424031762495, -0.9520424791877071247, -1.480283991513583697 ) ) ;
#21571=VECTOR ( 'NONE', #27729, 1000.000000000000000 ) ;
#21573=ORIENTED_EDGE ( 'NONE', *, *, #22855, .T. ) ;
#21578=DIRECTION ( 'NONE',  ( 0.000000000000000000, 0.000000000000000000, -1.000000000000000000 ) ) ;
#21581=EDGE_CURVE ( 'NONE', #15271, #29960, #18411, .T. ) ;
#21596=EDGE_CURVE ( 'NONE', #67, #8224, #3524, .T. ) ;
#21597=AXIS2_PLACEMENT_3D ( 'NONE', #11127, #8898, #8736 ) ;
#21604=DIRECTION ( 'NONE',  ( 0.000000000000000000, -0.5333333333333335480, 0.8459051693633012903 ) ) ;
#21607=CARTESIAN_POINT ( 'NONE',  ( 58.65000000000004121, -1.872332544500605378, 0.09997921184723741750 ) ) ;
#21609=EDGE_CURVE ( 'NONE', #17628, #25335, #30425, .T. ) ;
#21611=VECTOR ( 'NONE', #3691, 1000.000000000000000 ) ;
#21618=ORIENTED_EDGE ( 'NONE', *, *, #20650, .F. ) ;
#21622=ORIENTED_EDGE ( 'NONE', *, *, #5161, .F. ) ;
#21630=AXIS2_PLACEMENT_3D ( 'NONE', #26037, #9888, #9431 ) ;
#21632=EDGE_CURVE ( 'NONE', #10205, #1939, #12818, .T. ) ;
#21634=ORIENTED_EDGE ( 'NONE', *, *, #6982, .T. ) ;
#21637=CARTESIAN_POINT ( 'NONE',  ( 58.66122797211853879, -0.9232791089885744595, -1.632010475558218099 ) ) ;
#21638=ORIENTED_EDGE ( 'NONE', *, *, #21632, .F. ) ;
#21641=CARTESIAN_POINT ( 'NONE',  ( 58.75000000000002132, 6.153735859711025284E-13, 3.111507638930570854E-58 ) ) ;
#21642=CIRCLE ( 'NONE', #7959, 0.7375000000000040412 ) ;
#21644=AXIS2_PLACEMENT_3D ( 'NONE', #30367, #30688, #3765 ) ;
#21646=CARTESIAN_POINT ( 'NONE',  ( 58.75000000000002842, -0.8948927608042580584, 1.760622601995711189 ) ) ;
#21647=CARTESIAN_POINT ( 'NONE',  ( 58.71182503183446499, -0.4999999999993852695, 1.820794158166703314 ) ) ;
#21654=EDGE_CURVE ( 'NONE', #21439, #833, #23466, .T. ) ;
#21656=CARTESIAN_POINT ( 'NONE',  ( 58.67990267795825332, 0.5000000000006146195, -1.808383001045529292 ) ) ;
#21664=ORIENTED_EDGE ( 'NONE', *, *, #21654, .T. ) ;
#21665=DIRECTION ( 'NONE',  ( -1.000000000000000000, -1.047444401652940007E-14, -0.000000000000000000 ) ) ;
#21667=ORIENTED_EDGE ( 'NONE', *, *, #10213, .F. ) ;
#21683=DIRECTION ( 'NONE',  ( 0.000000000000000000, 0.000000000000000000, -1.000000000000000000 ) ) ;
#21684=CARTESIAN_POINT ( 'NONE',  ( 58.75000000000003553, -1.499837071477731820, -1.323060376181415254 ) ) ;
#21686=EDGE_CURVE ( 'NONE', #23034, #624, #22470, .T. ) ;
#21688=CARTESIAN_POINT ( 'NONE',  ( 52.06628335902944826, 0.5434431642986584654, 1.794517909405660250 ) ) ;
#21696=CARTESIAN_POINT ( 'NONE',  ( 58.74999999305995857, 0.9423072185563144965, -1.683452862812838235 ) ) ;
#21698=ORIENTED_EDGE ( 'NONE', *, *, #15859, .F. ) ;
#21699=FACE_OUTER_BOUND ( 'NONE', #29325, .T. ) ;
#21701=CARTESIAN_POINT ( 'NONE',  ( 58.74999981404332061, 1.050697058760077685, 1.649595783783794678 ) ) ;
#21706=VECTOR ( 'NONE', #30054, 1000.000000000000000 ) ;
#21713=CARTESIAN_POINT ( 'NONE',  ( 58.64999999999999858, 1.834410884276226117, 0.3880228184671293268 ) ) ;
#21722=CARTESIAN_POINT ( 'NONE',  ( 61.24343480274162488, -0.9192405086477845044, 1.710822371303207579 ) ) ;
#21726=ORIENTED_EDGE ( 'NONE', *, *, #22072, .F. ) ;
#21727=CIRCLE ( 'NONE', #7535, 0.1500000000000001887 ) ;
#21728=CARTESIAN_POINT ( 'NONE',  ( 58.65000045311414567, -1.830940512616420435, 0.4044292957153704515 ) ) ;
#21736=VERTEX_POINT ( 'NONE', #4753 ) ;
#21740=ORIENTED_EDGE ( 'NONE', *, *, #26567, .T. ) ;
#21742=EDGE_LOOP ( 'NONE', ( #20823, #11478, #10409, #20984 ) ) ;
#21755=CARTESIAN_POINT ( 'NONE',  ( 58.65000000000001990, 6.143261415694495821E-13, 3.111507638930570854E-58 ) ) ;
#21761=CARTESIAN_POINT ( 'NONE',  ( 58.65000000000000568, 1.394635017529600507, -1.253243060177047896 ) ) ;
#21765=ORIENTED_EDGE ( 'NONE', *, *, #5015, .F. ) ;
#21772=VERTEX_POINT ( 'NONE', #29590 ) ;
#21773=CARTESIAN_POINT ( 'NONE',  ( 58.65000000000001279, 0.6121634413823858756, 1.877732920581527631 ) ) ;
#21775=CIRCLE ( 'NONE', #8092, 1.875000000000001776 ) ;
#21781=LINE ( 'NONE', #26665, #22514 ) ;
#21798=CARTESIAN_POINT ( 'NONE',  ( 58.75000000000002132, 6.153735859711025284E-13, 3.111507638930570854E-58 ) ) ;
#21800=CARTESIAN_POINT ( 'NONE',  ( 58.65000000000001990, 6.143261415694495821E-13, 3.111507638930570854E-58 ) ) ;
#21804=ORIENTED_EDGE ( 'NONE', *, *, #27633, .F. ) ;
#21807=ORIENTED_EDGE ( 'NONE', *, *, #5209, .F. ) ;
#21808=DIRECTION ( 'NONE',  ( 0.000000000000000000, 0.000000000000000000, -1.000000000000000000 ) ) ;
#21811=CARTESIAN_POINT ( 'NONE',  ( 51.36702623273012591, 1.002608958138273554, -1.584424273060083044 ) ) ;
#21819=CARTESIAN_POINT ( 'NONE',  ( 58.65000000000004121, -1.656314228057949034, 0.8794134543728125974 ) ) ;
#21823=DIRECTION ( 'NONE',  ( 0.000000000000000000, 0.000000000000000000, 1.000000000000000000 ) ) ;
#21824=AXIS2_PLACEMENT_3D ( 'NONE', #19934, #17871, #27363 ) ;
#21825=CARTESIAN_POINT ( 'NONE',  ( 61.25000000000004263, -1.666164585741877424, -1.106298139389857660 ) ) ;
#21827=EDGE_CURVE ( 'NONE', #20276, #2603, #14856, .T. ) ;
#21842=CARTESIAN_POINT ( 'NONE',  ( 58.65000000000001279, 1.278599783849776461, -1.371849028670597104 ) ) ;
#21843=FACE_OUTER_BOUND ( 'NONE', #27901, .T. ) ;
#21865=EDGE_CURVE ( 'NONE', #26557, #18525, #19141, .T. ) ;
#21869=DIRECTION ( 'NONE',  ( 0.000000000000000000, 0.000000000000000000, 1.000000000000000000 ) ) ;
#21875=CARTESIAN_POINT ( 'NONE',  ( 58.75000000000001421, 0.5811678240972331100, 1.782657835995121509 ) ) ;
#21878=CARTESIAN_POINT ( 'NONE',  ( 58.65263613458537151, -1.792763816754253892, 0.5494533739914930770 ) ) ;
#21879=CARTESIAN_POINT ( 'NONE',  ( 60.75000000000001421, 0.6500000000006362910, 1.489337100860648189 ) ) ;
#21885=CARTESIAN_POINT ( 'NONE',  ( 58.75000000000000711, 1.800471618824440734, 1.039502773797588597 ) ) ;
#21894=DIRECTION ( 'NONE',  ( 1.000000000000000000, 1.047444401652940007E-14, 0.000000000000000000 ) ) ;
#21895=ORIENTED_EDGE ( 'NONE', *, *, #21434, .F. ) ;
#21897=B_SPLINE_CURVE_WITH_KNOTS ( 'NONE', 3,
 ( #28514, #6515, #25821, #13615 ),
 .UNSPECIFIED., .F., .F.,
 ( 4, 4 ),
 ( 0.0001521069361438105792, 0.0002184312136277813138 ),
 .UNSPECIFIED. ) ;
#21906=DIRECTION ( 'NONE',  ( -1.047444401652940007E-14, 1.000000000000000000, 0.000000000000000000 ) ) ;
#21911=CARTESIAN_POINT ( 'NONE',  ( 51.78416995154973534, 0.8999235898787814047, 1.360374659026170496 ) ) ;
#21926=EDGE_LOOP ( 'NONE', ( #5268, #28886, #17599, #29030, #14884 ) ) ;
#21927=ORIENTED_EDGE ( 'NONE', *, *, #12856, .T. ) ;
#21937=ORIENTED_EDGE ( 'NONE', *, *, #4031, .T. ) ;
#21938=EDGE_CURVE ( 'NONE', #5594, #21736, #11340, .T. ) ;
#21941=CARTESIAN_POINT ( 'NONE',  ( 58.73379417893105625, -1.006340787081331456, -1.582215608938851270 ) ) ;
#21942=DIRECTION ( 'NONE',  ( 1.000000000000000000, 1.047444401652940007E-14, 0.000000000000000000 ) ) ;
#21946=FACE_OUTER_BOUND ( 'NONE', #1841, .T. ) ;
#21950=CARTESIAN_POINT ( 'NONE',  ( 61.24959995150304337, -0.9774770340128312585, -1.663387054287091882 ) ) ;
#21960=VERTEX_POINT ( 'NONE', #28329 ) ;
#21961=CARTESIAN_POINT ( 'NONE',  ( 51.25000000000001421, 0.7500000000005367928, -1.718465885608440269 ) ) ;
#21962=ORIENTED_EDGE ( 'NONE', *, *, #5984, .T. ) ;
#21968=LINE ( 'NONE', #9152, #6661 ) ;
#21983=VERTEX_POINT ( 'NONE', #16139 ) ;
#21997=CARTESIAN_POINT ( 'NONE',  ( 61.24794577449333133, 0.9523642485468641894, 1.677218681935483069 ) ) ;
#22011=B_SPLINE_CURVE_WITH_KNOTS ( 'NONE', 3,
 ( #30169, #3721, #13537, #8487 ),
 .UNSPECIFIED., .F., .F.,
 ( 4, 4 ),
 ( 8.741117365843378158E-19, 2.862003379457917908E-05 ),
 .UNSPECIFIED. ) ;
#22012=ADVANCED_FACE ( 'NONE', ( #25790 ), #13890, .F. ) ;
#22016=CARTESIAN_POINT ( 'NONE',  ( 51.12687253673779253, 0.9194130538826106314, 1.491219977510798156 ) ) ;
#22018=ORIENTED_EDGE ( 'NONE', *, *, #26519, .T. ) ;
#22023=CARTESIAN_POINT ( 'NONE',  ( 58.66054497608038076, -0.4999999999994944599, -1.807104036850091688 ) ) ;
#22027=AXIS2_PLACEMENT_3D ( 'NONE', #6045, #27551, #5570 ) ;
#22030=FACE_OUTER_BOUND ( 'NONE', #13086, .T. ) ;
#22032=EDGE_CURVE ( 'NONE', #23034, #20928, #6287, .T. ) ;
#22054=CARTESIAN_POINT ( 'NONE',  ( 51.14630318392394770, 0.9364487020639118420, -1.503522130792751987 ) ) ;
#22061=CIRCLE ( 'NONE', #30120, 0.1000000000000001305 ) ;
#22063=DIRECTION ( 'NONE',  ( 1.000000000000000000, 1.047444401652940007E-14, 0.000000000000000000 ) ) ;
#22072=EDGE_CURVE ( 'NONE', #22168, #31257, #5259, .T. ) ;
#22073=CARTESIAN_POINT ( 'NONE',  ( 51.14630318392394770, 0.9364487020639118420, -1.503522130792751987 ) ) ;
#22074=ORIENTED_EDGE ( 'NONE', *, *, #5579, .F. ) ;
#22076=VECTOR ( 'NONE', #27092, 1000.000000000000000 ) ;
#22088=VECTOR ( 'NONE', #17840, 1000.000000000000000 ) ;
#22092=DIRECTION ( 'NONE',  ( 0.5633368246415009217, 0.8262273428075537218, 0.000000000000000000 ) ) ;
#22093=DIRECTION ( 'NONE',  ( 0.000000000000000000, 0.000000000000000000, 1.000000000000000000 ) ) ;
#22100=VECTOR ( 'NONE', #360, 1000.000000000000000 ) ;
#22101=CARTESIAN_POINT ( 'NONE',  ( 51.08379317338046377, 0.8723108729837811826, 1.374656996893403260 ) ) ;
#22102=CARTESIAN_POINT ( 'NONE',  ( 60.75000000000002842, -0.4999999999993638977, -1.863080903343643069 ) ) ;
#22104=CARTESIAN_POINT ( 'NONE',  ( 61.25000000000003553, -0.9999999999993586242, -1.655766640118113031 ) ) ;
#22111=CIRCLE ( 'NONE', #7916, 1.975000000000001865 ) ;
#22117=ORIENTED_EDGE ( 'NONE', *, *, #2364, .F. ) ;
#22119=ORIENTED_EDGE ( 'NONE', *, *, #29522, .F. ) ;
#22140=DIRECTION ( 'NONE',  ( 0.000000000000000000, 0.000000000000000000, 1.000000000000000000 ) ) ;
#22145=EDGE_CURVE ( 'NONE', #24125, #13972, #26566, .T. ) ;
#22153=VERTEX_POINT ( 'NONE', #19458 ) ;
#22154=CARTESIAN_POINT ( 'NONE',  ( 60.97799375661013244, -0.7610968749141068246, -1.436497712332848398 ) ) ;
#22161=CARTESIAN_POINT ( 'NONE',  ( 58.65000000000001990, 6.143261415694495821E-13, 3.111507638930570854E-58 ) ) ;
#22163=ADVANCED_FACE ( 'NONE', ( #24497 ), #9326, .T. ) ;
#22164=CARTESIAN_POINT ( 'NONE',  ( 58.75000000000000711, 1.800471618824440734, 1.039502773797588597 ) ) ;
#22167=CARTESIAN_POINT ( 'NONE',  ( 51.98914612709255323, -0.7788013043298537275, -1.433123603079401231 ) ) ;
#22168=VERTEX_POINT ( 'NONE', #26265 ) ;
#22174=CARTESIAN_POINT ( 'NONE',  ( 51.14630318392396902, -0.9364487020628400327, 1.503522130792752209 ) ) ;
#22176=DIRECTION ( 'NONE',  ( 0.000000000000000000, 0.000000000000000000, 1.000000000000000000 ) ) ;
#22179=EDGE_CURVE ( 'NONE', #26840, #31166, #30411, .T. ) ;
#22180=CARTESIAN_POINT ( 'NONE',  ( 61.25000000000004263, -1.499837071477534867, 1.323060376180833275 ) ) ;
#22181=VERTEX_POINT ( 'NONE', #14836 ) ;
#22186=DIRECTION ( 'NONE',  ( 0.000000000000000000, 0.000000000000000000, 1.000000000000000000 ) ) ;
#22191=DIRECTION ( 'NONE',  ( 1.000000000000000000, 1.047444401652940007E-14, 0.000000000000000000 ) ) ;
#22198=ORIENTED_EDGE ( 'NONE', *, *, #7021, .T. ) ;
#22200=ADVANCED_FACE ( 'NONE', ( #9791 ), #21380, .T. ) ;
#22201=CARTESIAN_POINT ( 'NONE',  ( 58.74154451056421067, -1.258335925859845439, -1.390058629628315057 ) ) ;
#22209=DIRECTION ( 'NONE',  ( 0.000000000000000000, 0.000000000000000000, 1.000000000000000000 ) ) ;
#22213=PRODUCT ( 'Eraser Holder', 'Eraser Holder', '', ( #23281 ) ) ;
#22217=CARTESIAN_POINT ( 'NONE',  ( 58.75000000000002132, 6.153735859711025284E-13, 3.111507638930570854E-58 ) ) ;
#22220=ADVANCED_FACE ( 'NONE', ( #21699 ), #10006, .T. ) ;
#22228=DIRECTION ( 'NONE',  ( 0.000000000000000000, 0.000000000000000000, 1.000000000000000000 ) ) ;
#22229=ORIENTED_EDGE ( 'NONE', *, *, #14630, .F. ) ;
#22233=CARTESIAN_POINT ( 'NONE',  ( 58.65000000000002700, -0.5811678240976775323, -1.782657835994575724 ) ) ;
#22235=ORIENTED_EDGE ( 'NONE', *, *, #6312, .T. ) ;
#22236=SURFACE_SIDE_STYLE ('',( #20330 ) ) ;
#22240=VERTEX_POINT ( 'NONE', #15159 ) ;
#22245=VERTEX_POINT ( 'NONE', #13091 ) ;
#22246=CARTESIAN_POINT ( 'NONE',  ( 51.69060524973921389, 0.7995873297242470645, -1.427997211818276435 ) ) ;
#22247=DIRECTION ( 'NONE',  ( -0.8262273428075537218, 0.5633368246415009217, 0.000000000000000000 ) ) ;
#22248=CARTESIAN_POINT ( 'NONE',  ( 60.81601545282717325, 0.5000000000006243894, -1.863080903339688899 ) ) ;
#22254=CARTESIAN_POINT ( 'NONE',  ( 58.75000000000002842, -1.065927491743560163, 1.652350234724849765 ) ) ;
#22255=CARTESIAN_POINT ( 'NONE',  ( 50.25000000000000711, 1.039502773797110979, -1.650471618823823539 ) ) ;
#22257=AXIS2_PLACEMENT_3D ( 'NONE', #2349, #18515, #28158 ) ;
#22261=VERTEX_POINT ( 'NONE', #15471 ) ;
#22269=ORIENTED_EDGE ( 'NONE', *, *, #23524, .F. ) ;
#22272=ORIENTED_EDGE ( 'NONE', *, *, #25005, .F. ) ;
#22273=DIRECTION ( 'NONE',  ( 0.000000000000000000, 0.7438053426821253922, -0.6683962987610911899 ) ) ;
#22277=ORIENTED_EDGE ( 'NONE', *, *, #4819, .F. ) ;
#22288=EDGE_CURVE ( 'NONE', #25335, #8224, #19966, .T. ) ;
#22291=CARTESIAN_POINT ( 'NONE',  ( 58.75000000000002132, 6.153735859711025284E-13, 3.111507638930570854E-58 ) ) ;
#22292=CARTESIAN_POINT ( 'NONE',  ( 51.22715433738867574, -0.9941391646896066137, 1.410349289489640556 ) ) ;
#22295=FACE_OUTER_BOUND ( 'NONE', #11109, .T. ) ;
#22301=DIRECTION ( 'NONE',  ( 1.000000000000000000, 1.047444401652940007E-14, 0.000000000000000000 ) ) ;
#22309=DIRECTION ( 'NONE',  ( -0.000000000000000000, -0.000000000000000000, -1.000000000000000000 ) ) ;
#22310=PLANE ( 'NONE',  #1394 ) ;
#22314=CARTESIAN_POINT ( 'NONE',  ( 50.25000000000002842, -1.106298139389803925, -1.666164585742599513 ) ) ;
#22326=CARTESIAN_POINT ( 'NONE',  ( 61.25000000000003553, -0.9999999999993586242, 1.655766640118854438 ) ) ;
#22334=CARTESIAN_POINT ( 'NONE',  ( 58.67159525762716754, -0.4999999999994943489, -1.807104036850090134 ) ) ;
#22336=ORIENTED_EDGE ( 'NONE', *, *, #30508, .T. ) ;
#22339=CARTESIAN_POINT ( 'NONE',  ( 51.45655683570191741, -0.9591657938390838467, -1.611094652690527873 ) ) ;
#22342=DIRECTION ( 'NONE',  ( 0.000000000000000000, 0.000000000000000000, -1.000000000000000000 ) ) ;
#22344=CARTESIAN_POINT ( 'NONE',  ( 58.75000000000004263, -1.253243060177393176, -1.394635017528124132 ) ) ;
#22346=ORIENTED_EDGE ( 'NONE', *, *, #13708, .T. ) ;
#22347=EDGE_CURVE ( 'NONE', #28844, #28012, #29547, .T. ) ;
#22357=FACE_OUTER_BOUND ( 'NONE', #12094, .T. ) ;
#22360=CARTESIAN_POINT ( 'NONE',  ( 51.45655683570189609, 0.9591657938401613182, -1.611094652690528317 ) ) ;
#22371=CARTESIAN_POINT ( 'NONE',  ( 51.31572262954152563, 1.002608958138273554, 1.584424273060082378 ) ) ;
#22379=ORIENTED_EDGE ( 'NONE', *, *, #14883, .T. ) ;
#22382=ORIENTED_EDGE ( 'NONE', *, *, #22855, .F. ) ;
#22383=CARTESIAN_POINT ( 'NONE',  ( 51.25000000000002842, -1.099999999999459410, 1.001327244211406953 ) ) ;
#22385=DIRECTION ( 'NONE',  ( 1.000000000000000000, 1.047444401652940007E-14, 0.000000000000000000 ) ) ;
#22386=ORIENTED_EDGE ( 'NONE', *, *, #30454, .T. ) ;
#22398=CARTESIAN_POINT ( 'NONE',  ( 50.25000000000000000, 2.008165151418772609, -0.5380862305899540843 ) ) ;
#22400=CARTESIAN_POINT ( 'NONE',  ( 58.64999999999999858, 1.872332544501833507, -0.09997921184724666011 ) ) ;
#22405=ORIENTED_EDGE ( 'NONE', *, *, #14110, .F. ) ;
#22408=CIRCLE ( 'NONE', #20899, 0.1500000000000003830 ) ;
#22411=ORIENTED_EDGE ( 'NONE', *, *, #9236, .F. ) ;
#22427=EDGE_CURVE ( 'NONE', #26529, #4543, #28124, .T. ) ;
#22429=CARTESIAN_POINT ( 'NONE',  ( 50.59602332238209499, 0.1408342061609078322, 1.212874140286674063 ) ) ;
#22435=CARTESIAN_POINT ( 'NONE',  ( 58.65000000000003411, -1.571497941946114363, -1.022750809560766694 ) ) ;
#22440=ORIENTED_EDGE ( 'NONE', *, *, #9944, .F. ) ;
#22441=CYLINDRICAL_SURFACE ( 'NONE', #26978, 0.1499999999999998557 ) ;
#22443=( BOUNDED_CURVE ( )  B_SPLINE_CURVE ( 3, ( #25930, #30685, #3933, #18667 ),
 .UNSPECIFIED., .F., .T. ) 
 B_SPLINE_CURVE_WITH_KNOTS ( ( 4, 4 ),
 ( 0.8272220676012492779, 0.8437250283369831516 ),
 .UNSPECIFIED. ) 
 CURVE ( )  GEOMETRIC_REPRESENTATION_ITEM ( )  RATIONAL_B_SPLINE_CURVE ( ( 1.000000000000000000, 0.9999773044860189586, 0.9999773044860189586, 1.000000000000000000 ) ) 
 REPRESENTATION_ITEM ( '' )  );
#22446=CARTESIAN_POINT ( 'NONE',  ( 58.75000000000002132, 6.153735859711025284E-13, 3.111507638930570854E-58 ) ) ;
#22450=CARTESIAN_POINT ( 'NONE',  ( 61.20598745287938414, -0.7563774268552496682, -1.657497327210055493 ) ) ;
#22457=EDGE_LOOP ( 'NONE', ( #4316, #21491, #15121, #14332, #23313, #11280 ) ) ;
#22461=DIRECTION ( 'NONE',  ( 1.000000000000000000, 1.047444401652940007E-14, 0.000000000000000000 ) ) ;
#22464=AXIS2_PLACEMENT_3D ( 'NONE', #29539, #10391, #27919 ) ;
#22465=ORIENTED_EDGE ( 'NONE', *, *, #16997, .T. ) ;
#22470=CIRCLE ( 'NONE', #204, 0.1499999999999999667 ) ;
#22476=EDGE_LOOP ( 'NONE', ( #18538, #19697, #17137, #18796 ) ) ;
#22479=VECTOR ( 'NONE', #9805, 1000.000000000000000 ) ;
#22489=CARTESIAN_POINT ( 'NONE',  ( 50.59602332238209499, 0.1408342061609073048, 0.8215393206232031176 ) ) ;
#22491=CIRCLE ( 'NONE', #20980, 1.975000000000001865 ) ;
#22495=CARTESIAN_POINT ( 'NONE',  ( 58.66118217212504504, -1.337770226785847338, -1.313877211063244621 ) ) ;
#22512=VERTEX_POINT ( 'NONE', #26229 ) ;
#22514=VECTOR ( 'NONE', #7191, 1000.000000000000000 ) ;
#22527=ORIENTED_EDGE ( 'NONE', *, *, #15742, .F. ) ;
#22533=ORIENTED_EDGE ( 'NONE', *, *, #24833, .T. ) ;
#22534=CARTESIAN_POINT ( 'NONE',  ( 61.09423418604053069, -0.6373668173463740150, -1.895722432252557432 ) ) ;
#22535=VERTEX_POINT ( 'NONE', #26708 ) ;
#22544=CARTESIAN_POINT ( 'NONE',  ( 60.97799375661035981, 0.7610968749155430091, 1.436497712332769794 ) ) ;
#22545=LINE ( 'NONE', #27440, #7671 ) ;
#22552=CARTESIAN_POINT ( 'NONE',  ( 50.50000000000001421, 0.7375000000005331735, 3.111507638930570854E-58 ) ) ;
#22553=EDGE_CURVE ( 'NONE', #12097, #29156, #2758, .T. ) ;
#22554=CARTESIAN_POINT ( 'NONE',  ( 58.66324791596930055, -0.4999999999993858246, 1.807104036850105899 ) ) ;
#22556=CARTESIAN_POINT ( 'NONE',  ( 58.75000018595668649, 1.333791840693631103, -1.404395290252168360 ) ) ;
#22559=CARTESIAN_POINT ( 'NONE',  ( 58.65000000000000568, 1.022750809560621921, 1.571497941947222587 ) ) ;
#22560=AXIS2_PLACEMENT_3D ( 'NONE', #12326, #12193, #26441 ) ;
#22582=CIRCLE ( 'NONE', #8897, 2.000000000000000000 ) ;
#22587=AXIS2_PLACEMENT_3D ( 'NONE', #6220, #20342, #18268 ) ;
#22590=AXIS2_PLACEMENT_3D ( 'NONE', #18171, #27812, #3727 ) ;
#22591=CARTESIAN_POINT ( 'NONE',  ( 58.65000000000001990, 6.143261415694495821E-13, 3.111507638930570854E-58 ) ) ;
#22593=CIRCLE ( 'NONE', #8912, 2.000000000000000000 ) ;
#22596=AXIS2_PLACEMENT_3D ( 'NONE', #17292, #26936, #5246 ) ;
#22605=CARTESIAN_POINT ( 'NONE',  ( 51.22715433738867574, -0.9941391646896066137, -1.410349289489640556 ) ) ;
#22608=EDGE_CURVE ( 'NONE', #19129, #19672, #11178, .T. ) ;
#22615=CARTESIAN_POINT ( 'NONE',  ( 58.65000000000001279, 0.8495817349399592544, 1.671477153794648673 ) ) ;
#22616=CARTESIAN_POINT ( 'NONE',  ( 51.31572262954152563, 1.002608958138273554, -1.996089927833914146 ) ) ;
#22617=VECTOR ( 'NONE', #28989, 1000.000000000000000 ) ;
#22620=CARTESIAN_POINT ( 'NONE',  ( 61.25000000000003553, -0.8825412585404734944, -1.623100356595552407 ) ) ;
#22622=CARTESIAN_POINT ( 'NONE',  ( 58.65000000000001990, 6.143261415694495821E-13, 3.111507638930570854E-58 ) ) ;
#22623=AXIS2_PLACEMENT_3D ( 'NONE', #16166, #25814, #14092 ) ;
#22625=CARTESIAN_POINT ( 'NONE',  ( 52.20711756518983293, 0.5000000000005468959, -1.996089927833914146 ) ) ;
#22629=CARTESIAN_POINT ( 'NONE',  ( 51.12687253673781385, -0.9194130538815391551, 1.491219977510798600 ) ) ;
#22634=CARTESIAN_POINT ( 'NONE',  ( 61.25000000000003553, -0.9999999999993586242, 1.863080903344643380 ) ) ;
#22635=CYLINDRICAL_SURFACE ( 'NONE', #26834, 0.2500000000000000000 ) ;
#22638=CARTESIAN_POINT ( 'NONE',  ( 51.59739104186229497, -1.010292945602099701, 1.272765950230261733 ) ) ;
#22639=ORIENTED_EDGE ( 'NONE', *, *, #3944, .F. ) ;
#22657=DIRECTION ( 'NONE',  ( 1.000000000000000000, 1.047444401652940007E-14, 0.000000000000000000 ) ) ;
#22659=CARTESIAN_POINT ( 'NONE',  ( 58.65000038048067665, -1.265626441015677450, 1.383507098106847799 ) ) ;
#22671=CARTESIAN_POINT ( 'NONE',  ( 58.66122797211845352, -1.314214529126519704, -1.337438849764270632 ) ) ;
#22673=ORIENTED_EDGE ( 'NONE', *, *, #13771, .F. ) ;
#22681=DIRECTION ( 'NONE',  ( 1.000000000000000000, 1.047444401652940007E-14, 0.000000000000000000 ) ) ;
#22682=CARTESIAN_POINT ( 'NONE',  ( 58.75000000694010538, -1.856761646087839113, -0.5233439189817360448 ) ) ;
#22687=CARTESIAN_POINT ( 'NONE',  ( 58.64999999999999858, 1.834410884276644227, -0.3880228184651523526 ) ) ;
#22691=DIRECTION ( 'NONE',  ( 0.000000000000000000, -0.8914544820234928668, -0.4531102586349443628 ) ) ;
#22694=CARTESIAN_POINT ( 'NONE',  ( 51.25000000000000711, 1.487500000000536504, 3.111507638930570854E-58 ) ) ;
#22698=EDGE_CURVE ( 'NONE', #12308, #12582, #6247, .T. ) ;
#22712=ORIENTED_EDGE ( 'NONE', *, *, #23414, .F. ) ;
#22719=CARTESIAN_POINT ( 'NONE',  ( 61.25000000000004263, -2.008165151418606520, 0.5380862305909606125 ) ) ;
#22725=DIRECTION ( 'NONE',  ( -9.329605248950888974E-15, 1.000000000000000000, 0.000000000000000000 ) ) ;
#22731=EDGE_CURVE ( 'NONE', #11180, #5002, #2285, .T. ) ;
#22738=VERTEX_POINT ( 'NONE', #29992 ) ;
#22739=VERTEX_POINT ( 'NONE', #13345 ) ;
#22756=CIRCLE ( 'NONE', #30834, 0.2500000000000000000 ) ;
#22762=CARTESIAN_POINT ( 'NONE',  ( 50.59602332238209499, -0.1408342061598474859, 0.8215393206232036727 ) ) ;
#22766=CARTESIAN_POINT ( 'NONE',  ( 50.55260020142763722, 0.05166409867394209515, 0.7900938592415983619 ) ) ;
#22769=ADVANCED_FACE ( 'NONE', ( #4171 ), #13376, .F. ) ;
#22770=DIRECTION ( 'NONE',  ( 0.000000000000000000, 0.000000000000000000, 1.000000000000000000 ) ) ;
#22775=PLANE ( 'NONE',  #13999 ) ;
#22778=CARTESIAN_POINT ( 'NONE',  ( 61.25000000000003553, -0.9999999999993586242, -1.586072192556190030 ) ) ;
#22781=VERTEX_POINT ( 'NONE', #16065 ) ;
#22798=EDGE_CURVE ( 'NONE', #20928, #2824, #18479, .T. ) ;
#22801=CARTESIAN_POINT ( 'NONE',  ( 51.25000000000002842, -0.9938153758920951208, -1.589954715908409977 ) ) ;
#22804=CARTESIAN_POINT ( 'NONE',  ( 58.65266784251146959, -1.873893454697892036, -0.06654060276246864802 ) ) ;
#22810=CARTESIAN_POINT ( 'NONE',  ( 50.25000000000000000, 1.895722432252826328, 0.6373668173479852816 ) ) ;
#22816=DIRECTION ( 'NONE',  ( 0.000000000000000000, 0.000000000000000000, -1.000000000000000000 ) ) ;
#22817=ORIENTED_EDGE ( 'NONE', *, *, #22145, .F. ) ;
#22819=CARTESIAN_POINT ( 'NONE',  ( 58.65000038048047060, 1.008797009996078353, 1.580579251836430332 ) ) ;
#22839=ORIENTED_EDGE ( 'NONE', *, *, #11479, .T. ) ;
#22840=FACE_OUTER_BOUND ( 'NONE', #465, .T. ) ;
#22843=DIRECTION ( 'NONE',  ( 1.000000000000000000, 1.047444401652940007E-14, 0.000000000000000000 ) ) ;
#22845=VERTEX_POINT ( 'NONE', #16858 ) ;
#22851=EDGE_CURVE ( 'NONE', #19841, #27197, #21781, .T. ) ;
#22854=ORIENTED_EDGE ( 'NONE', *, *, #3320, .F. ) ;
#22855=EDGE_CURVE ( 'NONE', #3662, #22512, #26552, .T. ) ;
#22865=CARTESIAN_POINT ( 'NONE',  ( 60.99999998418542901, 0.8156891353822055546, 1.406736638527498195 ) ) ;
#22866=CARTESIAN_POINT ( 'NONE',  ( 60.75000000000001421, 0.5000000000006363798, -1.863080903343375061 ) ) ;
#22879=ORIENTED_EDGE ( 'NONE', *, *, #20028, .F. ) ;
#22880=EDGE_LOOP ( 'NONE', ( #22405, #24225, #18772, #14823 ) ) ;
#22888=ORIENTED_EDGE ( 'NONE', *, *, #4402, .F. ) ;
#22892=CARTESIAN_POINT ( 'NONE',  ( 61.05386123796799325, 0.5990422800903768552, 1.861884024791375714 ) ) ;
#22893=CIRCLE ( 'NONE', #17847, 0.1500000000000001887 ) ;
#22904=DIRECTION ( 'NONE',  ( 0.000000000000000000, 0.000000000000000000, 1.000000000000000000 ) ) ;
#22915=EDGE_LOOP ( 'NONE', ( #24710, #9690, #5687, #27965 ) ) ;
#22917=CYLINDRICAL_SURFACE ( 'NONE', #29693, 2.000000000000000000 ) ;
#22920=VERTEX_POINT ( 'NONE', #12245 ) ;
#22926=CARTESIAN_POINT ( 'NONE',  ( 50.25000000000000000, 1.470078920828055358, -1.320078920826817992 ) ) ;
#22939=B_SPLINE_CURVE_WITH_KNOTS ( 'NONE', 3,
 ( #12159, #12760, #29090, #5319 ),
 .UNSPECIFIED., .F., .F.,
 ( 4, 4 ),
 ( 0.000000000000000000, 0.0003113238203253930773 ),
 .UNSPECIFIED. ) ;
#22953=EDGE_LOOP ( 'NONE', ( #12918, #24417, #26780, #21622 ) ) ;
#22954=ORIENTED_EDGE ( 'NONE', *, *, #29207, .T. ) ;
#22970=AXIS2_PLACEMENT_3D ( 'NONE', #26743, #28802, #283 ) ;
#22983=LINE ( 'NONE', #29943, #15454 ) ;
#22984=EDGE_CURVE ( 'NONE', #17367, #4648, #28174, .T. ) ;
#22986=CARTESIAN_POINT ( 'NONE',  ( 58.65000038048045639, 1.830965513785524967, 0.4043111005673222791 ) ) ;
#22987=CARTESIAN_POINT ( 'NONE',  ( 58.65000000000001990, -0.8794134543721436881, -1.656314228058597848 ) ) ;
#22999=DIRECTION ( 'NONE',  ( 0.000000000000000000, 0.000000000000000000, 1.000000000000000000 ) ) ;
#23012=AXIS2_PLACEMENT_3D ( 'NONE', #11492, #14005, #19103 ) ;
#23014=CARTESIAN_POINT ( 'NONE',  ( 58.65000000000001990, 6.143261415694495821E-13, 3.111507638930570854E-58 ) ) ;
#23015=DIRECTION ( 'NONE',  ( 1.000000000000000000, 1.047444401652940007E-14, 0.000000000000000000 ) ) ;
#23019=DIRECTION ( 'NONE',  ( 1.000000000000000000, 1.047444401652940007E-14, 0.000000000000000000 ) ) ;
#23025=FACE_OUTER_BOUND ( 'NONE', #15269, .T. ) ;
#23031=CARTESIAN_POINT ( 'NONE',  ( 61.25000000000001421, 0.8813478542995215603, -1.623476567772370815 ) ) ;
#23034=VERTEX_POINT ( 'NONE', #6207 ) ;
#23040=CARTESIAN_POINT ( 'NONE',  ( 58.72200624034190497, -1.634766674883864956, 0.9185080301421469917 ) ) ;
#23045=ORIENTED_EDGE ( 'NONE', *, *, #15891, .F. ) ;
#23048=AXIS2_PLACEMENT_3D ( 'NONE', #2366, #2533, #7125 ) ;
#23049=CARTESIAN_POINT ( 'NONE',  ( 51.64281244548084260, -0.8321733326261766539, -1.569379851958523808 ) ) ;
#23054=DIRECTION ( 'NONE',  ( -5.585208838989776544E-16, 0.05332224631852468255, -0.9985773570673163180 ) ) ;
#23055=DIRECTION ( 'NONE',  ( 1.000000000000000000, 1.047444401652940007E-14, 0.000000000000000000 ) ) ;
#23057=CIRCLE ( 'NONE', #10416, 0.1000000000000000333 ) ;
#23059=EDGE_CURVE ( 'NONE', #27852, #19299, #25404, .T. ) ;
#23061=DIRECTION ( 'NONE',  ( 0.8262273428075421755, 0.5633368246415175751, 0.000000000000000000 ) ) ;
#23063=VERTEX_POINT ( 'NONE', #20787 ) ;
#23070=EDGE_LOOP ( 'NONE', ( #7654, #18792, #20485, #8418, #195, #26107, #3126, #3829 ) ) ;
#23074=CARTESIAN_POINT ( 'NONE',  ( 60.98985426489760187, -0.5466942006285966382, 1.538695758318286311 ) ) ;
#23076=EDGE_LOOP ( 'NONE', ( #13249, #16371, #19029, #3913 ) ) ;
#23089=CARTESIAN_POINT ( 'NONE',  ( 58.75000000000000000, 1.877732920581777654, -0.6121634413828943577 ) ) ;
#23105=AXIS2_PLACEMENT_3D ( 'NONE', #9816, #7448, #17118 ) ;
#23107=CIRCLE ( 'NONE', #29159, 0.2500000000000000000 ) ;
#23108=CARTESIAN_POINT ( 'NONE',  ( 58.75000000000004263, -1.964000600390203743, 0.09700564724538153494 ) ) ;
#23111=CARTESIAN_POINT ( 'NONE',  ( 58.75000000000000000, 1.571497941946486288, 1.022750809562083418 ) ) ;
#23114=CARTESIAN_POINT ( 'NONE',  ( 61.25000000000000000, 1.895722432253201140, -0.6373668173460090847 ) ) ;
#23117=VECTOR ( 'NONE', #29321, 1000.000000000000000 ) ;
#23118=ORIENTED_EDGE ( 'NONE', *, *, #18313, .F. ) ;
#23120=DIRECTION ( 'NONE',  ( 1.000000000000000000, 1.047444401652940007E-14, 0.000000000000000000 ) ) ;
#23122=EDGE_CURVE ( 'NONE', #6274, #16870, #10649, .T. ) ;
#23132=ORIENTED_EDGE ( 'NONE', *, *, #13970, .T. ) ;
#23135=CIRCLE ( 'NONE', #21644, 0.1500000000000001887 ) ;
#23141=EDGE_CURVE ( 'NONE', #14302, #29895, #9237, .T. ) ;
#23143=CARTESIAN_POINT ( 'NONE',  ( 50.59602332238209499, -0.1408342061598477080, -1.212874140286674507 ) ) ;
#23151=CARTESIAN_POINT ( 'NONE',  ( 61.01567056675808942, -0.5566600462012117889, -1.706616170210760508 ) ) ;
#23154=CARTESIAN_POINT ( 'NONE',  ( 58.65000045311409593, 1.787855644602297067, 0.5652242121858112034 ) ) ;
#23156=LINE ( 'NONE', #25203, #20113 ) ;
#23160=AXIS2_PLACEMENT_3D ( 'NONE', #5292, #19586, #5624 ) ;
#23164=CARTESIAN_POINT ( 'NONE',  ( 50.25000000000000711, 1.039502773796242119, 1.800471618825331355 ) ) ;
#23168=ORIENTED_EDGE ( 'NONE', *, *, #967, .F. ) ;
#23173=CARTESIAN_POINT ( 'NONE',  ( 58.64999999999999858, 1.872332544501737361, 0.09997921184905503300 ) ) ;
#23193=VERTEX_POINT ( 'NONE', #5049 ) ;
#23195=CARTESIAN_POINT ( 'NONE',  ( 58.65000000000002700, -0.8495817349406442620, 1.671477153793675896 ) ) ;
#23199=CARTESIAN_POINT ( 'NONE',  ( 61.25000000000004263, -1.791164585741916282, 0.8897917884436183922 ) ) ;
#23207=CARTESIAN_POINT ( 'NONE',  ( 58.65000000000004121, -1.834410884275093911, -0.3880228184666750235 ) ) ;
#23209=EDGE_CURVE ( 'NONE', #26303, #25442, #12684, .T. ) ;
#23220=CARTESIAN_POINT ( 'NONE',  ( 58.75000000000000711, 1.800471618824440734, 1.039502773797588597 ) ) ;
#23229=ORIENTED_EDGE ( 'NONE', *, *, #19188, .T. ) ;
#23234=AXIS2_PLACEMENT_3D ( 'NONE', #28498, #6802, #11718 ) ;
#23235=CARTESIAN_POINT ( 'NONE',  ( 60.89332643996541350, -0.4999999999993604560, 1.718465855720804569 ) ) ;
#23240=AXIS2_PLACEMENT_3D ( 'NONE', #25172, #13127, #22816 ) ;
#23250=AXIS2_PLACEMENT_3D ( 'NONE', #6514, #22843, #30091 ) ;
#23252=DIRECTION ( 'NONE',  ( -1.000000000000000000, -1.047444401652940007E-14, 0.000000000000000000 ) ) ;
#23256=FACE_OUTER_BOUND ( 'NONE', #11038, .T. ) ;
#23263=DIRECTION ( 'NONE',  ( 0.000000000000000000, 0.000000000000000000, 1.000000000000000000 ) ) ;
#23266=CARTESIAN_POINT ( 'NONE',  ( 58.65844932252345245, 1.607045716458644913, 0.9660788770032165962 ) ) ;
#23267=ORIENTED_EDGE ( 'NONE', *, *, #12779, .T. ) ;
#23270=CARTESIAN_POINT ( 'NONE',  ( 58.75000000000003553, -1.320082690054269703, 1.469015551795342933 ) ) ;
#23271=ORIENTED_EDGE ( 'NONE', *, *, #20813, .T. ) ;
#23281=PRODUCT_CONTEXT ( 'NONE', #5898, 'mechanical' ) ;
#23283=DIRECTION ( 'NONE',  ( 0.000000000000000000, 0.000000000000000000, 1.000000000000000000 ) ) ;
#23289=CARTESIAN_POINT ( 'NONE',  ( 61.24019690292467999, 0.9013423465692351755, -1.739682280369793999 ) ) ;
#23290=CARTESIAN_POINT ( 'NONE',  ( 51.17950113889408925, 0.9670426259161513105, 1.523577707254208269 ) ) ;
#23295=DIRECTION ( 'NONE',  ( 1.000000000000000000, 1.047444401652940007E-14, 0.000000000000000000 ) ) ;
#23298=LINE ( 'NONE', #21403, #2380 ) ;
#23302=DIRECTION ( 'NONE',  ( 1.000000000000000000, 1.047444401652940007E-14, 0.000000000000000000 ) ) ;
#23312=CARTESIAN_POINT ( 'NONE',  ( 58.75000000000000000, 1.972190280208463653, 0.1053114364810046333 ) ) ;
#23313=ORIENTED_EDGE ( 'NONE', *, *, #8234, .F. ) ;
#23316=EDGE_CURVE ( 'NONE', #5946, #26529, #28505, .T. ) ;
#23318=EDGE_LOOP ( 'NONE', ( #17579, #29752, #4672, #25980 ) ) ;
#23320=VERTEX_POINT ( 'NONE', #145 ) ;
#23325=TOROIDAL_SURFACE ( 'NONE', #13696, 1.975000000000001865, 0.1000000000000000056 ) ;
#23334=CARTESIAN_POINT ( 'NONE',  ( 58.74154451056422488, -1.575232816092377197, -1.017012227664425117 ) ) ;
#23340=EDGE_CURVE ( 'NONE', #7928, #16870, #5239, .T. ) ;
#23343=CARTESIAN_POINT ( 'NONE',  ( 50.25000000000000711, 1.323060376181943720, -1.499837071477343242 ) ) ;
#23346=ORIENTED_EDGE ( 'NONE', *, *, #4617, .T. ) ;
#23347=ORIENTED_EDGE ( 'NONE', *, *, #29207, .F. ) ;
#23349=ORIENTED_EDGE ( 'NONE', *, *, #15574, .F. ) ;
#23350=CARTESIAN_POINT ( 'NONE',  ( 51.34893360928145256, 1.002183861493406436, -1.396106892655430975 ) ) ;
#23356=EDGE_CURVE ( 'NONE', #19192, #2931, #14844, .T. ) ;
#23364=CARTESIAN_POINT ( 'NONE',  ( 61.25000000000001421, 1.000000000000641709, -1.586072192556190474 ) ) ;
#23366=CARTESIAN_POINT ( 'NONE',  ( 58.75000018595669360, 1.404395290252203665, 1.333791840694332320 ) ) ;
#23369=DIRECTION ( 'NONE',  ( 0.000000000000000000, 0.000000000000000000, 1.000000000000000000 ) ) ;
#23378=ORIENTED_EDGE ( 'NONE', *, *, #11433, .T. ) ;
#23384=CARTESIAN_POINT ( 'NONE',  ( 60.82166330297945223, -0.6500000603358897511, 1.489337074527665505 ) ) ;
#23389=VERTEX_POINT ( 'NONE', #30808 ) ;
#23391=ORIENTED_EDGE ( 'NONE', *, *, #27633, .T. ) ;
#23399=FACE_OUTER_BOUND ( 'NONE', #3875, .T. ) ;
#23411=CARTESIAN_POINT ( 'NONE',  ( 61.00000000000002842, -0.8666666666660278739, -1.374595900215364708 ) ) ;
#23414=EDGE_CURVE ( 'NONE', #8262, #20483, #16837, .T. ) ;
#23421=CARTESIAN_POINT ( 'NONE',  ( 58.66122797211808404, -1.337438849764076121, 1.314214529126705777 ) ) ;
#23424=LINE ( 'NONE', #6636, #9601 ) ;
#23426=CARTESIAN_POINT ( 'NONE',  ( 58.65263613458537151, 0.9947326234272455547, 1.589467873455418845 ) ) ;
#23438=CARTESIAN_POINT ( 'NONE',  ( 51.12687253673779253, 0.9194130538826112975, -1.491219977510798378 ) ) ;
#23445=LINE ( 'NONE', #1582, #18043 ) ;
#23446=ADVANCED_FACE ( 'NONE', ( #16248 ), #30636, .T. ) ;
#23448=LINE ( 'NONE', #1915, #12398 ) ;
#23450=CARTESIAN_POINT ( 'NONE',  ( 58.66122797211864537, 1.806862593129175965, 0.5011487553415301388 ) ) ;
#23452=EDGE_LOOP ( 'NONE', ( #13542, #20093, #521, #13695 ) ) ;
#23458=VERTEX_POINT ( 'NONE', #16094 ) ;
#23460=ORIENTED_EDGE ( 'NONE', *, *, #18885, .T. ) ;
#23464=ORIENTED_EDGE ( 'NONE', *, *, #25702, .T. ) ;
#23466=CIRCLE ( 'NONE', #9813, 0.1500000000000001887 ) ;
#23467=EDGE_LOOP ( 'NONE', ( #17043, #21740, #11806, #25627 ) ) ;
#23479=EDGE_CURVE ( 'NONE', #20434, #15271, #30010, .T. ) ;
#23480=CARTESIAN_POINT ( 'NONE',  ( 58.74999999999981526, -1.671477153793549331, -0.8495817349403145258 ) ) ;
#23485=CARTESIAN_POINT ( 'NONE',  ( 51.38214458811558671, -1.084857585945107505, -1.209959298770751923 ) ) ;
#23495=ORIENTED_EDGE ( 'NONE', *, *, #2062, .F. ) ;
#23496=DIRECTION ( 'NONE',  ( -1.000000000000000000, -1.047444401652940007E-14, -0.000000000000000000 ) ) ;
#23505=ORIENTED_EDGE ( 'NONE', *, *, #24867, .F. ) ;
#23509=CARTESIAN_POINT ( 'NONE',  ( 60.88479802533563401, 0.5000000000006354917, -1.718465885608769339 ) ) ;
#23516=CARTESIAN_POINT ( 'NONE',  ( 58.73309930451018346, -0.5681566835778693036, -1.786899855579580310 ) ) ;
#23517=CARTESIAN_POINT ( 'NONE',  ( 58.72204580543434105, -0.9179489429356002539, 1.635081356932753804 ) ) ;
#23521=EDGE_CURVE ( 'NONE', #1478, #30797, #22893, .T. ) ;
#23524=EDGE_CURVE ( 'NONE', #4648, #27829, #10264, .T. ) ;
#23527=AXIS2_PLACEMENT_3D ( 'NONE', #30249, #15219, #24866 ) ;
#23531=DIRECTION ( 'NONE',  ( 1.000000000000000000, 1.047444401652940007E-14, 0.000000000000000000 ) ) ;
#23535=CARTESIAN_POINT ( 'NONE',  ( 58.75000000000000000, 1.996089927834530542, -0.1249999999989956784 ) ) ;
#23542=EDGE_CURVE ( 'NONE', #5737, #7647, #5702, .T. ) ;
#23546=AXIS2_PLACEMENT_3D ( 'NONE', #11150, #26021, #1075 ) ;
#23550=CARTESIAN_POINT ( 'NONE',  ( 58.74154451056406856, 1.832994048939196263, -0.3947215634740703916 ) ) ;
#23564=EDGE_CURVE ( 'NONE', #28412, #7544, #7728, .T. ) ;
#23566=ADVANCED_FACE ( 'NONE', ( #30263 ), #17231, .F. ) ;
#23567=VERTEX_POINT ( 'NONE', #13769 ) ;
#23576=ORIENTED_EDGE ( 'NONE', *, *, #19781, .T. ) ;
#23578=CARTESIAN_POINT ( 'NONE',  ( 58.75000018595672913, -1.333791840694231956, 1.404395290251547079 ) ) ;
#23585=DIRECTION ( 'NONE',  ( 0.000000000000000000, 0.000000000000000000, 1.000000000000000000 ) ) ;
#23593=CARTESIAN_POINT ( 'NONE',  ( 50.55258015808398397, 0.05185913279273118848, -1.177580158083963324 ) ) ;
#23598=EDGE_CURVE ( 'NONE', #21195, #16714, #9946, .T. ) ;
#23609=CIRCLE ( 'NONE', #11991, 0.1500000000000001887 ) ;
#23621=CARTESIAN_POINT ( 'NONE',  ( 58.65844932252355193, 1.802326573994337044, 0.5172264997599709258 ) ) ;
#23630=CIRCLE ( 'NONE', #14510, 0.2499999999999997780 ) ;
#23635=CARTESIAN_POINT ( 'NONE',  ( 58.74999981404334903, -1.441842230225807819, -1.321446761053086449 ) ) ;
#23636=VERTEX_POINT ( 'NONE', #24351 ) ;
#23645=ADVANCED_FACE ( 'NONE', ( #20397 ), #3595, .F. ) ;
#23650=DIRECTION ( 'NONE',  ( -1.000000000000000000, -1.047444401652940007E-14, -0.000000000000000000 ) ) ;
#23656=FILL_AREA_STYLE ('',( #28062 ) ) ;
#23660=CARTESIAN_POINT ( 'NONE',  ( 58.65000045311413857, -1.580645149930897109, -1.008695754909851416 ) ) ;
#23661=AXIS2_PLACEMENT_3D ( 'NONE', #10087, #19901, #574 ) ;
#23668=ORIENTED_EDGE ( 'NONE', *, *, #27816, .F. ) ;
#23675=ORIENTED_EDGE ( 'NONE', *, *, #9386, .F. ) ;
#23676=CARTESIAN_POINT ( 'NONE',  ( 51.17290532404582848, 0.9646187004851777269, -1.462925393634799232 ) ) ;
#23681=CIRCLE ( 'NONE', #22587, 0.1500000000000001887 ) ;
#23682=CARTESIAN_POINT ( 'NONE',  ( 58.75000000000002132, 6.153735859711025284E-13, 3.111507638930570854E-58 ) ) ;
#23683=ORIENTED_EDGE ( 'NONE', *, *, #8643, .F. ) ;
#23696=CARTESIAN_POINT ( 'NONE',  ( 58.65000000000001990, 6.143261415694495821E-13, 3.111507638930570854E-58 ) ) ;
#23699=EDGE_CURVE ( 'NONE', #18829, #28844, #22408, .T. ) ;
#23704=CARTESIAN_POINT ( 'NONE',  ( 58.73794315689197987, 0.5000000000006152856, -1.843373610710533628 ) ) ;
#23705=EDGE_LOOP ( 'NONE', ( #11242, #17796, #22839, #25513 ) ) ;
#23711=ADVANCED_FACE ( 'NONE', ( #17541 ), #6222, .T. ) ;
#23726=CIRCLE ( 'NONE', #10061, 0.1000000000000001166 ) ;
#23731=CARTESIAN_POINT ( 'NONE',  ( 61.16864364483315342, 0.7080009476653978950, 1.871974308545524490 ) ) ;
#23733=VERTEX_POINT ( 'NONE', #13198 ) ;
#23737=ORIENTED_EDGE ( 'NONE', *, *, #27843, .F. ) ;
#23739=ORIENTED_EDGE ( 'NONE', *, *, #4237, .T. ) ;
#23740=CARTESIAN_POINT ( 'NONE',  ( 50.59602332238209499, -0.1408342061598477080, -1.212874140286674507 ) ) ;
#23741=CARTESIAN_POINT ( 'NONE',  ( 58.72419296898098651, -1.357170035999222035, 1.293880926823872457 ) ) ;
#23748=DIRECTION ( 'NONE',  ( 1.000000000000000000, 1.047444401652940007E-14, 0.000000000000000000 ) ) ;
#23749=CARTESIAN_POINT ( 'NONE',  ( 58.72419296898083019, 0.8985315506027614640, 1.645806614395225242 ) ) ;
#23764=CARTESIAN_POINT ( 'NONE',  ( 61.24672990992799981, 0.9412912739139536189, -1.685898893892158412 ) ) ;
#23768=AXIS2_PLACEMENT_3D ( 'NONE', #6632, #30856, #6781 ) ;
#23769=CARTESIAN_POINT ( 'NONE',  ( 52.06628335902946247, -0.5434431642975677823, 1.718465885608439603 ) ) ;
#23784=LINE ( 'NONE', #4134, #20944 ) ;
#23787=EDGE_CURVE ( 'NONE', #15114, #27829, #11268, .T. ) ;
#23788=CARTESIAN_POINT ( 'NONE',  ( 58.75000000000002132, 6.153735859711025284E-13, 3.111507638930570854E-58 ) ) ;
#23794=EDGE_CURVE ( 'NONE', #12232, #19795, #13661, .T. ) ;
#23800=DIRECTION ( 'NONE',  ( -1.000000000000000000, -1.047444401652940007E-14, 0.000000000000000000 ) ) ;
#23812=CARTESIAN_POINT ( 'NONE',  ( 50.25000000000004263, -1.996089927834392208, -0.1249999999999982098 ) ) ;
#23816=CARTESIAN_POINT ( 'NONE',  ( 58.75000000000002132, 6.153735859711025284E-13, 3.111507638930570854E-58 ) ) ;
#23819=ORIENTED_EDGE ( 'NONE', *, *, #4791, .F. ) ;
#23832=FACE_OUTER_BOUND ( 'NONE', #12387, .T. ) ;
#23839=CARTESIAN_POINT ( 'NONE',  ( 51.43641343869300186, -0.9728999281633509133, 1.446772403416499930 ) ) ;
#23845=DIRECTION ( 'NONE',  ( 0.000000000000000000, 0.000000000000000000, 1.000000000000000000 ) ) ;
#23850=ADVANCED_FACE ( 'NONE', ( #30139 ), #3970, .T. ) ;
#23853=CARTESIAN_POINT ( 'NONE',  ( 58.75000000000001421, 0.5000000000003640421, -1.863080903343440786 ) ) ;
#23859=ORIENTED_EDGE ( 'NONE', *, *, #25005, .T. ) ;
#23860=EDGE_LOOP ( 'NONE', ( #14592, #9045, #408, #29392 ) ) ;
#23867=ORIENTED_EDGE ( 'NONE', *, *, #2293, .T. ) ;
#23886=VERTEX_POINT ( 'NONE', #9251 ) ;
#23889=VERTEX_POINT ( 'NONE', #14146 ) ;
#23895=CARTESIAN_POINT ( 'NONE',  ( 61.25000000000001421, 1.039502773797213120, -1.650471618823823539 ) ) ;
#23896=CARTESIAN_POINT ( 'NONE',  ( 58.65000000000002700, -0.5540123067490997366, 1.791510860176260600 ) ) ;
#23897=CARTESIAN_POINT ( 'NONE',  ( 58.73371041428920591, 0.8671977075797476786, 1.662559130998980894 ) ) ;
#23900=CARTESIAN_POINT ( 'NONE',  ( 61.24891880570152836, 0.9671362613610259285, 1.669082548207006633 ) ) ;
#23915=B_SPLINE_CURVE_WITH_KNOTS ( 'NONE', 3,
 ( #3695, #30134, #20508, #30443, #27610, #23195 ),
 .UNSPECIFIED., .F., .F.,
 ( 4, 2, 4 ),
 ( 0.000000000000000000, 0.0001000270069598648232, 0.0002000540139197296463 ),
 .UNSPECIFIED. ) ;
#23917=CARTESIAN_POINT ( 'NONE',  ( 58.65000000000001990, 6.143261415694495821E-13, 3.111507638930570854E-58 ) ) ;
#23918=DIRECTION ( 'NONE',  ( 0.000000000000000000, 0.000000000000000000, 1.000000000000000000 ) ) ;
#23919=CARTESIAN_POINT ( 'NONE',  ( 51.25000000000001421, 5.368152558471320595E-13, 3.111507638930570854E-58 ) ) ;
#23921=EDGE_CURVE ( 'NONE', #5946, #2387, #5199, .T. ) ;
#23937=CARTESIAN_POINT ( 'NONE',  ( 58.74999999999999289, 1.872332544501730256, 0.09997921184905476932 ) ) ;
#23947=AXIS2_PLACEMENT_3D ( 'NONE', #18714, #28510, #26135 ) ;
#23948=DIRECTION ( 'NONE',  ( 0.000000000000000000, 0.000000000000000000, 1.000000000000000000 ) ) ;
#23954=DIRECTION ( 'NONE',  ( 1.000000000000000000, 1.047444401652940007E-14, 0.000000000000000000 ) ) ;
#23966=EDGE_CURVE ( 'NONE', #22535, #24580, #19877, .T. ) ;
#23973=ORIENTED_EDGE ( 'NONE', *, *, #11843, .F. ) ;
#23974=ORIENTED_EDGE ( 'NONE', *, *, #20283, .T. ) ;
#23983=ORIENTED_EDGE ( 'NONE', *, *, #29857, .T. ) ;
#23992=EDGE_CURVE ( 'NONE', #1882, #7461, #13790, .T. ) ;
#23995=AXIS2_PLACEMENT_3D ( 'NONE', #26417, #18993, #139 ) ;
#23996=CARTESIAN_POINT ( 'NONE',  ( 51.59739104186226655, 1.010292945603182391, 1.272765950230260179 ) ) ;
#24001=CARTESIAN_POINT ( 'NONE',  ( 58.66864673770887606, 0.5000000000006145084, -1.807442289571237204 ) ) ;
#24005=CARTESIAN_POINT ( 'NONE',  ( 51.41633779460606490, 0.9865878673145904720, -1.594768911165097558 ) ) ;
#24012=ORIENTED_EDGE ( 'NONE', *, *, #1937, .F. ) ;
#24026=CARTESIAN_POINT ( 'NONE',  ( 61.25000000000002132, 6.415596960124259844E-13, 3.111507638930570854E-58 ) ) ;
#24031=LINE ( 'NONE', #11839, #28534 ) ;
#24051=CARTESIAN_POINT ( 'NONE',  ( 60.75000000000001421, 0.5000000000006363798, 1.863080903344386030 ) ) ;
#24068=CARTESIAN_POINT ( 'NONE',  ( 61.24796382359981806, -0.9549219522834025975, 1.676592304037839209 ) ) ;
#24069=FACE_OUTER_BOUND ( 'NONE', #22880, .T. ) ;
#24083=CARTESIAN_POINT ( 'NONE',  ( 61.25000000000003553, -1.039502773796076474, -1.800471618824325493 ) ) ;
#24086=EDGE_LOOP ( 'NONE', ( #24957, #25135, #25239, #29812 ) ) ;
#24088=LINE ( 'NONE', #8751, #22617 ) ;
#24089=CARTESIAN_POINT ( 'NONE',  ( 58.69321565534330887, 0.5000000000006147305, 1.812725888577170430 ) ) ;
#24105=EDGE_CURVE ( 'NONE', #7417, #30820, #11873, .T. ) ;
#24116=B_SPLINE_CURVE_WITH_KNOTS ( 'NONE', 3,
 ( #30924, #21136, #27918, #13653 ),
 .UNSPECIFIED., .F., .F.,
 ( 4, 4 ),
 ( 2.710505431213761085E-20, 0.0001543670095910070058 ),
 .UNSPECIFIED. ) ;
#24119=CARTESIAN_POINT ( 'NONE',  ( 50.25000000000001421, 0.6373668173475077747, -1.895722432252298084 ) ) ;
#24122=CARTESIAN_POINT ( 'NONE',  ( 58.65000000000001990, 6.143261415694495821E-13, 3.111507638930570854E-58 ) ) ;
#24125=VERTEX_POINT ( 'NONE', #15852 ) ;
#24133=ADVANCED_FACE ( 'NONE', ( #15559 ), #25208, .F. ) ;
#24137=CARTESIAN_POINT ( 'NONE',  ( 51.25000000000001421, 1.100000000000534994, 1.001327244211404732 ) ) ;
#24139=ORIENTED_EDGE ( 'NONE', *, *, #18885, .F. ) ;
#24150=AXIS2_PLACEMENT_3D ( 'NONE', #5928, #23019, #8738 ) ;
#24153=CARTESIAN_POINT ( 'NONE',  ( 58.65815574817527533, 0.5272471384325619903, -1.799565140949186404 ) ) ;
#24154=CIRCLE ( 'NONE', #10493, 1.975000000000001865 ) ;
#24156=VECTOR ( 'NONE', #18509, 1000.000000000000114 ) ;
#24157=CARTESIAN_POINT ( 'NONE',  ( 58.75000018595671492, -0.9248597378508944811, 1.701752411746787930 ) ) ;
#24159=CARTESIAN_POINT ( 'NONE',  ( 58.75000000000000711, 1.039502773796331159, 1.800471618825331355 ) ) ;
#24163=AXIS2_PLACEMENT_3D ( 'NONE', #24716, #21906, #10015 ) ;
#24167=ORIENTED_EDGE ( 'NONE', *, *, #5040, .F. ) ;
#24169=CARTESIAN_POINT ( 'NONE',  ( 58.75000000000002132, 6.153735859711025284E-13, 3.111507638930570854E-58 ) ) ;
#24181=EDGE_CURVE ( 'NONE', #5779, #29991, #26039, .T. ) ;
#24182=ORIENTED_EDGE ( 'NONE', *, *, #25736, .T. ) ;
#24185=CARTESIAN_POINT ( 'NONE',  ( 58.64999999999999858, 1.872332544501833507, -0.09997921184724666011 ) ) ;
#24189=B_SPLINE_CURVE_WITH_KNOTS ( 'NONE', 3,
 ( #28714, #28390, #14288, #16839 ),
 .UNSPECIFIED., .F., .F.,
 ( 4, 4 ),
 ( 4.848699518061080308E-19, 0.0003408895603972687729 ),
 .UNSPECIFIED. ) ;
#24198=CARTESIAN_POINT ( 'NONE',  ( 52.20711756518984004, -0.4999999999994533817, 1.807104036850122109 ) ) ;
#24206=EDGE_LOOP ( 'NONE', ( #23683, #16476, #5396, #31293 ) ) ;
#24211=DIRECTION ( 'NONE',  ( 1.000000000000000000, 1.047444401652940007E-14, 0.000000000000000000 ) ) ;
#24217=AXIS2_PLACEMENT_3D ( 'NONE', #2842, #14864, #7743 ) ;
#24222=CARTESIAN_POINT ( 'NONE',  ( 52.10742411006412311, -0.5153926522284794087, 1.803012591436477408 ) ) ;
#24225=ORIENTED_EDGE ( 'NONE', *, *, #24349, .T. ) ;
#24227=CARTESIAN_POINT ( 'NONE',  ( 58.75000000000000000, 1.394635017528132570, 1.253243060178681922 ) ) ;
#24231=CARTESIAN_POINT ( 'NONE',  ( 58.66107449606962376, 1.301839550768181919, 1.349793924522737054 ) ) ;
#24238=CARTESIAN_POINT ( 'NONE',  ( 58.65000000000001279, 0.8799718970826592157, -1.656030381686704134 ) ) ;
#24243=ORIENTED_EDGE ( 'NONE', *, *, #10323, .T. ) ;
#24244=ORIENTED_EDGE ( 'NONE', *, *, #17773, .T. ) ;
#24247=EDGE_LOOP ( 'NONE', ( #21807, #20096, #23132, #16583, #17343 ) ) ;
#24248=DIRECTION ( 'NONE',  ( 1.000000000000000000, 1.047444401652940007E-14, 0.000000000000000000 ) ) ;
#24249=AXIS2_PLACEMENT_3D ( 'NONE', #2204, #10231, #27174 ) ;
#24252=ORIENTED_EDGE ( 'NONE', *, *, #16827, .T. ) ;
#24269=CARTESIAN_POINT ( 'NONE',  ( 51.59739104186227365, 1.010292945603182169, 1.272765950230260401 ) ) ;
#24274=CARTESIAN_POINT ( 'NONE',  ( 58.66107449606967350, -1.301839550767874165, -1.349793924521847988 ) ) ;
#24276=DIRECTION ( 'NONE',  ( 0.000000000000000000, 0.000000000000000000, 1.000000000000000000 ) ) ;
#24277=CARTESIAN_POINT ( 'NONE',  ( 51.59739104186229497, -1.010292945602101256, 1.272765950230260623 ) ) ;
#24286=EDGE_CURVE ( 'NONE', #25794, #23733, #11367, .T. ) ;
#24301=CARTESIAN_POINT ( 'NONE',  ( 58.65000038048066955, -1.008797009995799465, -1.580579251835824595 ) ) ;
#24303=CARTESIAN_POINT ( 'NONE',  ( 58.65000000000001279, 0.5540123067551541158, -1.791510860174695408 ) ) ;
#24309=CARTESIAN_POINT ( 'NONE',  ( 51.34893360928145256, 1.002183861493406436, 1.396106892655430753 ) ) ;
#24310=CARTESIAN_POINT ( 'NONE',  ( 52.06628335902944826, 0.5434431642986571331, -1.794517909405660694 ) ) ;
#24315=ORIENTED_EDGE ( 'NONE', *, *, #4581, .F. ) ;
#24320=DIRECTION ( 'NONE',  ( 0.000000000000000000, 0.000000000000000000, 1.000000000000000000 ) ) ;
#24331=CARTESIAN_POINT ( 'NONE',  ( 51.12687253673781385, -0.9194130538815391551, 1.491219977510798600 ) ) ;
#24332=CARTESIAN_POINT ( 'NONE',  ( 60.75000000000002842, -0.4999999999993638977, -1.718465885608440047 ) ) ;
#24346=ORIENTED_EDGE ( 'NONE', *, *, #21686, .T. ) ;
#24348=VERTEX_POINT ( 'NONE', #28991 ) ;
#24349=EDGE_CURVE ( 'NONE', #30905, #18829, #9637, .T. ) ;
#24351=CARTESIAN_POINT ( 'NONE',  ( 58.64999999999999858, 1.671477153795419390, -0.8495817349390374362 ) ) ;
#24353=CARTESIAN_POINT ( 'NONE',  ( 60.75000000000002842, -0.4999999999993638977, 1.546164609606623053 ) ) ;
#24355=VERTEX_POINT ( 'NONE', #11590 ) ;
#24364=CARTESIAN_POINT ( 'NONE',  ( 51.31572262954152563, 1.002608958138273554, -1.584424273060082378 ) ) ;
#24371=FACE_OUTER_BOUND ( 'NONE', #22476, .T. ) ;
#24373=ADVANCED_FACE ( 'NONE', ( #21271 ), #14106, .T. ) ;
#24383=CARTESIAN_POINT ( 'NONE',  ( 58.74999981404335614, -1.865327579933669710, 0.5879486190978074900 ) ) ;
#24386=CARTESIAN_POINT ( 'NONE',  ( 58.65000000000003411, -1.022750809560713181, -1.571497941946363497 ) ) ;
#24398=ORIENTED_EDGE ( 'NONE', *, *, #23059, .F. ) ;
#24400=CARTESIAN_POINT ( 'NONE',  ( 58.73379417893114152, -1.381558089341666795, -1.267842757871614490 ) ) ;
#24405=DIRECTION ( 'NONE',  ( 0.000000000000000000, -0.5333333333333335480, -0.8459051693633012903 ) ) ;
#24417=ORIENTED_EDGE ( 'NONE', *, *, #18229, .T. ) ;
#24425=ADVANCED_FACE ( 'NONE', ( #9998 ), #20136, .T. ) ;
#24448=CARTESIAN_POINT ( 'NONE',  ( 58.65266784251146959, -0.9945725797245054123, 1.589569034372780854 ) ) ;
#24453=EDGE_LOOP ( 'NONE', ( #5069, #25502, #26698, #4865, #27530, #17122, #10958, #17496, #6830, #20972, #870, #2622 ) ) ;
#24459=CYLINDRICAL_SURFACE ( 'NONE', #14532, 2.000000000000000000 ) ;
#24460=FACE_OUTER_BOUND ( 'NONE', #30828, .T. ) ;
#24461=ORIENTED_EDGE ( 'NONE', *, *, #31034, .T. ) ;
#24462=EDGE_LOOP ( 'NONE', ( #3233, #18732, #6622, #30948 ) ) ;
#24465=CARTESIAN_POINT ( 'NONE',  ( 50.25000000000002842, -0.4999999999994738653, 1.863080903344643380 ) ) ;
#24470=CARTESIAN_POINT ( 'NONE',  ( 51.12687253673779253, 0.9194130538826112975, -1.491219977510798378 ) ) ;
#24473=AXIS2_PLACEMENT_3D ( 'NONE', #16623, #9656, #5188 ) ;
#24478=ADVANCED_FACE ( 'NONE', ( #11294 ), #4027, .F. ) ;
#24490=ORIENTED_EDGE ( 'NONE', *, *, #30108, .F. ) ;
#24494=CARTESIAN_POINT ( 'NONE',  ( 58.65000000000000568, 1.022750809560621921, 1.571497941947222587 ) ) ;
#24497=FACE_OUTER_BOUND ( 'NONE', #11377, .T. ) ;
#24518=DIRECTION ( 'NONE',  ( 2.775557561562891351E-14, -1.000000000000000000, 0.000000000000000000 ) ) ;
#24522=CARTESIAN_POINT ( 'NONE',  ( 58.72200907981798679, 0.5299537992503529082, 1.799145225589759756 ) ) ;
#24526=VERTEX_POINT ( 'NONE', #27358 ) ;
#24529=DIRECTION ( 'NONE',  ( 1.000000000000000000, 1.047444401652940007E-14, 0.000000000000000000 ) ) ;
#24534=DIRECTION ( 'NONE',  ( 0.000000000000000000, 0.000000000000000000, 1.000000000000000000 ) ) ;
#24536=CARTESIAN_POINT ( 'NONE',  ( 52.20711756518982583, 0.6500000000005481393, 1.489337100860647523 ) ) ;
#24544=VECTOR ( 'NONE', #30954, 1000.000000000000000 ) ;
#24546=AXIS2_PLACEMENT_3D ( 'NONE', #27539, #25331, #15525 ) ;
#24547=EDGE_CURVE ( 'NONE', #29149, #4586, #17131, .T. ) ;
#24548=EDGE_LOOP ( 'NONE', ( #30811, #1062, #13478, #26457 ) ) ;
#24565=AXIS2_PLACEMENT_3D ( 'NONE', #7589, #17248, #12473 ) ;
#24566=DIRECTION ( 'NONE',  ( 0.000000000000000000, 0.000000000000000000, 1.000000000000000000 ) ) ;
#24571=CARTESIAN_POINT ( 'NONE',  ( 61.25000000000002842, -0.8716090598184202953, 1.626546686965557820 ) ) ;
#24580=VERTEX_POINT ( 'NONE', #8199 ) ;
#24595=CARTESIAN_POINT ( 'NONE',  ( 52.20711756518982583, 0.6500000000005479173, -1.489337100860647745 ) ) ;
#24602=AXIS2_PLACEMENT_3D ( 'NONE', #12882, #8300, #10831 ) ;
#24606=CARTESIAN_POINT ( 'NONE',  ( 58.65000000000001279, 0.8495817349399592544, 1.671477153794648673 ) ) ;
#24607=CARTESIAN_POINT ( 'NONE',  ( 60.75000000000002842, -0.6499999999993638644, -1.489337100860647967 ) ) ;
#24608=CARTESIAN_POINT ( 'NONE',  ( 58.75000000000000711, 1.320164791810142679, -1.457351493772217843 ) ) ;
#24612=AXIS2_PLACEMENT_3D ( 'NONE', #27553, #10631, #25018 ) ;
#24617=DIRECTION ( 'NONE',  ( 0.000000000000000000, 0.000000000000000000, -1.000000000000000000 ) ) ;
#24619=CARTESIAN_POINT ( 'NONE',  ( 58.75000000000002132, 6.153735859711025284E-13, 3.111507638930570854E-58 ) ) ;
#24622=ORIENTED_EDGE ( 'NONE', *, *, #20393, .F. ) ;
#24626=CARTESIAN_POINT ( 'NONE',  ( 58.64999999999999858, 1.834410884276226117, 0.3880228184671293268 ) ) ;
#24627=ORIENTED_EDGE ( 'NONE', *, *, #19611, .T. ) ;
#24634=AXIS2_PLACEMENT_3D ( 'NONE', #25786, #13262, #4094 ) ;
#24647=CARTESIAN_POINT ( 'NONE',  ( 51.31943556899496173, -1.088761256243092612, 1.206353010735627729 ) ) ;
#24650=DIRECTION ( 'NONE',  ( 1.000000000000000000, 1.047444401652940007E-14, 0.000000000000000000 ) ) ;
#24651=CARTESIAN_POINT ( 'NONE',  ( 51.45655683570191741, -0.9591657938390837357, -1.468576096419531574 ) ) ;
#24655=AXIS2_PLACEMENT_3D ( 'NONE', #9773, #2955, #27330 ) ;
#24656=ORIENTED_EDGE ( 'NONE', *, *, #10626, .F. ) ;
#24657=( BOUNDED_SURFACE ( )  B_SPLINE_SURFACE ( 3, 2, ( 
 ( #23089, #6928, #18966 ),
 ( #1384, #6289, #11675 ),
 ( #1537, #21355, #30354 ),
 ( #8660, #18811, #11198 ),
 ( #28455, #6457, #18340 ),
 ( #30982, #1849, #14033 ),
 ( #4221, #20871, #13860 ),
 ( #30498, #8980, #9301 ),
 ( #6759, #23550, #4073 ),
 ( #21200, #6609, #16419 ) ),
 .UNSPECIFIED., .F., .F., .F. ) 
 B_SPLINE_SURFACE_WITH_KNOTS ( ( 4, 2, 2, 2, 4 ),
 ( 3, 3 ),
 ( 0.0001706658715691471151, 0.0002229276920778181924, 0.0002751895125864892697, 0.0003274513330951603742, 0.0003797131536038314244 ),
 ( 0.000000000000000000, 1.000000000000000000 ),
 .UNSPECIFIED. ) 
 GEOMETRIC_REPRESENTATION_ITEM ( )  RATIONAL_B_SPLINE_SURFACE ( (
 ( 1.000000000000000000, 0.7071067811865189290, 1.000000000000000000),
 ( 1.000000000000000000, 0.7375607040702090167, 1.000000000000000000),
 ( 1.000000000000000000, 0.7730431127430185123, 1.000000000000000000),
 ( 1.000000000000000000, 0.8321012486991855583, 1.000000000000000000),
 ( 1.000000000000000000, 0.8541932017417042111, 1.000000000000000000),
 ( 1.000000000000000000, 0.8545723906069231379, 1.000000000000000000),
 ( 1.000000000000000000, 0.8327032135054186490, 1.000000000000000000),
 ( 1.000000000000000000, 0.7734559727066918633, 1.000000000000000000),
 ( 1.000000000000000000, 0.7377766653996046253, 1.000000000000000000),
 ( 1.000000000000000000, 0.7071067811865201502, 1.000000000000000000) ) ) 
 REPRESENTATION_ITEM ( '' )  SURFACE ( )  );
#24659=DIRECTION ( 'NONE',  ( 0.000000000000000000, 0.000000000000000000, 1.000000000000000000 ) ) ;
#24660=DIRECTION ( 'NONE',  ( 1.000000000000000000, 1.047444401652940007E-14, 0.000000000000000000 ) ) ;
#24661=VERTEX_POINT ( 'NONE', #31225 ) ;
#24670=EDGE_LOOP ( 'NONE', ( #24461, #7885, #21962, #23668, #1922, #19703 ) ) ;
#24677=CARTESIAN_POINT ( 'NONE',  ( 52.20711756518984714, -0.6499999999994519051, -1.489337100860648633 ) ) ;
#24683=CARTESIAN_POINT ( 'NONE',  ( 52.20711756518982583, 0.7500000000005468959, 1.718465885608440047 ) ) ;
#24684=EDGE_CURVE ( 'NONE', #27461, #2740, #16462, .T. ) ;
#24687=DIRECTION ( 'NONE',  ( 1.000000000000000000, 1.047444401652940007E-14, 0.000000000000000000 ) ) ;
#24688=FACE_OUTER_BOUND ( 'NONE', #17465, .T. ) ;
#24693=PLANE ( 'NONE',  #6002 ) ;
#24695=CARTESIAN_POINT ( 'NONE',  ( 58.73868664959883290, -0.4999999999993850475, -1.844330893389452219 ) ) ;
#24700=ADVANCED_FACE ( 'NONE', ( #28996 ), #20188, .F. ) ;
#24707=CARTESIAN_POINT ( 'NONE',  ( 58.75000000000002132, 6.153735859711025284E-13, 3.111507638930570854E-58 ) ) ;
#24709=CARTESIAN_POINT ( 'NONE',  ( 58.74999999305997989, -1.382203543030976034, -1.345908541130527381 ) ) ;
#24710=ORIENTED_EDGE ( 'NONE', *, *, #4237, .F. ) ;
#24716=CARTESIAN_POINT ( 'NONE',  ( 52.13000000000001677, 0.5000000000005460077, -1.996089927833914146 ) ) ;
#24722=PLANE ( 'NONE',  #18547 ) ;
#24748=AXIS2_PLACEMENT_3D ( 'NONE', #1407, #13263, #8370 ) ;
#24772=ORIENTED_EDGE ( 'NONE', *, *, #9703, .F. ) ;
#24782=CARTESIAN_POINT ( 'NONE',  ( 51.49777277048503521, 1.059151787769027298, -1.232523824083105346 ) ) ;
#24787=B_SPLINE_CURVE_WITH_KNOTS ( 'NONE', 3,
 ( #22534, #15092, #2604, #12703 ),
 .UNSPECIFIED., .F., .F.,
 ( 4, 4 ),
 ( 0.000000000000000000, 0.0003111614939242397359 ),
 .UNSPECIFIED. ) ;
#24788=CARTESIAN_POINT ( 'NONE',  ( 50.25000000000002132, 5.263408118306026973E-13, 0.8749999999999990008 ) ) ;
#24790=DIRECTION ( 'NONE',  ( -1.000000000000000000, -1.047444401652940007E-14, -0.000000000000000000 ) ) ;
#24796=CARTESIAN_POINT ( 'NONE',  ( 50.25000000000002842, -0.4999999999994738653, -1.863080903343643069 ) ) ;
#24797=LINE ( 'NONE', #27177, #26712 ) ;
#24800=CARTESIAN_POINT ( 'NONE',  ( 58.75000000000003553, -1.996089927834303168, -0.1249999999999982098 ) ) ;
#24815=EDGE_CURVE ( 'NONE', #12697, #26529, #10376, .T. ) ;
#24821=EDGE_LOOP ( 'NONE', ( #21573, #2236, #17446, #436 ) ) ;
#24833=EDGE_CURVE ( 'NONE', #27318, #15189, #8359, .T. ) ;
#24839=CARTESIAN_POINT ( 'NONE',  ( 58.75000000000000711, 1.760622601996782999, 0.8948927608044728865 ) ) ;
#24843=ORIENTED_EDGE ( 'NONE', *, *, #23921, .F. ) ;
#24848=VERTEX_POINT ( 'NONE', #11382 ) ;
#24851=DIRECTION ( 'NONE',  ( 0.000000000000000000, -1.000000000000000000, 0.000000000000000000 ) ) ;
#24852=FACE_OUTER_BOUND ( 'NONE', #25286, .T. ) ;
#24866=DIRECTION ( 'NONE',  ( 0.000000000000000000, 0.000000000000000000, 1.000000000000000000 ) ) ;
#24867=EDGE_CURVE ( 'NONE', #10792, #11068, #7838, .T. ) ;
#24869=DIRECTION ( 'NONE',  ( 1.000000000000000000, 1.047444401652940007E-14, 0.000000000000000000 ) ) ;
#24880=LINE ( 'NONE', #823, #13452 ) ;
#24884=CARTESIAN_POINT ( 'NONE',  ( 51.24373197084326392, 0.9939375204961439225, -1.410940055059475062 ) ) ;
#24894=DIRECTION ( 'NONE',  ( 1.000000000000000000, 1.047444401652940007E-14, 0.000000000000000000 ) ) ;
#24895=EDGE_CURVE ( 'NONE', #13972, #21339, #20177, .T. ) ;
#24898=CARTESIAN_POINT ( 'NONE',  ( 51.64281244548096339, 0.8321733326271696374, -1.569379851958313754 ) ) ;
#24899=CARTESIAN_POINT ( 'NONE',  ( 58.72200959573668655, 0.5298027519224196569, -1.799185603788116872 ) ) ;
#24900=DIRECTION ( 'NONE',  ( -8.165490522235077225E-15, 0.5454670984324081484, -0.8381322357049213467 ) ) ;
#24907=EDGE_CURVE ( 'NONE', #21439, #29156, #18490, .T. ) ;
#24911=CARTESIAN_POINT ( 'NONE',  ( 58.73371041428899275, 1.381461519774649149, -1.267950628960770487 ) ) ;
#24916=ORIENTED_EDGE ( 'NONE', *, *, #5579, .T. ) ;
#24917=DIRECTION ( 'NONE',  ( 1.000000000000000000, 1.047444401652940007E-14, 0.000000000000000000 ) ) ;
#24929=CARTESIAN_POINT ( 'NONE',  ( 50.59602332238209499, 0.1408342061609074158, -1.212874140286673841 ) ) ;
#24930=EDGE_CURVE ( 'NONE', #3048, #19414, #29575, .T. ) ;
#24939=CARTESIAN_POINT ( 'NONE',  ( 58.72202590012995671, -0.4851648829343623293, 1.811143295643880213 ) ) ;
#24947=CARTESIAN_POINT ( 'NONE',  ( 51.13585994975462512, -0.9262448312163767961, -1.518514878530177192 ) ) ;
#24949=ORIENTED_EDGE ( 'NONE', *, *, #11316, .F. ) ;
#24957=ORIENTED_EDGE ( 'NONE', *, *, #23598, .F. ) ;
#24958=CARTESIAN_POINT ( 'NONE',  ( 60.99000702708185884, -0.5469907030321375929, -1.538545889480080309 ) ) ;
#24959=CARTESIAN_POINT ( 'NONE',  ( 60.75000000000001421, 0.5000000000006363798, 1.863080903344385808 ) ) ;
#24964=ORIENTED_EDGE ( 'NONE', *, *, #26456, .T. ) ;
#24968=CARTESIAN_POINT ( 'NONE',  ( 58.75000000000000000, 1.671477153795420501, -0.8495817349390359929 ) ) ;
#24973=DIRECTION ( 'NONE',  ( 1.000000000000000000, 1.047444401652940007E-14, 0.000000000000000000 ) ) ;
#24974=AXIS2_PLACEMENT_3D ( 'NONE', #14983, #24650, #28068 ) ;
#24975=ORIENTED_EDGE ( 'NONE', *, *, #6013, .F. ) ;
#24982=CARTESIAN_POINT ( 'NONE',  ( 58.75000000000004974, -1.872332544500606044, -0.09997921184723379540 ) ) ;
#24995=EDGE_LOOP ( 'NONE', ( #4061, #4210, #12884, #20671, #29060, #5584, #16188 ) ) ;
#25000=AXIS2_PLACEMENT_3D ( 'NONE', #1016, #23015, #25526 ) ;
#25005=EDGE_CURVE ( 'NONE', #21960, #21439, #2826, .T. ) ;
#25016=CARTESIAN_POINT ( 'NONE',  ( 58.65838214097819048, -1.819565423306627627, -0.4528606663874174543 ) ) ;
#25018=DIRECTION ( 'NONE',  ( 0.000000000000000000, 0.000000000000000000, 1.000000000000000000 ) ) ;
#25020=DIRECTION ( 'NONE',  ( 9.408669700213139918E-15, -1.000000000000000000, 0.000000000000000000 ) ) ;
#25023=DIRECTION ( 'NONE',  ( 1.000000000000000000, 1.047444401652940007E-14, 0.000000000000000000 ) ) ;
#25034=AXIS2_PLACEMENT_3D ( 'NONE', #4614, #21894, #4930 ) ;
#25037=EDGE_LOOP ( 'NONE', ( #12696, #26912, #27789, #4458 ) ) ;
#25042=CARTESIAN_POINT ( 'NONE',  ( 51.31572262954149011, 1.002608958138273554, -1.395204572094392637 ) ) ;
#25043=EDGE_CURVE ( 'NONE', #7544, #19375, #29417, .T. ) ;
#25055=CARTESIAN_POINT ( 'NONE',  ( 61.25000000000001421, 0.8666666666673038533, 1.374595900215357824 ) ) ;
#25056=CARTESIAN_POINT ( 'NONE',  ( 60.88043801789655163, 0.5128233974954672370, -1.858165151416652394 ) ) ;
#25059=EDGE_CURVE ( 'NONE', #2603, #2931, #19469, .T. ) ;
#25060=CARTESIAN_POINT ( 'NONE',  ( 58.65000000000001990, 6.143261415694495821E-13, 3.111507638930570854E-58 ) ) ;
#25068=CARTESIAN_POINT ( 'NONE',  ( 58.64999999999992752, -1.655311165517189931, 1.077297519403137116 ) ) ;
#25074=ORIENTED_EDGE ( 'NONE', *, *, #19533, .T. ) ;
#25079=ORIENTED_EDGE ( 'NONE', *, *, #27636, .T. ) ;
#25092=EDGE_CURVE ( 'NONE', #29220, #22240, #26586, .T. ) ;
#25097=DIRECTION ( 'NONE',  ( 0.000000000000000000, 0.000000000000000000, 1.000000000000000000 ) ) ;
#25098=CIRCLE ( 'NONE', #23105, 0.1000000000000000749 ) ;
#25102=CIRCLE ( 'NONE', #22623, 2.000000000000000000 ) ;
#25103=CARTESIAN_POINT ( 'NONE',  ( 50.25000000000004263, -2.008165151418721983, 0.5380862305909606125 ) ) ;
#25104=DIRECTION ( 'NONE',  ( 0.000000000000000000, 0.000000000000000000, 1.000000000000000000 ) ) ;
#25106=AXIS2_PLACEMENT_3D ( 'NONE', #29617, #24869, #5881 ) ;
#25107=AXIS2_PLACEMENT_3D ( 'NONE', #19758, #7844, #29387 ) ;
#25110=CARTESIAN_POINT ( 'NONE',  ( 51.49777277048506363, -1.059151787767940389, 1.232523824083111563 ) ) ;
#25112=( BOUNDED_SURFACE ( )  B_SPLINE_SURFACE ( 3, 2, ( 
 ( #27849, #20273, #29903 ),
 ( #23108, #3622, #6011 ),
 ( #20423, #8213, #8363 ),
 ( #27691, #25157, #15809 ),
 ( #15665, #3475, #1399 ),
 ( #10894, #13115, #30365 ),
 ( #11059, #27516, #18352 ),
 ( #5841, #20584, #22804 ),
 ( #25312, #15184, #30218 ),
 ( #13255, #24982, #8525 ) ),
 .UNSPECIFIED., .F., .F., .T. ) 
 B_SPLINE_SURFACE_WITH_KNOTS ( ( 4, 2, 2, 2, 4 ),
 ( 3, 3 ),
 ( 0.0001706658715700577907, 0.0002229276920781165106, 0.0002751895125861752306, 0.0003274513330942339234, 0.0003797131536022926705 ),
 ( 0.000000000000000000, 1.000000000000000000 ),
 .UNSPECIFIED. ) 
 GEOMETRIC_REPRESENTATION_ITEM ( )  RATIONAL_B_SPLINE_SURFACE ( (
 ( 1.000000000000000000, 0.7071067811873469333, 1.000000000000000000),
 ( 1.000000000000000000, 0.7375607040709394324, 1.000000000000000000),
 ( 1.000000000000000000, 0.7730431127427472848, 1.000000000000000000),
 ( 1.000000000000000000, 0.8321012486975403188, 1.000000000000000000),
 ( 1.000000000000000000, 0.8541932017388174092, 1.000000000000000000),
 ( 1.000000000000000000, 0.8545723906033031447, 1.000000000000000000),
 ( 1.000000000000000000, 0.8327032135027588877, 1.000000000000000000),
 ( 1.000000000000000000, 0.7734559727054394207, 1.000000000000000000),
 ( 1.000000000000000000, 0.7377766653992711143, 1.000000000000000000),
 ( 1.000000000000000000, 0.7071067811865520136, 1.000000000000000000) ) ) 
 REPRESENTATION_ITEM ( '' )  SURFACE ( )  );
#25121=CARTESIAN_POINT ( 'NONE',  ( 51.98855675296393031, -0.7791495708602246273, 1.432971607104406075 ) ) ;
#25127=CARTESIAN_POINT ( 'NONE',  ( 61.22059884411349628, -0.7794434480077455651, -1.429589005548589142 ) ) ;
#25135=ORIENTED_EDGE ( 'NONE', *, *, #16330, .T. ) ;
#25141=AXIS2_PLACEMENT_3D ( 'NONE', #20090, #27828, #6136 ) ;
#25144=AXIS2_PLACEMENT_3D ( 'NONE', #20770, #23295, #1578 ) ;
#25146=CARTESIAN_POINT ( 'NONE',  ( 52.06628335902946247, -0.5434431642975651178, 1.718465885608441379 ) ) ;
#25150=AXIS2_PLACEMENT_3D ( 'NONE', #7117, #16625, #11702 ) ;
#25157=CARTESIAN_POINT ( 'NONE',  ( 58.72427158855739293, -1.874564523101702740, 0.04519892032188633363 ) ) ;
#25165=EDGE_CURVE ( 'NONE', #1336, #23034, #17484, .T. ) ;
#25171=DIRECTION ( 'NONE',  ( 1.000000000000000000, 1.047444401652940007E-14, 0.000000000000000000 ) ) ;
#25172=CARTESIAN_POINT ( 'NONE',  ( 61.25000000000002132, 6.415596960124259844E-13, 3.111507638930570854E-58 ) ) ;
#25193=CARTESIAN_POINT ( 'NONE',  ( 60.75000000000001421, 1.000000000000636380, -1.996089927833914146 ) ) ;
#25195=CARTESIAN_POINT ( 'NONE',  ( 58.64999999999999858, 1.793224408422687377, -0.5487562170608069056 ) ) ;
#25201=CARTESIAN_POINT ( 'NONE',  ( 58.65000000000004121, -1.872332544500605822, -0.09997921184723339294 ) ) ;
#25203=CARTESIAN_POINT ( 'NONE',  ( 50.25000000000000000, 1.960427193528716305, -0.3958853607737420899 ) ) ;
#25207=ORIENTED_EDGE ( 'NONE', *, *, #3944, .T. ) ;
#25208=CYLINDRICAL_SURFACE ( 'NONE', #9350, 0.1500000000000003830 ) ;
#25212=ORIENTED_EDGE ( 'NONE', *, *, #28131, .F. ) ;
#25222=AXIS2_PLACEMENT_3D ( 'NONE', #30442, #6552, #20356 ) ;
#25224=CARTESIAN_POINT ( 'NONE',  ( 61.25000000000001421, 0.8825412585414260658, 1.623100356595665206 ) ) ;
#25225=FACE_OUTER_BOUND ( 'NONE', #12736, .T. ) ;
#25230=CARTESIAN_POINT ( 'NONE',  ( 51.31572262954149721, 1.002608958138273554, 1.395204572094392192 ) ) ;
#25239=ORIENTED_EDGE ( 'NONE', *, *, #31034, .F. ) ;
#25242=CARTESIAN_POINT ( 'NONE',  ( 58.64999999999999858, 1.782657835994909901, 0.5811678240991515754 ) ) ;
#25251=ADVANCED_FACE ( 'NONE', ( #1682 ), #31139, .F. ) ;
#25253=DIRECTION ( 'NONE',  ( 1.000000000000000000, 1.047444401652940007E-14, 0.000000000000000000 ) ) ;
#25254=DIRECTION ( 'NONE',  ( 0.000000000000000000, 0.000000000000000000, 1.000000000000000000 ) ) ;
#25260=PLANE ( 'NONE',  #21041 ) ;
#25265=AXIS2_PLACEMENT_3D ( 'NONE', #19051, #14597, #29004 ) ;
#25270=CYLINDRICAL_SURFACE ( 'NONE', #5860, 2.000000000000000000 ) ;
#25271=DIRECTION ( 'NONE',  ( 0.000000000000000000, 0.000000000000000000, 1.000000000000000000 ) ) ;
#25273=CARTESIAN_POINT ( 'NONE',  ( 51.43355796162965987, -0.9748468443428969232, 1.443681521171313653 ) ) ;
#25278=VERTEX_POINT ( 'NONE', #20812 ) ;
#25280=EDGE_LOOP ( 'NONE', ( #1525, #24916, #3906, #5213, #11823 ) ) ;
#25286=EDGE_LOOP ( 'NONE', ( #21895, #2308, #31048, #27957 ) ) ;
#25287=CARTESIAN_POINT ( 'NONE',  ( 50.25000000000000000, 1.895722432253085898, -0.6373668173460090847 ) ) ;
#25291=DIRECTION ( 'NONE',  ( 0.000000000000000000, 0.000000000000000000, 1.000000000000000000 ) ) ;
#25296=CARTESIAN_POINT ( 'NONE',  ( 58.72427158855702345, 1.600821037878942033, -0.9764256747740378550 ) ) ;
#25297=CIRCLE ( 'NONE', #15185, 0.2500000000000003331 ) ;
#25304=EDGE_CURVE ( 'NONE', #15307, #4089, #23915, .T. ) ;
#25305=( BOUNDED_CURVE ( )  B_SPLINE_CURVE ( 3, ( #12680, #14897, #12229, #22360 ),
 .UNSPECIFIED., .F., .T. ) 
 B_SPLINE_CURVE_WITH_KNOTS ( ( 4, 4 ),
 ( 5.006444828673937586, 5.249382619234884473 ),
 .UNSPECIFIED. ) 
 CURVE ( )  GEOMETRIC_REPRESENTATION_ITEM ( )  RATIONAL_B_SPLINE_CURVE ( ( 1.000000000000000000, 0.9950878134350367166, 0.9950878134350367166, 1.000000000000000000 ) ) 
 REPRESENTATION_ITEM ( '' )  );
#25309=ADVANCED_FACE ( 'NONE', ( #1320 ), #5936, .F. ) ;
#25312=CARTESIAN_POINT ( 'NONE',  ( 58.75000000000004263, -1.963941025092382109, -0.09694516907979738862 ) ) ;
#25315=ORIENTED_EDGE ( 'NONE', *, *, #29706, .F. ) ;
#25317=ORIENTED_EDGE ( 'NONE', *, *, #11149, .F. ) ;
#25321=DIRECTION ( 'NONE',  ( 0.000000000000000000, 0.000000000000000000, 1.000000000000000000 ) ) ;
#25322=ORIENTED_EDGE ( 'NONE', *, *, #1726, .F. ) ;
#25331=DIRECTION ( 'NONE',  ( 1.000000000000000000, 1.047444401652940007E-14, 0.000000000000000000 ) ) ;
#25335=VERTEX_POINT ( 'NONE', #4165 ) ;
#25340=CARTESIAN_POINT ( 'NONE',  ( 51.18880157753719828, 1.010242313721750662, -1.292695951881195571 ) ) ;
#25349=EDGE_LOOP ( 'NONE', ( #5692, #6629 ) ) ;
#25351=CARTESIAN_POINT ( 'NONE',  ( 58.65000000000001990, 6.143261415694495821E-13, 3.111507638930570854E-58 ) ) ;
#25353=CARTESIAN_POINT ( 'NONE',  ( 58.64999999999999147, 1.834410884276226117, 0.3880228184671297154 ) ) ;
#25359=ORIENTED_EDGE ( 'NONE', *, *, #12856, .F. ) ;
#25362=ORIENTED_EDGE ( 'NONE', *, *, #17004, .F. ) ;
#25364=DIRECTION ( 'NONE',  ( -1.000000000000000000, -1.018631342913014973E-14, -0.000000000000000000 ) ) ;
#25371=ORIENTED_EDGE ( 'NONE', *, *, #25165, .F. ) ;
#25372=ORIENTED_EDGE ( 'NONE', *, *, #4359, .T. ) ;
#25373=ADVANCED_FACE ( 'NONE', ( #29023 ), #26338, .T. ) ;
#25376=EDGE_CURVE ( 'NONE', #28844, #16661, #22061, .T. ) ;
#25377=CARTESIAN_POINT ( 'NONE',  ( 58.72202590012963697, 0.4851648829358031767, -1.811143295643827811 ) ) ;
#25382=CARTESIAN_POINT ( 'NONE',  ( 58.65000000000001990, 6.143261415694495821E-13, 3.111507638930570854E-58 ) ) ;
#25387=ADVANCED_FACE ( 'NONE', ( #14140 ), #18758, .T. ) ;
#25394=DIRECTION ( 'NONE',  ( 0.000000000000000000, 0.000000000000000000, 1.000000000000000000 ) ) ;
#25395=CARTESIAN_POINT ( 'NONE',  ( 60.99999997330885293, 0.8151934526821700278, -1.407049160682770861 ) ) ;
#25404=CIRCLE ( 'NONE', #15299, 2.000000000000000000 ) ;
#25406=CARTESIAN_POINT ( 'NONE',  ( 58.75000000000003553, -1.932246131436417436, 0.4087173687851147208 ) ) ;
#25408=ADVANCED_FACE ( 'NONE', ( #1958 ), #14451, .F. ) ;
#25410=ADVANCED_FACE ( 'NONE', ( #6862 ), #31184, .F. ) ;
#25418=DIRECTION ( 'NONE',  ( 0.000000000000000000, -1.000000000000000000, 0.000000000000000000 ) ) ;
#25437=CARTESIAN_POINT ( 'NONE',  ( 58.75000000000000711, 1.791164585743217685, -0.8897917884432153812 ) ) ;
#25438=ORIENTED_EDGE ( 'NONE', *, *, #8258, .T. ) ;
#25442=VERTEX_POINT ( 'NONE', #30931 ) ;
#25444=CARTESIAN_POINT ( 'NONE',  ( 58.73379417893117704, 1.582215608939472773, -1.006340787082015131 ) ) ;
#25449=FACE_OUTER_BOUND ( 'NONE', #5599, .T. ) ;
#25457=CARTESIAN_POINT ( 'NONE',  ( 60.75000000000002842, -0.6499999999993638644, -1.489337100860647967 ) ) ;
#25465=CARTESIAN_POINT ( 'NONE',  ( 58.74160516400048238, 0.8556415768453904391, -1.668397168088362026 ) ) ;
#25466=FACE_OUTER_BOUND ( 'NONE', #5047, .T. ) ;
#25481=EDGE_LOOP ( 'NONE', ( #2739, #27934, #3980, #22954, #4169, #24182, #25372, #4618, #26344, #16577, #19111, #7532 ) ) ;
#25495=CARTESIAN_POINT ( 'NONE',  ( 52.06628335902944826, 0.5434431642986583544, 1.718465885608440491 ) ) ;
#25497=CARTESIAN_POINT ( 'NONE',  ( 58.74999999999999289, 1.782657835994903461, 0.5811678240991487998 ) ) ;
#25502=ORIENTED_EDGE ( 'NONE', *, *, #28147, .T. ) ;
#25513=ORIENTED_EDGE ( 'NONE', *, *, #4106, .F. ) ;
#25517=EDGE_LOOP ( 'NONE', ( #3088, #23867, #29469, #5464 ) ) ;
#25521=CARTESIAN_POINT ( 'NONE',  ( 58.75000000000001421, 0.4991259882264960646, -1.863313159664827134 ) ) ;
#25522=PLANE ( 'NONE',  #18304 ) ;
#25526=DIRECTION ( 'NONE',  ( 0.000000000000000000, 0.000000000000000000, 1.000000000000000000 ) ) ;
#25529=CARTESIAN_POINT ( 'NONE',  ( 50.75360625943719839, 0.3719558471750615269, 1.344678919698701236 ) ) ;
#25537=EDGE_CURVE ( 'NONE', #17902, #28408, #24880, .T. ) ;
#25540=ORIENTED_EDGE ( 'NONE', *, *, #30508, .F. ) ;
#25541=EDGE_CURVE ( 'NONE', #7544, #704, #21303, .T. ) ;
#25542=CARTESIAN_POINT ( 'NONE',  ( 61.16418558922026705, 0.6863720863842518449, -1.477277441814810688 ) ) ;
#25556=DIRECTION ( 'NONE',  ( 0.000000000000000000, 0.000000000000000000, 1.000000000000000000 ) ) ;
#25559=EDGE_CURVE ( 'NONE', #1256, #15189, #9933, .T. ) ;
#25562=CARTESIAN_POINT ( 'NONE',  ( 60.75000000000001421, 0.5000000000006363798, -1.718465885608440047 ) ) ;
#25566=CARTESIAN_POINT ( 'NONE',  ( 58.75000000000004263, -2.008165151418633165, 0.5380862305909606125 ) ) ;
#25572=CARTESIAN_POINT ( 'NONE',  ( 51.31572262954152563, 0.7526089581382734428, -1.996089927833914146 ) ) ;
#25581=ORIENTED_EDGE ( 'NONE', *, *, #11843, .T. ) ;
#25585=CARTESIAN_POINT ( 'NONE',  ( 61.20721104068434215, -0.7580073711285438831, 1.657084523451290536 ) ) ;
#25593=DIRECTION ( 'NONE',  ( 1.000000000000000000, 0.000000000000000000, -0.000000000000000000 ) ) ;
#25600=EDGE_CURVE ( 'NONE', #16439, #4172, #6929, .T. ) ;
#25617=DIRECTION ( 'NONE',  ( 0.000000000000000000, 0.000000000000000000, 1.000000000000000000 ) ) ;
#25621=AXIS2_PLACEMENT_3D ( 'NONE', #7737, #9815, #14718 ) ;
#25627=ORIENTED_EDGE ( 'NONE', *, *, #21827, .F. ) ;
#25637=DIRECTION ( 'NONE',  ( 0.000000000000000000, 0.000000000000000000, 1.000000000000000000 ) ) ;
#25643=EDGE_LOOP ( 'NONE', ( #16916, #17734, #15434, #13080 ) ) ;
#25646=CIRCLE ( 'NONE', #30691, 1.487500000000000933 ) ;
#25649=CYLINDRICAL_SURFACE ( 'NONE', #29612, 0.2500000000000000000 ) ;
#25651=EDGE_CURVE ( 'NONE', #5737, #23458, #18035, .T. ) ;
#25661=EDGE_CURVE ( 'NONE', #18852, #23886, #13220, .T. ) ;
#25663=EDGE_CURVE ( 'NONE', #26954, #27318, #10939, .T. ) ;
#25666=CARTESIAN_POINT ( 'NONE',  ( 58.74999999305994436, 1.869977652031684423, 0.4744892162742392339 ) ) ;
#25668=DIRECTION ( 'NONE',  ( 0.000000000000000000, 0.000000000000000000, 1.000000000000000000 ) ) ;
#25675=AXIS2_PLACEMENT_3D ( 'NONE', #14100, #16328, #31039 ) ;
#25676=ORIENTED_EDGE ( 'NONE', *, *, #27228, .T. ) ;
#25680=CARTESIAN_POINT ( 'NONE',  ( 58.65000000000000568, 1.571497941947157084, -1.022750809561052021 ) ) ;
#25681=EDGE_LOOP ( 'NONE', ( #21765, #28734, #52, #2571, #4240, #276, #8180 ) ) ;
#25683=EDGE_CURVE ( 'NONE', #20775, #12730, #22582, .T. ) ;
#25696=EDGE_CURVE ( 'NONE', #7044, #11180, #28658, .T. ) ;
#25702=EDGE_CURVE ( 'NONE', #10186, #16343, #14980, .T. ) ;
#25703=CARTESIAN_POINT ( 'NONE',  ( 58.75000000000003553, -1.895722432252686884, -0.6373668173469783094 ) ) ;
#25705=CARTESIAN_POINT ( 'NONE',  ( 51.25000000000001421, 5.368159983410797313E-13, 3.111507638930570854E-58 ) ) ;
#25715=ORIENTED_EDGE ( 'NONE', *, *, #2364, .T. ) ;
#25719=CARTESIAN_POINT ( 'NONE',  ( 58.74999981196286569, -1.734557215427702026, 0.9033020670135759600 ) ) ;
#25722=ORIENTED_EDGE ( 'NONE', *, *, #29139, .T. ) ;
#25729=CARTESIAN_POINT ( 'NONE',  ( 51.50435016707359637, -0.9265794315402079429, -1.339215852266877116 ) ) ;
#25730=CARTESIAN_POINT ( 'NONE',  ( 58.75000000000002132, -0.5380862305913116650, 2.008165151418990213 ) ) ;
#25732=EDGE_CURVE ( 'NONE', #18525, #4586, #22011, .T. ) ;
#25736=EDGE_CURVE ( 'NONE', #19672, #22738, #8410, .T. ) ;
#25739=DIRECTION ( 'NONE',  ( 1.000000000000000000, 1.047444401652940007E-14, 0.000000000000000000 ) ) ;
#25744=CARTESIAN_POINT ( 'NONE',  ( 61.23770293222996486, -0.8897917884435792013, -1.791164585742600179 ) ) ;
#25746=ORIENTED_EDGE ( 'NONE', *, *, #24684, .F. ) ;
#25747=ORIENTED_EDGE ( 'NONE', *, *, #23316, .F. ) ;
#25758=ORIENTED_EDGE ( 'NONE', *, *, #17860, .F. ) ;
#25780=ORIENTED_EDGE ( 'NONE', *, *, #30363, .T. ) ;
#25781=AXIS2_PLACEMENT_3D ( 'NONE', #15639, #5657, #27964 ) ;
#25783=CARTESIAN_POINT ( 'NONE',  ( 58.75000018803716983, 1.651902078983338740, 1.010830333487720223 ) ) ;
#25786=CARTESIAN_POINT ( 'NONE',  ( 58.64999999999999858, 1.932246131438032366, -0.4087173687832937885 ) ) ;
#25790=FACE_OUTER_BOUND ( 'NONE', #24247, .T. ) ;
#25794=VERTEX_POINT ( 'NONE', #1815 ) ;
#25803=ADVANCED_FACE ( 'NONE', ( #11491 ), #31063, .F. ) ;
#25811=DIRECTION ( 'NONE',  ( 1.000000000000000000, 1.047444401652940007E-14, 0.000000000000000000 ) ) ;
#25814=DIRECTION ( 'NONE',  ( 1.000000000000000000, 1.047444401652940007E-14, 0.000000000000000000 ) ) ;
#25815=DIRECTION ( 'NONE',  ( 0.000000000000000000, 0.000000000000000000, 1.000000000000000000 ) ) ;
#25821=CARTESIAN_POINT ( 'NONE',  ( 51.27134721049148425, 0.9996319491831118231, -1.586319014895851032 ) ) ;
#25826=ORIENTED_EDGE ( 'NONE', *, *, #29744, .F. ) ;
#25831=CARTESIAN_POINT ( 'NONE',  ( 58.72204580543392893, 1.874996463826736459, -0.02257357450714411046 ) ) ;
#25832=ORIENTED_EDGE ( 'NONE', *, *, #20443, .T. ) ;
#25838=ORIENTED_EDGE ( 'NONE', *, *, #21170, .T. ) ;
#25845=DIRECTION ( 'NONE',  ( 0.000000000000000000, 0.000000000000000000, 1.000000000000000000 ) ) ;
#25847=AXIS2_PLACEMENT_3D ( 'NONE', #26701, #19417, #21808 ) ;
#25850=CARTESIAN_POINT ( 'NONE',  ( 58.75000000000003553, -1.655311165516937910, 1.077297519403497050 ) ) ;
#25851=DIRECTION ( 'NONE',  ( 1.000000000000000000, 1.047444401652940007E-14, -0.000000000000000000 ) ) ;
#25855=CARTESIAN_POINT ( 'NONE',  ( 58.75000000000003553, -1.571497941946114141, -1.022750809560766916 ) ) ;
#25860=CARTESIAN_POINT ( 'NONE',  ( 50.95599726996785961, -0.9532299437226279260, -1.316046228059489120 ) ) ;
#25869=ORIENTED_EDGE ( 'NONE', *, *, #5524, .T. ) ;
#25871=ORIENTED_EDGE ( 'NONE', *, *, #23794, .F. ) ;
#25873=CIRCLE ( 'NONE', #19321, 0.1500000000000001887 ) ;
#25875=ORIENTED_EDGE ( 'NONE', *, *, #2077, .T. ) ;
#25877=CARTESIAN_POINT ( 'NONE',  ( 58.65000000000004121, -1.874150328519937680, 0.06593717335357722475 ) ) ;
#25884=CARTESIAN_POINT ( 'NONE',  ( 61.01502350126985874, 0.5557829358563669553, -1.706838207573794453 ) ) ;
#25887=CARTESIAN_POINT ( 'NONE',  ( 50.25000000000001421, 0.5000000000005263567, -1.863080903343375061 ) ) ;
#25892=CARTESIAN_POINT ( 'NONE',  ( 52.06628335902944826, 0.5434431642986583544, -1.718465885608440269 ) ) ;
#25894=CARTESIAN_POINT ( 'NONE',  ( 61.23883361641919976, -0.8947175514078024028, -1.757895546654327124 ) ) ;
#25898=DIRECTION ( 'NONE',  ( -1.000000000000000000, -1.047444401652940007E-14, -0.000000000000000000 ) ) ;
#25913=CARTESIAN_POINT ( 'NONE',  ( 58.64999999999999858, 1.877732920581776321, -0.6121634413828938026 ) ) ;
#25917=FACE_OUTER_BOUND ( 'NONE', #10490, .T. ) ;
#25923=CARTESIAN_POINT ( 'NONE',  ( 61.25000000000001421, 1.039502773797226221, -1.800471618823823450 ) ) ;
#25924=CARTESIAN_POINT ( 'NONE',  ( 58.75000000000001421, 0.6121634413823869858, 1.877732920581527631 ) ) ;
#25928=ORIENTED_EDGE ( 'NONE', *, *, #24867, .T. ) ;
#25929=DIRECTION ( 'NONE',  ( 1.000000000000000000, 1.047444401652940007E-14, 0.000000000000000000 ) ) ;
#25930=CARTESIAN_POINT ( 'NONE',  ( 51.25000000000001421, 1.100000000000537215, 1.196087371390568643 ) ) ;
#25931=PLANE ( 'NONE',  #15628 ) ;
#25934=CARTESIAN_POINT ( 'NONE',  ( 58.72204580543402130, 1.635081356933473895, 0.9179489429359590780 ) ) ;
#25938=CARTESIAN_POINT ( 'NONE',  ( 58.75000000694009827, -1.381609951798472791, 1.346330794794275310 ) ) ;
#25947=ADVANCED_FACE ( 'NONE', ( #8595 ), #17559, .F. ) ;
#25955=EDGE_CURVE ( 'NONE', #2034, #10008, #847, .T. ) ;
#25958=CARTESIAN_POINT ( 'NONE',  ( 58.66133336607592952, -1.640092727267175698, -0.9092995659212040893 ) ) ;
#25959=CARTESIAN_POINT ( 'NONE',  ( 58.75000000000002132, 6.153735859711025284E-13, 3.111507638930570854E-58 ) ) ;
#25962=CARTESIAN_POINT ( 'NONE',  ( 58.65000000000004121, -1.782657835994226225, -0.5811678240974795795 ) ) ;
#25964=CIRCLE ( 'NONE', #30518, 2.000000000000000000 ) ;
#25968=EDGE_LOOP ( 'NONE', ( #10498, #2075, #8833 ) ) ;
#25969=DIRECTION ( 'NONE',  ( 0.000000000000000000, -1.509903313490210686E-14, 1.000000000000000000 ) ) ;
#25978=ADVANCED_FACE ( 'NONE', ( #8443 ), #4393, .F. ) ;
#25979=( BOUNDED_SURFACE ( )  B_SPLINE_SURFACE ( 3, 2, ( 
 ( #14322, #9746, #23996 ),
 ( #14486, #2138, #19408 ),
 ( #28900, #29052, #17039 ),
 ( #24309, #2616, #26835 ),
 ( #26213, #9893, #6899 ),
 ( #11802, #19573, #31110 ),
 ( #394, #5137, #2295 ),
 ( #14790, #22101, #16566 ) ),
 .UNSPECIFIED., .F., .F., .F. ) 
 B_SPLINE_SURFACE_WITH_KNOTS ( ( 4, 2, 2, 4 ),
 ( 3, 3 ),
 ( 0.001762834131042899637, 0.001945267826973971379, 0.002127701522905043122, 0.002492568914767187040 ),
 ( 0.000000000000000000, 1.000000000000000000 ),
 .UNSPECIFIED. ) 
 GEOMETRIC_REPRESENTATION_ITEM ( )  RATIONAL_B_SPLINE_SURFACE ( (
 ( 1.000000000000000000, 0.8699658093904929501, 1.000000000000000000),
 ( 1.000000000000000000, 0.8851796357839230023, 1.000000000000000000),
 ( 1.000000000000000000, 0.8977447492167212051, 1.000000000000000000),
 ( 1.000000000000000000, 0.9127836411835494879, 1.000000000000000000),
 ( 1.000000000000000000, 0.9151168517135812586, 1.000000000000000000),
 ( 1.000000000000000000, 0.9045976586032165034, 1.000000000000000000),
 ( 1.000000000000000000, 0.8745315534097227728, 1.000000000000000000),
 ( 1.000000000000000000, 0.8388746406931710808, 1.000000000000000000) ) ) 
 REPRESENTATION_ITEM ( '' )  SURFACE ( )  );
#25980=ORIENTED_EDGE ( 'NONE', *, *, #7666, .F. ) ;
#25981=CARTESIAN_POINT ( 'NONE',  ( 58.75000000000001421, 0.5000000000004131140, 1.863080903344439321 ) ) ;
#25982=ORIENTED_EDGE ( 'NONE', *, *, #27474, .T. ) ;
#25986=ORIENTED_EDGE ( 'NONE', *, *, #24907, .T. ) ;
#25987=CARTESIAN_POINT ( 'NONE',  ( 0.000000000000000000, 0.000000000000000000, 0.000000000000000000 ) ) ;
#25988=ORIENTED_EDGE ( 'NONE', *, *, #20495, .F. ) ;
#25997=FACE_OUTER_BOUND ( 'NONE', #23860, .T. ) ;
#26003=CARTESIAN_POINT ( 'NONE',  ( 58.65263613458545677, -1.656197658588108856, -0.8791532451975312412 ) ) ;
#26006=CARTESIAN_POINT ( 'NONE',  ( 60.87794714816571684, -0.5123471864359163686, 1.858409133840800198 ) ) ;
#26010=DIRECTION ( 'NONE',  ( 0.000000000000000000, 0.000000000000000000, 1.000000000000000000 ) ) ;
#26021=DIRECTION ( 'NONE',  ( 0.5633368246415009217, 0.8262273428075537218, 0.000000000000000000 ) ) ;
#26022=ORIENTED_EDGE ( 'NONE', *, *, #12017, .F. ) ;
#26025=CARTESIAN_POINT ( 'NONE',  ( 50.25000000000001421, 0.5380862305914526633, -2.008165151417984351 ) ) ;
#26035=ORIENTED_EDGE ( 'NONE', *, *, #13771, .T. ) ;
#26037=CARTESIAN_POINT ( 'NONE',  ( 50.25000000000002132, 5.263408118306026973E-13, 3.111507638930570854E-58 ) ) ;
#26038=DIRECTION ( 'NONE',  ( -4.746078037389309365E-15, 0.4531102586351761219, -0.8914544820233751832 ) ) ;
#26039=CIRCLE ( 'NONE', #5285, 0.1500000000000001887 ) ;
#26040=DIRECTION ( 'NONE',  ( 0.000000000000000000, 0.000000000000000000, 1.000000000000000000 ) ) ;
#26041=CARTESIAN_POINT ( 'NONE',  ( 58.72202590147323065, -0.4851612519489579833, -1.811144268316629447 ) ) ;
#26043=EDGE_CURVE ( 'NONE', #4648, #14207, #29655, .T. ) ;
#26052=CARTESIAN_POINT ( 'NONE',  ( 58.66054497608050866, 0.5000000000006143974, -1.807104036850122109 ) ) ;
#26058=DIRECTION ( 'NONE',  ( 1.000000000000000000, 1.047444401652940007E-14, 0.000000000000000000 ) ) ;
#26060=EDGE_CURVE ( 'NONE', #20284, #10512, #13986, .T. ) ;
#26066=CARTESIAN_POINT ( 'NONE',  ( 51.25000000000002842, -1.099999999999462963, -1.196087371390569087 ) ) ;
#26070=AXIS2_PLACEMENT_3D ( 'NONE', #3326, #15046, #24851 ) ;
#26083=EDGE_CURVE ( 'NONE', #11180, #833, #22111, .T. ) ;
#26093=ORIENTED_EDGE ( 'NONE', *, *, #22553, .T. ) ;
#26106=CARTESIAN_POINT ( 'NONE',  ( 58.65000000000004121, -1.278599783849087235, 1.371849028670080184 ) ) ;
#26107=ORIENTED_EDGE ( 'NONE', *, *, #5788, .T. ) ;
#26110=CYLINDRICAL_SURFACE ( 'NONE', #7193, 2.000000000000000000 ) ;
#26111=CIRCLE ( 'NONE', #5380, 0.1000000000000000888 ) ;
#26115=CARTESIAN_POINT ( 'NONE',  ( 51.24551381660813831, -1.093420264358021532, 1.202138525661323731 ) ) ;
#26116=VERTEX_POINT ( 'NONE', #25850 ) ;
#26121=FACE_OUTER_BOUND ( 'NONE', #2035, .T. ) ;
#26129=EDGE_CURVE ( 'NONE', #4296, #6099, #28679, .T. ) ;
#26135=DIRECTION ( 'NONE',  ( 0.000000000000000000, 0.000000000000000000, 1.000000000000000000 ) ) ;
#26136=AXIS2_PLACEMENT_3D ( 'NONE', #9743, #2134, #11796 ) ;
#26141=LINE ( 'NONE', #30737, #27668 ) ;
#26146=EDGE_CURVE ( 'NONE', #21339, #29648, #793, .T. ) ;
#26151=CARTESIAN_POINT ( 'NONE',  ( 58.72427158855713003, 1.874564523102884017, -0.04519892032209443800 ) ) ;
#26159=ORIENTED_EDGE ( 'NONE', *, *, #15574, .T. ) ;
#26166=DIRECTION ( 'NONE',  ( 1.000000000000000000, 1.047444401652940007E-14, 0.000000000000000000 ) ) ;
#26167=CARTESIAN_POINT ( 'NONE',  ( 58.75000000000000711, 1.469015551797814290, -1.320082690053157037 ) ) ;
#26183=DIRECTION ( 'NONE',  ( 0.000000000000000000, 0.000000000000000000, 1.000000000000000000 ) ) ;
#26185=CIRCLE ( 'NONE', #6985, 1.975000000000001865 ) ;
#26198=FACE_OUTER_BOUND ( 'NONE', #21019, .T. ) ;
#26199=DIRECTION ( 'NONE',  ( 0.000000000000000000, 0.000000000000000000, 1.000000000000000000 ) ) ;
#26201=ORIENTED_EDGE ( 'NONE', *, *, #21270, .F. ) ;
#26202=ORIENTED_EDGE ( 'NONE', *, *, #9189, .T. ) ;
#26212=CARTESIAN_POINT ( 'NONE',  ( 52.20711756518984714, -0.7499999999994533262, 1.718465885608440269 ) ) ;
#26213=CARTESIAN_POINT ( 'NONE',  ( 51.31757909864145972, 1.004435980686513963, 1.391945786376508343 ) ) ;
#26217=CIRCLE ( 'NONE', #7018, 0.2499999999999986955 ) ;
#26218=AXIS2_PLACEMENT_3D ( 'NONE', #20795, #18409, #10507 ) ;
#26227=EDGE_LOOP ( 'NONE', ( #9783, #14961, #8118, #11917 ) ) ;
#26229=CARTESIAN_POINT ( 'NONE',  ( 58.75000000000003553, -1.877732920580616804, -0.6121634413826790855 ) ) ;
#26230=VERTEX_POINT ( 'NONE', #7771 ) ;
#26231=CARTESIAN_POINT ( 'NONE',  ( 58.75000000000000711, 1.470078920828157498, -1.320078920826817992 ) ) ;
#26235=ORIENTED_EDGE ( 'NONE', *, *, #1897, .F. ) ;
#26237=EDGE_CURVE ( 'NONE', #30900, #30820, #30675, .T. ) ;
#26240=CARTESIAN_POINT ( 'NONE',  ( 51.59739104186229497, -1.010292945602101256, -1.272765950230260623 ) ) ;
#26243=CIRCLE ( 'NONE', #30277, 0.1000000000000000333 ) ;
#26248=EDGE_CURVE ( 'NONE', #21490, #17628, #84, .T. ) ;
#26253=DIRECTION ( 'NONE',  ( -0.000000000000000000, -0.000000000000000000, -1.000000000000000000 ) ) ;
#26260=CYLINDRICAL_SURFACE ( 'NONE', #9688, 0.2500000000000000000 ) ;
#26262=CARTESIAN_POINT ( 'NONE',  ( 58.75000000000003553, -1.457266603152898243, 1.320165430233939841 ) ) ;
#26265=CARTESIAN_POINT ( 'NONE',  ( 58.75000000000000000, 1.972190280208464097, 0.1053114364810050774 ) ) ;
#26267=CIRCLE ( 'NONE', #23250, 0.1500000000000001887 ) ;
#26269=CARTESIAN_POINT ( 'NONE',  ( 58.73379417893125520, 1.006340787081485999, 1.582215608939591789 ) ) ;
#26272=CARTESIAN_POINT ( 'NONE',  ( 61.23770293222972327, 0.8897917884438596436, 1.791164585743606041 ) ) ;
#26286=EDGE_CURVE ( 'NONE', #29895, #10800, #15537, .T. ) ;
#26303=VERTEX_POINT ( 'NONE', #4944 ) ;
#26308=CARTESIAN_POINT ( 'NONE',  ( 58.74664129364603582, 0.5000000000006152856, 1.856789660955970200 ) ) ;
#26313=EDGE_CURVE ( 'NONE', #12164, #20434, #10928, .T. ) ;
#26317=EDGE_CURVE ( 'NONE', #21148, #22845, #18238, .T. ) ;
#26328=( BOUNDED_CURVE ( )  B_SPLINE_CURVE ( 3, ( #28948, #7256, #16924, #26568 ),
 .UNSPECIFIED., .F., .T. ) 
 B_SPLINE_CURVE_WITH_KNOTS ( ( 4, 4 ),
 ( 4.094114376165668645, 4.828985806059319152 ),
 .UNSPECIFIED. ) 
 CURVE ( )  GEOMETRIC_REPRESENTATION_ITEM ( )  RATIONAL_B_SPLINE_CURVE ( ( 1.000000000000000000, 0.9555010429016485007, 0.9555010429016485007, 1.000000000000000000 ) ) 
 REPRESENTATION_ITEM ( '' )  );
#26335=CARTESIAN_POINT ( 'NONE',  ( 58.65000000000003411, -1.253243060178072188, 1.394635017527513510 ) ) ;
#26338=CYLINDRICAL_SURFACE ( 'NONE', #299, 2.000000000000000000 ) ;
#26340=ORIENTED_EDGE ( 'NONE', *, *, #26313, .F. ) ;
#26341=CARTESIAN_POINT ( 'NONE',  ( 51.69060524973902204, 0.7995873297242745981, 1.427997211818381684 ) ) ;
#26344=ORIENTED_EDGE ( 'NONE', *, *, #15742, .T. ) ;
#26345=ORIENTED_EDGE ( 'NONE', *, *, #16160, .T. ) ;
#26352=EDGE_LOOP ( 'NONE', ( #20786, #13302, #18005, #25747 ) ) ;
#26354=FACE_OUTER_BOUND ( 'NONE', #13579, .T. ) ;
#26356=ORIENTED_EDGE ( 'NONE', *, *, #4617, .F. ) ;
#26358=FACE_OUTER_BOUND ( 'NONE', #5383, .T. ) ;
#26360=ORIENTED_EDGE ( 'NONE', *, *, #12620, .F. ) ;
#26364=( BOUNDED_SURFACE ( )  B_SPLINE_SURFACE ( 3, 2, ( 
 ( #12910, #8324, #17998 ),
 ( #10388, #8179, #25273 ),
 ( #25110, #20235, #20542 ),
 ( #30176, #27009, #5316 ),
 ( #24647, #19906, #17846 ),
 ( #29534, #2961, #22292 ),
 ( #27483, #17531, #5801 ),
 ( #27181, #5492, #15144 ) ),
 .UNSPECIFIED., .F., .F., .T. ) 
 B_SPLINE_SURFACE_WITH_KNOTS ( ( 4, 2, 2, 4 ),
 ( 3, 3 ),
 ( 0.001762834131042892915, 0.001945267826973966826, 0.002127701522905040520, 0.002492568914767187907 ),
 ( 0.000000000000000000, 1.000000000000000000 ),
 .UNSPECIFIED. ) 
 GEOMETRIC_REPRESENTATION_ITEM ( )  RATIONAL_B_SPLINE_SURFACE ( (
 ( 1.000000000000000000, 0.8699658093904940603, 1.000000000000000000),
 ( 1.000000000000000000, 0.8851796357839156748, 1.000000000000000000),
 ( 1.000000000000000000, 0.8977447492167196508, 1.000000000000000000),
 ( 1.000000000000000000, 0.9127836411835481556, 1.000000000000000000),
 ( 1.000000000000000000, 0.9151168517135812586, 1.000000000000000000),
 ( 1.000000000000000000, 0.9045976586032163924, 1.000000000000000000),
 ( 1.000000000000000000, 0.8745315534097299892, 1.000000000000000000),
 ( 1.000000000000000000, 0.8388746406931726352, 1.000000000000000000) ) ) 
 REPRESENTATION_ITEM ( '' )  SURFACE ( )  );
#26365=CARTESIAN_POINT ( 'NONE',  ( 58.75000000000000711, 1.470078920828144620, -1.470078920826818125 ) ) ;
#26370=DIRECTION ( 'NONE',  ( 1.000000000000000000, 1.047444401652940007E-14, 0.000000000000000000 ) ) ;
#26375=CARTESIAN_POINT ( 'NONE',  ( 51.12687253673779253, 0.9194130538826106314, 1.491219977510798156 ) ) ;
#26379=FACE_OUTER_BOUND ( 'NONE', #7643, .T. ) ;
#26382=ORIENTED_EDGE ( 'NONE', *, *, #7473, .T. ) ;
#26383=CARTESIAN_POINT ( 'NONE',  ( 61.00000000000000711, 0.8111533433300022189, -1.409596402461000597 ) ) ;
#26387=ORIENTED_EDGE ( 'NONE', *, *, #27559, .T. ) ;
#26394=CIRCLE ( 'NONE', #13217, 0.1500000000000000777 ) ;
#26401=CARTESIAN_POINT ( 'NONE',  ( 58.66054497607991891, 0.5000000000007229772, 1.807104036850091910 ) ) ;
#26403=CARTESIAN_POINT ( 'NONE',  ( 52.20711756518983293, 0.5000000000005468959, -1.718465885608440269 ) ) ;
#26407=DIRECTION ( 'NONE',  ( 0.000000000000000000, 0.000000000000000000, 1.000000000000000000 ) ) ;
#26408=DIRECTION ( 'NONE',  ( 2.470865626055588132E-12, -0.5454670984319637261, -0.8381322357052104488 ) ) ;
#26412=ORIENTED_EDGE ( 'NONE', *, *, #5998, .T. ) ;
#26414=CARTESIAN_POINT ( 'NONE',  ( 58.75000000000000711, 1.065927491745594757, -1.652350234724163203 ) ) ;
#26415=CARTESIAN_POINT ( 'NONE',  ( 58.65838214097802705, -1.301971553119757763, 1.349359547237667600 ) ) ;
#26417=CARTESIAN_POINT ( 'NONE',  ( 51.25000000000001421, 5.368152558471320595E-13, 3.111507638930570854E-58 ) ) ;
#26418=ADVANCED_FACE ( 'NONE', ( #22357 ), #15696, .F. ) ;
#26420=FACE_OUTER_BOUND ( 'NONE', #16778, .T. ) ;
#26421=CARTESIAN_POINT ( 'NONE',  ( 58.75000000694006275, 0.9428687169911466048, 1.682988785001243492 ) ) ;
#26422=ORIENTED_EDGE ( 'NONE', *, *, #26567, .F. ) ;
#26424=CARTESIAN_POINT ( 'NONE',  ( 61.23793632918098240, 0.8908246368668226722, 1.774550402280007155 ) ) ;
#26430=CARTESIAN_POINT ( 'NONE',  ( 52.15659567665551322, -0.4999999999994547695, 1.807104036850121886 ) ) ;
#26433=ORIENTED_EDGE ( 'NONE', *, *, #27243, .T. ) ;
#26434=EDGE_CURVE ( 'NONE', #4172, #16714, #10452, .T. ) ;
#26439=DIRECTION ( 'NONE',  ( -1.000000000000000000, -1.047444401652940007E-14, -0.000000000000000000 ) ) ;
#26441=DIRECTION ( 'NONE',  ( 0.000000000000000000, 0.4531102586343168093, 0.8914544820238118339 ) ) ;
#26449=AXIS2_PLACEMENT_3D ( 'NONE', #13299, #18251, #20633 ) ;
#26450=CARTESIAN_POINT ( 'NONE',  ( 58.65000000000001990, 6.143261415694495821E-13, 3.111507638930570854E-58 ) ) ;
#26454=ORIENTED_EDGE ( 'NONE', *, *, #16574, .T. ) ;
#26455=CARTESIAN_POINT ( 'NONE',  ( 51.32256723588026404, -1.004590634318890174, -1.391663617071707826 ) ) ;
#26456=EDGE_CURVE ( 'NONE', #10573, #12424, #9351, .T. ) ;
#26457=ORIENTED_EDGE ( 'NONE', *, *, #19429, .F. ) ;
#26462=EDGE_CURVE ( 'NONE', #16343, #10792, #5353, .T. ) ;
#26464=ORIENTED_EDGE ( 'NONE', *, *, #27816, .T. ) ;
#26466=ORIENTED_EDGE ( 'NONE', *, *, #23564, .F. ) ;
#26467=ORIENTED_EDGE ( 'NONE', *, *, #26146, .F. ) ;
#26472=CIRCLE ( 'NONE', #5221, 2.000000000000000000 ) ;
#26478=CARTESIAN_POINT ( 'NONE',  ( 58.75000000000000711, 1.320082690054482866, -1.469015551796560182 ) ) ;
#26479=DIRECTION ( 'NONE',  ( 0.000000000000000000, 0.000000000000000000, 1.000000000000000000 ) ) ;
#26482=DIRECTION ( 'NONE',  ( -8.860386339788720432E-15, 0.8459051693633012903, 0.5333333333333336590 ) ) ;
#26485=LINE ( 'NONE', #26803, #22100 ) ;
#26491=DIRECTION ( 'NONE',  ( 1.000000000000000000, 1.047444401652940007E-14, 0.000000000000000000 ) ) ;
#26502=CIRCLE ( 'NONE', #5271, 0.1500000000000003830 ) ;
#26507=CARTESIAN_POINT ( 'NONE',  ( 50.55256015243838164, 0.05146993878642957404, -0.7900664826958426756 ) ) ;
#26512=CARTESIAN_POINT ( 'NONE',  ( 58.65000000000004121, -1.782657835994225781, -0.5811678240974800236 ) ) ;
#26518=CARTESIAN_POINT ( 'NONE',  ( 61.24473505568558096, -0.9276313280769659109, -1.700547749640250350 ) ) ;
#26519=EDGE_CURVE ( 'NONE', #21490, #29648, #26825, .T. ) ;
#26522=EDGE_LOOP ( 'NONE', ( #9291, #19857, #17163, #13730, #12644, #20416 ) ) ;
#26527=CARTESIAN_POINT ( 'NONE',  ( 61.25000000000002132, 6.415596960124259844E-13, 3.111507638930570854E-58 ) ) ;
#26528=CARTESIAN_POINT ( 'NONE',  ( 51.25000000000001421, 0.7500000000005367928, 1.718465885608440269 ) ) ;
#26529=VERTEX_POINT ( 'NONE', #28350 ) ;
#26531=ORIENTED_EDGE ( 'NONE', *, *, #14630, .T. ) ;
#26548=CIRCLE ( 'NONE', #6337, 1.975000000000001865 ) ;
#26549=FACE_OUTER_BOUND ( 'NONE', #22915, .T. ) ;
#26551=DIRECTION ( 'NONE',  ( 0.000000000000000000, 0.000000000000000000, 1.000000000000000000 ) ) ;
#26552=CIRCLE ( 'NONE', #18978, 0.1499999999999998557 ) ;
#26557=VERTEX_POINT ( 'NONE', #8853 ) ;
#26560=AXIS2_PLACEMENT_3D ( 'NONE', #31182, #19322, #11712 ) ;
#26562=DIRECTION ( 'NONE',  ( 0.000000000000000000, 0.000000000000000000, 1.000000000000000000 ) ) ;
#26566=LINE ( 'NONE', #28947, #20450 ) ;
#26567=EDGE_CURVE ( 'NONE', #1256, #22240, #872, .T. ) ;
#26568=CARTESIAN_POINT ( 'NONE',  ( 51.25000000000001421, 1.100000000000534994, -1.001327244211404732 ) ) ;
#26575=AXIS2_PLACEMENT_3D ( 'NONE', #7242, #17222, #26551 ) ;
#26582=EDGE_CURVE ( 'NONE', #12058, #22168, #26674, .T. ) ;
#26586=CIRCLE ( 'NONE', #24565, 0.1000000000000002137 ) ;
#26604=CARTESIAN_POINT ( 'NONE',  ( 58.73097752866983967, -0.4999999999993850475, -1.835761897403959564 ) ) ;
#26607=ORIENTED_EDGE ( 'NONE', *, *, #14517, .T. ) ;
#26614=AXIS2_PLACEMENT_3D ( 'NONE', #15769, #23055, #25104 ) ;
#26617=ORIENTED_EDGE ( 'NONE', *, *, #15428, .T. ) ;
#26619=EDGE_LOOP ( 'NONE', ( #17667, #7796, #21726, #27833 ) ) ;
#26625=B_SPLINE_CURVE_WITH_KNOTS ( 'NONE', 3,
 ( #15101, #3070, #388, #27292, #5608, #12715 ),
 .UNSPECIFIED., .F., .F.,
 ( 4, 2, 4 ),
 ( 9.263427422397553349E-18, 0.0001101512007266922219, 0.0002203024014533751739 ),
 .UNSPECIFIED. ) ;
#26627=VECTOR ( 'NONE', #1656, 1000.000000000000000 ) ;
#26635=CARTESIAN_POINT ( 'NONE',  ( 60.75000000000001421, 0.5000000000006363798, 1.718465885608440047 ) ) ;
#26644=DIRECTION ( 'NONE',  ( 1.000000000000000000, 1.047444401652940007E-14, -0.000000000000000000 ) ) ;
#26647=CARTESIAN_POINT ( 'NONE',  ( 61.25000000000003553, -0.9999999999993586242, 1.655766640118854438 ) ) ;
#26652=DIRECTION ( 'NONE',  ( -1.000000000000000000, -1.047444401652940007E-14, -0.000000000000000000 ) ) ;
#26655=VERTEX_POINT ( 'NONE', #24800 ) ;
#26661=CARTESIAN_POINT ( 'NONE',  ( 60.75000000000001421, 0.5000000000006328271, -1.718465885608478239 ) ) ;
#26665=CARTESIAN_POINT ( 'NONE',  ( 50.25000000000004263, -1.791164585742575976, -0.8897917884440847969 ) ) ;
#26674=CIRCLE ( 'NONE', #25144, 0.1500000000000001887 ) ;
#26682=CARTESIAN_POINT ( 'NONE',  ( 51.25000000000001421, 1.100000000000537215, -1.996089927833914146 ) ) ;
#26689=CARTESIAN_POINT ( 'NONE',  ( 50.80258015808398397, 5.323456221955952384E-13, -1.996089927833914146 ) ) ;
#26697=ORIENTED_EDGE ( 'NONE', *, *, #27488, .F. ) ;
#26698=ORIENTED_EDGE ( 'NONE', *, *, #26146, .T. ) ;
#26699=CARTESIAN_POINT ( 'NONE',  ( 58.69114869172459237, 0.5000000000006147305, -1.811349421029180284 ) ) ;
#26701=CARTESIAN_POINT ( 'NONE',  ( 52.13000000000003098, -0.4999999999994542144, -1.996089927833914146 ) ) ;
#26703=CARTESIAN_POINT ( 'NONE',  ( 58.75000000000002132, 6.153735859711025284E-13, 3.111507638930570854E-58 ) ) ;
#26708=CARTESIAN_POINT ( 'NONE',  ( 58.75000000000002842, -1.106298139390583302, 1.666164585743104443 ) ) ;
#26710=EDGE_LOOP ( 'NONE', ( #18964, #29513, #15480, #11186 ) ) ;
#26712=VECTOR ( 'NONE', #17075, 1000.000000000000000 ) ;
#26718=EDGE_CURVE ( 'NONE', #16137, #12097, #15930, .T. ) ;
#26733=CARTESIAN_POINT ( 'NONE',  ( 58.64999999999999858, 1.782657835995388407, -0.5811678240976838605 ) ) ;
#26740=DIRECTION ( 'NONE',  ( 0.000000000000000000, 0.000000000000000000, 1.000000000000000000 ) ) ;
#26743=CARTESIAN_POINT ( 'NONE',  ( 58.64999999999999858, 1.972190280208463209, 0.1053114364810046055 ) ) ;
#26745=DIRECTION ( 'NONE',  ( 1.000000000000000000, 1.047444401652940007E-14, 0.000000000000000000 ) ) ;
#26752=ADVANCED_FACE ( 'NONE', ( #11312 ), #27482, .F. ) ;
#26764=CARTESIAN_POINT ( 'NONE',  ( 61.25000000000000000, 1.996089927834492350, 0.1250000000010043355 ) ) ;
#26770=CARTESIAN_POINT ( 'NONE',  ( 61.00000000000001421, 0.8112099027105408311, 1.409560742431902103 ) ) ;
#26773=CARTESIAN_POINT ( 'NONE',  ( 58.65000000000000568, 1.671477153794444392, 0.8495817349409554575 ) ) ;
#26780=ORIENTED_EDGE ( 'NONE', *, *, #16973, .T. ) ;
#26781=DIRECTION ( 'NONE',  ( 1.000000000000000000, 1.047444401652940007E-14, -0.000000000000000000 ) ) ;
#26783=ADVANCED_FACE ( 'NONE', ( #8635 ), #30473, .F. ) ;
#26798=CARTESIAN_POINT ( 'NONE',  ( 58.75000000000000711, 1.499837071478669959, -1.323060376180706710 ) ) ;
#26799=CARTESIAN_POINT ( 'NONE',  ( 51.24099374247644789, 1.086790822299314785, -1.208135181987622708 ) ) ;
#26803=CARTESIAN_POINT ( 'NONE',  ( 51.25000000000001421, 0.6500000000005367040, -1.489337100860647967 ) ) ;
#26810=EDGE_LOOP ( 'NONE', ( #17472, #4214, #18909 ) ) ;
#26813=EDGE_LOOP ( 'NONE', ( #7682, #19078, #16538, #30776 ) ) ;
#26821=CARTESIAN_POINT ( 'NONE',  ( 51.14630318392394770, 0.9364487020639118420, -1.503522130792751987 ) ) ;
#26822=EDGE_CURVE ( 'NONE', #17335, #22245, #18311, .T. ) ;
#26825=( BOUNDED_CURVE ( )  B_SPLINE_CURVE ( 3, ( #11396, #18706, #13441, #23143 ),
 .UNSPECIFIED., .F., .T. ) 
 B_SPLINE_CURVE_WITH_KNOTS ( ( 4, 4 ),
 ( 1.817784745758537435, 2.232964403949253551 ),
 .UNSPECIFIED. ) 
 CURVE ( )  GEOMETRIC_REPRESENTATION_ITEM ( )  RATIONAL_B_SPLINE_CURVE ( ( 1.000000000000000000, 0.9856869983806464397, 0.9856869983806464397, 1.000000000000000000 ) ) 
 REPRESENTATION_ITEM ( '' )  );
#26833=DIRECTION ( 'NONE',  ( 1.000000000000000000, 1.047444401652940007E-14, 0.000000000000000000 ) ) ;
#26834=AXIS2_PLACEMENT_3D ( 'NONE', #5198, #7880, #20412 ) ;
#26835=CARTESIAN_POINT ( 'NONE',  ( 51.38214458811555829, 1.084857585946179315, 1.209959298770756808 ) ) ;
#26836=CARTESIAN_POINT ( 'NONE',  ( 52.15659567665549901, 0.5000000000005454526, -1.807104036850122331 ) ) ;
#26840=VERTEX_POINT ( 'NONE', #22762 ) ;
#26843=DIRECTION ( 'NONE',  ( 1.000000000000000000, 1.047444401652940007E-14, 0.000000000000000000 ) ) ;
#26844=CARTESIAN_POINT ( 'NONE',  ( 58.75000000000003553, -1.800471618824212694, -1.039502773796582069 ) ) ;
#26848=ADVANCED_FACE ( 'NONE', ( #6431 ), #16093, .T. ) ;
#26853=CARTESIAN_POINT ( 'NONE',  ( 61.25000000000001421, 1.000000000000641709, 1.586072192556190252 ) ) ;
#26869=ORIENTED_EDGE ( 'NONE', *, *, #13176, .F. ) ;
#26870=CYLINDRICAL_SURFACE ( 'NONE', #8272, 0.1499999999999999667 ) ;
#26871=ORIENTED_EDGE ( 'NONE', *, *, #12385, .F. ) ;
#26875=DIRECTION ( 'NONE',  ( 1.000000000000000000, 1.047444401652940007E-14, 0.000000000000000000 ) ) ;
#26879=CIRCLE ( 'NONE', #29905, 0.09999999999999996392 ) ;
#26884=CARTESIAN_POINT ( 'NONE',  ( 61.24959995150299363, 0.9774770340133932534, 1.663387054287940092 ) ) ;
#26892=CARTESIAN_POINT ( 'NONE',  ( 58.65000000000001990, 6.143261415694495821E-13, 3.111507638930570854E-58 ) ) ;
#26896=AXIS2_PLACEMENT_3D ( 'NONE', #27976, #28614, #4383 ) ;
#26898=CARTESIAN_POINT ( 'NONE',  ( 61.24019690292481499, -0.9013423465685174163, 1.739682280371792178 ) ) ;
#26899=CARTESIAN_POINT ( 'NONE',  ( 58.65000076404082563, 0.5493821916573852215, 1.793020333199914385 ) ) ;
#26902=ORIENTED_EDGE ( 'NONE', *, *, #22288, .F. ) ;
#26903=CARTESIAN_POINT ( 'NONE',  ( 58.73371041428940487, -1.830356084954447793, 0.4073466955389919431 ) ) ;
#26904=ORIENTED_EDGE ( 'NONE', *, *, #9699, .T. ) ;
#26909=CARTESIAN_POINT ( 'NONE',  ( 58.74664129364624898, -0.4999999999993849364, -1.856789660955697308 ) ) ;
#26912=ORIENTED_EDGE ( 'NONE', *, *, #3762, .T. ) ;
#26914=FACE_OUTER_BOUND ( 'NONE', #16746, .T. ) ;
#26936=DIRECTION ( 'NONE',  ( -1.000000000000000000, -1.047444401652940007E-14, -0.000000000000000000 ) ) ;
#26945=CARTESIAN_POINT ( 'NONE',  ( 58.65000000000001990, 6.143261415694495821E-13, 3.111507638930570854E-58 ) ) ;
#26949=ORIENTED_EDGE ( 'NONE', *, *, #14824, .T. ) ;
#26954=VERTEX_POINT ( 'NONE', #19106 ) ;
#26960=CIRCLE ( 'NONE', #29005, 1.875000000000001776 ) ;
#26962=CIRCLE ( 'NONE', #12801, 1.975000000000001865 ) ;
#26967=CARTESIAN_POINT ( 'NONE',  ( 58.72200624034167760, -0.9185080301417619664, -1.634766674884353010 ) ) ;
#26968=DIRECTION ( 'NONE',  ( 0.000000000000000000, 0.000000000000000000, 1.000000000000000000 ) ) ;
#26973=CARTESIAN_POINT ( 'NONE',  ( 50.25000000000000711, 1.039502773797110979, -1.800471618823823450 ) ) ;
#26976=EDGE_CURVE ( 'NONE', #24355, #14302, #12022, .T. ) ;
#26978=AXIS2_PLACEMENT_3D ( 'NONE', #27341, #13085, #22770 ) ;
#26989=ORIENTED_EDGE ( 'NONE', *, *, #27008, .T. ) ;
#26994=( BOUNDED_CURVE ( )  B_SPLINE_CURVE ( 3, ( #2391, #168, #11883, #19345 ),
 .UNSPECIFIED., .F., .T. ) 
 B_SPLINE_CURVE_WITH_KNOTS ( ( 4, 4 ),
 ( 4.041453792691655167, 4.300872134317202722 ),
 .UNSPECIFIED. ) 
 CURVE ( )  GEOMETRIC_REPRESENTATION_ITEM ( )  RATIONAL_B_SPLINE_CURVE ( ( 1.000000000000000000, 0.9943997021150918769, 0.9943997021150918769, 1.000000000000000000 ) ) 
 REPRESENTATION_ITEM ( '' )  );
#27006=CIRCLE ( 'NONE', #4751, 2.000000000000000000 ) ;
#27008=EDGE_CURVE ( 'NONE', #29991, #91, #28433, .T. ) ;
#27009=CARTESIAN_POINT ( 'NONE',  ( 51.36283714269054457, -1.001673184507024805, 1.284520656909109659 ) ) ;
#27021=DIRECTION ( 'NONE',  ( 0.000000000000000000, 0.000000000000000000, 1.000000000000000000 ) ) ;
#27023=EDGE_LOOP ( 'NONE', ( #22074, #24490, #13699, #27573, #8114, #7779 ) ) ;
#27024=DIRECTION ( 'NONE',  ( 1.000000000000000000, 1.047444401652940007E-14, 0.000000000000000000 ) ) ;
#27026=ORIENTED_EDGE ( 'NONE', *, *, #26434, .F. ) ;
#27038=AXIS2_PLACEMENT_3D ( 'NONE', #22398, #2923, #12564 ) ;
#27040=EDGE_CURVE ( 'NONE', #31257, #8227, #30237, .T. ) ;
#27046=EDGE_CURVE ( 'NONE', #9856, #23389, #17806, .T. ) ;
#27048=CARTESIAN_POINT ( 'NONE',  ( 58.64999999999999858, 1.972190280208564683, -0.1053114364790997820 ) ) ;
#27049=DIRECTION ( 'NONE',  ( 1.000000000000000000, 1.047444401652940007E-14, 0.000000000000000000 ) ) ;
#27051=VERTEX_POINT ( 'NONE', #22102 ) ;
#27058=ORIENTED_EDGE ( 'NONE', *, *, #25600, .T. ) ;
#27060=ORIENTED_EDGE ( 'NONE', *, *, #6652, .F. ) ;
#27064=VERTEX_POINT ( 'NONE', #24607 ) ;
#27074=ADVANCED_BREP_SHAPE_REPRESENTATION ( '', ( #15609, #9018 ), #3487 ) ;
#27085=CARTESIAN_POINT ( 'NONE',  ( 51.12687253673781385, -0.9194130538815391551, -1.491219977510798600 ) ) ;
#27092=DIRECTION ( 'NONE',  ( 1.000000000000000000, 1.047444401652940007E-14, 0.000000000000000000 ) ) ;
#27102=EDGE_LOOP ( 'NONE', ( #23349, #3702, #5223, #2502, #9140 ) ) ;
#27104=B_SPLINE_CURVE_WITH_KNOTS ( 'NONE', 3,
 ( #4574, #23896, #2188, #19166 ),
 .UNSPECIFIED., .F., .F.,
 ( 4, 4 ),
 ( 0.000000000000000000, 8.537476505502571882E-05 ),
 .UNSPECIFIED. ) ;
#27109=VERTEX_POINT ( 'NONE', #15105 ) ;
#27110=ORIENTED_EDGE ( 'NONE', *, *, #2643, .T. ) ;
#27122=COLOUR_RGB ( '', 0.08235294, 0.09019608, 0.10196078) ;
#27125=AXIS2_PLACEMENT_3D ( 'NONE', #6425, #13688, #26040 ) ;
#27127=CIRCLE ( 'NONE', #29623, 1.975000000000001865 ) ;
#27134=CARTESIAN_POINT ( 'NONE',  ( 58.65000045311413146, -1.008695754909590070, 1.580645149931285021 ) ) ;
#27137=CIRCLE ( 'NONE', #13471, 0.09999999999999997780 ) ;
#27139=CARTESIAN_POINT ( 'NONE',  ( 52.10742411006411601, 0.5153926522295700918, -1.803012591436477630 ) ) ;
#27142=CIRCLE ( 'NONE', #9953, 0.7375000000000040412 ) ;
#27151=( BOUNDED_SURFACE ( )  B_SPLINE_SURFACE ( 3, 2, ( 
 ( #23270, #27381, #5691 ),
 ( #15342, #3314, #22659 ),
 ( #10605, #8222, #4095 ),
 ( #23578, #21223, #26415 ),
 ( #2033, #13733, #21054 ),
 ( #25938, #2182, #23421 ),
 ( #16771, #23741, #18676 ),
 ( #1881, #9173, #28326 ),
 ( #26262, #30520, #20890 ),
 ( #9005, #1701, #4569 ) ),
 .UNSPECIFIED., .F., .F., .F. ) 
 B_SPLINE_SURFACE_WITH_KNOTS ( ( 4, 2, 2, 2, 4 ),
 ( 3, 3 ),
 ( 0.0001706658715701448250, 0.0002229276920781092194, 0.0002751895125860735866, 0.0003274513330940380081, 0.0003797131536020023753 ),
 ( 0.000000000000000000, 1.000000000000000000 ),
 .UNSPECIFIED. ) 
 GEOMETRIC_REPRESENTATION_ITEM ( )  RATIONAL_B_SPLINE_SURFACE ( (
 ( 1.000000000000000000, 0.7071067811873470443, 1.000000000000000000),
 ( 1.000000000000000000, 0.7375607040708359596, 1.000000000000000000),
 ( 1.000000000000000000, 0.7730431127426509175, 1.000000000000000000),
 ( 1.000000000000000000, 0.8321012486970587041, 1.000000000000000000),
 ( 1.000000000000000000, 0.8541932017381176356, 1.000000000000000000),
 ( 1.000000000000000000, 0.8545723906027663519, 1.000000000000000000),
 ( 1.000000000000000000, 0.8327032135020736581, 1.000000000000000000),
 ( 1.000000000000000000, 0.7734559727054440836, 1.000000000000000000),
 ( 1.000000000000000000, 0.7377766653990520673, 1.000000000000000000),
 ( 1.000000000000000000, 0.7071067811865519026, 1.000000000000000000) ) ) 
 REPRESENTATION_ITEM ( '' )  SURFACE ( )  );
#27152=DIRECTION ( 'NONE',  ( 0.000000000000000000, 0.000000000000000000, 1.000000000000000000 ) ) ;
#27155=CARTESIAN_POINT ( 'NONE',  ( 50.59602332238209499, 0.1408342061609078322, 1.212874140286674063 ) ) ;
#27156=ORIENTED_EDGE ( 'NONE', *, *, #4375, .F. ) ;
#27161=ORIENTED_EDGE ( 'NONE', *, *, #22427, .F. ) ;
#27166=AXIS2_PLACEMENT_3D ( 'NONE', #18054, #10900, #27698 ) ;
#27172=CARTESIAN_POINT ( 'NONE',  ( 58.66107449606978008, 1.802323084877999859, 0.5180360531268706215 ) ) ;
#27174=DIRECTION ( 'NONE',  ( 0.000000000000000000, 0.000000000000000000, 1.000000000000000000 ) ) ;
#27176=CARTESIAN_POINT ( 'NONE',  ( 58.65000000000002700, -0.8495817349395312634, -1.671477153794241666 ) ) ;
#27177=CARTESIAN_POINT ( 'NONE',  ( 50.25000000000000711, 0.8897917884437445135, 1.791164585743606041 ) ) ;
#27181=CARTESIAN_POINT ( 'NONE',  ( 50.95599726996785961, -0.9532299437226279260, 1.316046228059489120 ) ) ;
#27193=DIRECTION ( 'NONE',  ( 1.000000000000000000, 1.047444401652940007E-14, 0.000000000000000000 ) ) ;
#27197=VERTEX_POINT ( 'NONE', #27603 ) ;
#27198=CARTESIAN_POINT ( 'NONE',  ( 60.99999998418545033, -0.8156891353810385992, -1.406736638527428029 ) ) ;
#27202=PLANE ( 'NONE',  #31238 ) ;
#27228=EDGE_CURVE ( 'NONE', #22535, #22261, #2839, .T. ) ;
#27232=CARTESIAN_POINT ( 'NONE',  ( 51.21562071718021514, -0.9844478935104048478, 1.555267182539685766 ) ) ;
#27243=EDGE_CURVE ( 'NONE', #10684, #12730, #1822, .T. ) ;
#27257=DIRECTION ( 'NONE',  ( 0.000000000000000000, 0.000000000000000000, 1.000000000000000000 ) ) ;
#27273=DIRECTION ( 'NONE',  ( 0.000000000000000000, 0.000000000000000000, 1.000000000000000000 ) ) ;
#27274=ORIENTED_EDGE ( 'NONE', *, *, #23992, .F. ) ;
#27281=ORIENTED_EDGE ( 'NONE', *, *, #13473, .T. ) ;
#27283=ORIENTED_EDGE ( 'NONE', *, *, #21938, .F. ) ;
#27284=DIRECTION ( 'NONE',  ( 1.000000000000000000, 1.047444401652940007E-14, 0.000000000000000000 ) ) ;
#27289=CARTESIAN_POINT ( 'NONE',  ( 60.75000000000002842, 0.5000000000006363798, 1.554802467931445165 ) ) ;
#27290=CARTESIAN_POINT ( 'NONE',  ( 50.25000000000001421, 0.5380862305904824394, 2.008165151419250449 ) ) ;
#27292=CARTESIAN_POINT ( 'NONE',  ( 51.24366546300165481, 0.9939151496001219499, 1.410979063385805032 ) ) ;
#27293=DIRECTION ( 'NONE',  ( 0.000000000000000000, 0.000000000000000000, 1.000000000000000000 ) ) ;
#27303=ADVANCED_FACE ( 'NONE', ( #20663 ), #9440, .F. ) ;
#27306=ORIENTED_EDGE ( 'NONE', *, *, #16330, .F. ) ;
#27308=EDGE_CURVE ( 'NONE', #16066, #18954, #3858, .T. ) ;
#27317=CARTESIAN_POINT ( 'NONE',  ( 51.45655683570189609, 0.9591657938401607630, -1.468576096419531130 ) ) ;
#27318=VERTEX_POINT ( 'NONE', #29977 ) ;
#27323=DIRECTION ( 'NONE',  ( 0.000000000000000000, -2.664535259100368992E-15, 1.000000000000000000 ) ) ;
#27329=LINE ( 'NONE', #24796, #22088 ) ;
#27330=DIRECTION ( 'NONE',  ( 0.000000000000000000, 0.8914544820238954337, -0.4531102586341524963 ) ) ;
#27341=CARTESIAN_POINT ( 'NONE',  ( 50.25000000000004263, -2.008165151418462191, -0.5380862305909229759 ) ) ;
#27346=B_SPLINE_CURVE_WITH_KNOTS ( 'NONE', 3,
 ( #16722, #24303, #24153, #13998 ),
 .UNSPECIFIED., .F., .F.,
 ( 4, 4 ),
 ( 0.000000000000000000, 8.537476504122688803E-05 ),
 .UNSPECIFIED. ) ;
#27356=DIRECTION ( 'NONE',  ( 0.000000000000000000, 0.000000000000000000, 1.000000000000000000 ) ) ;
#27358=CARTESIAN_POINT ( 'NONE',  ( 52.20711756518983293, 0.5000000000005468959, 1.718465885608440491 ) ) ;
#27359=CARTESIAN_POINT ( 'NONE',  ( 58.75000000000001421, 0.5000000000003640421, -1.863080903343440786 ) ) ;
#27360=CARTESIAN_POINT ( 'NONE',  ( 58.75000000000000711, 1.760622601997809733, -0.8948927608024527247 ) ) ;
#27363=DIRECTION ( 'NONE',  ( 0.000000000000000000, 6.217248937900896348E-15, 1.000000000000000000 ) ) ;
#27376=CARTESIAN_POINT ( 'NONE',  ( 58.75000000000002132, 6.153735859711025284E-13, 3.111507638930570854E-58 ) ) ;
#27381=CARTESIAN_POINT ( 'NONE',  ( 58.74999999999980105, -1.253243060178207413, 1.394635017527392495 ) ) ;
#27388=ORIENTED_EDGE ( 'NONE', *, *, #10120, .T. ) ;
#27399=CARTESIAN_POINT ( 'NONE',  ( 52.13000000000003098, -0.4999999999994542144, -1.996089927833914146 ) ) ;
#27400=CIRCLE ( 'NONE', #13731, 2.000000000000000000 ) ;
#27406=CARTESIAN_POINT ( 'NONE',  ( 58.73379417893121257, -1.830385781109359344, -0.4072049916502183398 ) ) ;
#27407=CARTESIAN_POINT ( 'NONE',  ( 60.75000000000002842, -0.4999999999993638977, 1.863080903344643380 ) ) ;
#27412=EDGE_CURVE ( 'NONE', #12164, #15114, #17520, .T. ) ;
#27415=CARTESIAN_POINT ( 'NONE',  ( 51.45655683570189609, 0.9591657938401613182, 1.611094652690528317 ) ) ;
#27419=EDGE_CURVE ( 'NONE', #27109, #18954, #11963, .T. ) ;
#27420=ORIENTED_EDGE ( 'NONE', *, *, #24547, .T. ) ;
#27440=CARTESIAN_POINT ( 'NONE',  ( 50.25000000000002842, -0.5380862305904318132, -1.858165151418244010 ) ) ;
#27448=CARTESIAN_POINT ( 'NONE',  ( 51.45655683570189609, 0.9591657938401617622, 1.468576096419531352 ) ) ;
#27449=CARTESIAN_POINT ( 'NONE',  ( 58.75000000000003553, -1.470078920827206925, -1.470078920827526892 ) ) ;
#27450=CARTESIAN_POINT ( 'NONE',  ( 58.65844932252365851, 1.349094575299792043, -1.302247349114688424 ) ) ;
#27455=VERTEX_POINT ( 'NONE', #26798 ) ;
#27461=VERTEX_POINT ( 'NONE', #3512 ) ;
#27465=ORIENTED_EDGE ( 'NONE', *, *, #28524, .F. ) ;
#27471=DIRECTION ( 'NONE',  ( 1.000000000000000000, 1.047444401652940007E-14, -0.000000000000000000 ) ) ;
#27474=EDGE_CURVE ( 'NONE', #10684, #4543, #22593, .T. ) ;
#27482=PLANE ( 'NONE',  #7941 ) ;
#27483=CARTESIAN_POINT ( 'NONE',  ( 51.02976068049119363, -1.019450805964126516, 1.268081568884226407 ) ) ;
#27488=EDGE_CURVE ( 'NONE', #17902, #6274, #27142, .T. ) ;
#27489=DIRECTION ( 'NONE',  ( 0.000000000000000000, -0.9507508458640268056, 0.3099561728516426751 ) ) ;
#27493=CARTESIAN_POINT ( 'NONE',  ( 61.25000000000003553, -0.8666666666660258755, 1.374595900215366262 ) ) ;
#27496=VERTEX_POINT ( 'NONE', #11093 ) ;
#27501=ORIENTED_EDGE ( 'NONE', *, *, #12017, .T. ) ;
#27516=CARTESIAN_POINT ( 'NONE',  ( 58.72419296898093677, -1.874576113083205486, -0.04475215827324158929 ) ) ;
#27517=CARTESIAN_POINT ( 'NONE',  ( 58.72202590147342249, 0.4851612519499358678, 1.811144268316692729 ) ) ;
#27521=VERTEX_POINT ( 'NONE', #20157 ) ;
#27528=CARTESIAN_POINT ( 'NONE',  ( 58.75000000000002132, 6.153735859711025284E-13, 3.111507638930570854E-58 ) ) ;
#27529=CYLINDRICAL_SURFACE ( 'NONE', #23240, 1.875000000000001776 ) ;
#27530=ORIENTED_EDGE ( 'NONE', *, *, #26248, .T. ) ;
#27539=CARTESIAN_POINT ( 'NONE',  ( 58.75000000000002132, 6.153735859711025284E-13, 3.111507638930570854E-58 ) ) ;
#27548=B_SPLINE_CURVE_WITH_KNOTS ( 'NONE', 3,
 ( #26401, #118, #11998, #18973 ),
 .UNSPECIFIED., .F., .F.,
 ( 4, 4 ),
 ( 0.0001159639600970536317, 0.0002000540139203089898 ),
 .UNSPECIFIED. ) ;
#27551=DIRECTION ( 'NONE',  ( 2.457191765101193999E-12, 0.8381322357048476279, -0.5454670984325213912 ) ) ;
#27552=CIRCLE ( 'NONE', #22027, 0.09999999999999989453 ) ;
#27553=CARTESIAN_POINT ( 'NONE',  ( 50.25000000000000000, 1.470078920828055358, -1.470078920826818125 ) ) ;
#27559=EDGE_CURVE ( 'NONE', #20392, #10836, #18928, .T. ) ;
#27573=ORIENTED_EDGE ( 'NONE', *, *, #26313, .T. ) ;
#27575=CARTESIAN_POINT ( 'NONE',  ( 51.25000000000002842, -1.099999999999462963, -1.196087371390569087 ) ) ;
#27593=EDGE_CURVE ( 'NONE', #10800, #16137, #15505, .T. ) ;
#27596=VECTOR ( 'NONE', #26166, 1000.000000000000000 ) ;
#27601=LINE ( 'NONE', #22255, #31178 ) ;
#27603=CARTESIAN_POINT ( 'NONE',  ( 61.25000000000004263, -1.791164585742460735, -0.8897917884440847969 ) ) ;
#27604=CARTESIAN_POINT ( 'NONE',  ( 58.74999981404332061, 1.321446761053438168, -1.441842230226794808 ) ) ;
#27610=CARTESIAN_POINT ( 'NONE',  ( 58.65000000000003411, -0.8799718970823581232, 1.656030381686199870 ) ) ;
#27621=DIRECTION ( 'NONE',  ( 0.000000000000000000, 0.000000000000000000, 1.000000000000000000 ) ) ;
#27626=CARTESIAN_POINT ( 'NONE',  ( 58.66054497607991891, 0.5000000000007229772, 1.807104036850091910 ) ) ;
#27630=CYLINDRICAL_SURFACE ( 'NONE', #4558, 0.2500000000000000000 ) ;
#27632=CIRCLE ( 'NONE', #29226, 0.1500000000000001887 ) ;
#27633=EDGE_CURVE ( 'NONE', #25794, #11615, #19071, .T. ) ;
#27636=EDGE_CURVE ( 'NONE', #4273, #16343, #28024, .T. ) ;
#27637=AXIS2_PLACEMENT_3D ( 'NONE', #23919, #16167, #25815 ) ;
#27638=CARTESIAN_POINT ( 'NONE',  ( 58.64999999999999858, 1.782657835994909901, 0.5811678240991515754 ) ) ;
#27639=AXIS2_PLACEMENT_3D ( 'NONE', #20963, #20237, #29869 ) ;
#27641=AXIS2_PLACEMENT_3D ( 'NONE', #31031, #18387, #23918 ) ;
#27642=FACE_OUTER_BOUND ( 'NONE', #2474, .T. ) ;
#27643=DIRECTION ( 'NONE',  ( 0.000000000000000000, 0.000000000000000000, 1.000000000000000000 ) ) ;
#27649=AXIS2_PLACEMENT_3D ( 'NONE', #25060, #15583, #13039 ) ;
#27653=DIRECTION ( 'NONE',  ( 1.000000000000000000, 1.047444401652940007E-14, 0.000000000000000000 ) ) ;
#27656=ORIENTED_EDGE ( 'NONE', *, *, #8109, .T. ) ;
#27659=CARTESIAN_POINT ( 'NONE',  ( 61.00000000000003553, -0.8666666666660277629, 1.374595900215364930 ) ) ;
#27665=AXIS2_PLACEMENT_3D ( 'NONE', #22446, #26875, #26740 ) ;
#27668=VECTOR ( 'NONE', #1920, 1000.000000000000000 ) ;
#27670=DIRECTION ( 'NONE',  ( 1.000000000000000000, 1.047444401652940007E-14, 0.000000000000000000 ) ) ;
#27674=EDGE_LOOP ( 'NONE', ( #22854, #13854, #21698, #12683 ) ) ;
#27676=CARTESIAN_POINT ( 'NONE',  ( 58.64999999999999858, 1.671477153795419834, -0.8495817349390366591 ) ) ;
#27691=CARTESIAN_POINT ( 'NONE',  ( 58.75000018595672913, -1.936190688449155317, 0.04992417795738181979 ) ) ;
#27695=CARTESIAN_POINT ( 'NONE',  ( 61.25000000000000711, 1.499837071478820505, -1.323060376180830833 ) ) ;
#27698=DIRECTION ( 'NONE',  ( 0.000000000000000000, 0.000000000000000000, 1.000000000000000000 ) ) ;
#27729=DIRECTION ( 'NONE',  ( 1.000000000000000000, 1.047444401652940007E-14, 0.000000000000000000 ) ) ;
#27734=DIRECTION ( 'NONE',  ( 1.000000000000000000, 1.047444401652940007E-14, 0.000000000000000000 ) ) ;
#27735=CARTESIAN_POINT ( 'NONE',  ( 58.73371041428909933, 1.788808215312048588, 0.5624054559947927467 ) ) ;
#27738=ORIENTED_EDGE ( 'NONE', *, *, #30350, .T. ) ;
#27743=ORIENTED_EDGE ( 'NONE', *, *, #16679, .T. ) ;
#27770=EDGE_LOOP ( 'NONE', ( #9128, #2800, #19361, #3164 ) ) ;
#27777=ORIENTED_EDGE ( 'NONE', *, *, #24895, .F. ) ;
#27780=CARTESIAN_POINT ( 'NONE',  ( 61.25000000000001421, 1.000000000000641709, -1.586072192556190474 ) ) ;
#27784=ORIENTED_EDGE ( 'NONE', *, *, #20495, .T. ) ;
#27786=DIRECTION ( 'NONE',  ( -0.000000000000000000, -0.000000000000000000, -1.000000000000000000 ) ) ;
#27789=ORIENTED_EDGE ( 'NONE', *, *, #28236, .F. ) ;
#27790=CARTESIAN_POINT ( 'NONE',  ( 60.99723038499097783, 0.5606956656655598392, 1.857935671878364614 ) ) ;
#27792=DIRECTION ( 'NONE',  ( 1.000000000000000000, 1.047444401652940007E-14, 0.000000000000000000 ) ) ;
#27794=EDGE_CURVE ( 'NONE', #1478, #8275, #25102, .T. ) ;
#27797=CARTESIAN_POINT ( 'NONE',  ( 58.75000000000000711, 1.470078920828144620, -1.470078920826818125 ) ) ;
#27801=CARTESIAN_POINT ( 'NONE',  ( 58.65844932252339561, 1.302247349114951991, 1.349094575299514931 ) ) ;
#27806=CARTESIAN_POINT ( 'NONE',  ( 61.25000000000002132, 6.415596960124259844E-13, 3.111507638930570854E-58 ) ) ;
#27810=DIRECTION ( 'NONE',  ( 0.000000000000000000, 0.000000000000000000, 1.000000000000000000 ) ) ;
#27812=DIRECTION ( 'NONE',  ( 1.000000000000000000, 1.047444401652940007E-14, -0.000000000000000000 ) ) ;
#27816=EDGE_CURVE ( 'NONE', #18829, #779, #23298, .T. ) ;
#27823=CARTESIAN_POINT ( 'NONE',  ( 60.97860563121706434, -0.7618031158890644639, 1.436139941719672075 ) ) ;
#27828=DIRECTION ( 'NONE',  ( 1.000000000000000000, 1.047444401652940007E-14, 0.000000000000000000 ) ) ;
#27829=VERTEX_POINT ( 'NONE', #19338 ) ;
#27830=SPHERICAL_SURFACE ( 'NONE', #8493, 0.2500000000000000000 ) ;
#27833=ORIENTED_EDGE ( 'NONE', *, *, #2782, .T. ) ;
#27840=VERTEX_POINT ( 'NONE', #17403 ) ;
#27843=EDGE_CURVE ( 'NONE', #28852, #1336, #13476, .T. ) ;
#27848=CARTESIAN_POINT ( 'NONE',  ( 60.97363240180333577, -0.7541976959271894376, -1.440084173506624765 ) ) ;
#27849=CARTESIAN_POINT ( 'NONE',  ( 58.75000000000004263, -1.972190280207122726, 0.1053114364788733381 ) ) ;
#27852=VERTEX_POINT ( 'NONE', #26764 ) ;
#27853=CARTESIAN_POINT ( 'NONE',  ( 58.64999999999999858, 1.671477153794443504, 0.8495817349409569008 ) ) ;
#27862=FACE_OUTER_BOUND ( 'NONE', #3439, .T. ) ;
#27867=B_SPLINE_CURVE_WITH_KNOTS ( 'NONE', 3,
 ( #22023, #22334, #4916, #17264, #10445, #15036, #9822, #26604, #24695, #316, #26909, #7907, #3159 ),
 .UNSPECIFIED., .F., .F.,
 ( 4, 3, 3, 3, 4 ),
 ( 0.000000000000000000, 3.315084464037111269E-05, 6.626473632988943725E-05, 9.991171812031440650E-05, 0.0001104636331259644592 ),
 .UNSPECIFIED. ) ;
#27871=ADVANCED_FACE ( 'NONE', ( #15026 ), #5067, .T. ) ;
#27872=EDGE_CURVE ( 'NONE', #14808, #28206, #16634, .T. ) ;
#27875=FACE_OUTER_BOUND ( 'NONE', #990, .T. ) ;
#27876=EDGE_CURVE ( 'NONE', #27852, #91, #23609, .T. ) ;
#27882=LINE ( 'NONE', #20923, #30087 ) ;
#27885=CARTESIAN_POINT ( 'NONE',  ( 58.66133336607612137, -0.9657121834148485462, -1.607522887371789722 ) ) ;
#27891=EDGE_CURVE ( 'NONE', #27064, #67, #12329, .T. ) ;
#27896=CARTESIAN_POINT ( 'NONE',  ( 51.25000000000002842, -1.487499999999464029, 1.821662113731689224E-16 ) ) ;
#27901=EDGE_LOOP ( 'NONE', ( #2471, #21405, #18979, #12241, #11300, #7703 ) ) ;
#27908=FACE_OUTER_BOUND ( 'NONE', #23076, .T. ) ;
#27910=DIRECTION ( 'NONE',  ( -0.5633368246415004776, -0.8262273428075539439, 0.000000000000000000 ) ) ;
#27918=CARTESIAN_POINT ( 'NONE',  ( 50.55258015808398397, -0.05185913279167173734, 1.177580158083963324 ) ) ;
#27919=DIRECTION ( 'NONE',  ( 0.000000000000000000, 0.000000000000000000, 1.000000000000000000 ) ) ;
#27921=FACE_OUTER_BOUND ( 'NONE', #25643, .T. ) ;
#27929=ORIENTED_EDGE ( 'NONE', *, *, #4581, .T. ) ;
#27933=CARTESIAN_POINT ( 'NONE',  ( 58.75000000000003553, -1.749295403804336013, 0.8980135333491227057 ) ) ;
#27934=ORIENTED_EDGE ( 'NONE', *, *, #3153, .T. ) ;
#27942=CARTESIAN_POINT ( 'NONE',  ( 51.16322638839886849, -0.9520444587745244824, 1.480281041496170902 ) ) ;
#27947=CARTESIAN_POINT ( 'NONE',  ( 58.65000000000004121, -1.972190280207337443, -0.1053114364790862928 ) ) ;
#27948=DIRECTION ( 'NONE',  ( 1.000000000000000000, 1.047444401652940007E-14, 0.000000000000000000 ) ) ;
#27951=CARTESIAN_POINT ( 'NONE',  ( 58.65000000000000568, 1.394635017528131904, 1.253243060178682144 ) ) ;
#27953=AXIS2_PLACEMENT_3D ( 'NONE', #3122, #27193, #7863 ) ;
#27955=CARTESIAN_POINT ( 'NONE',  ( 52.20711756518981872, -0.7499999999994703126, -1.718465885608432941 ) ) ;
#27957=ORIENTED_EDGE ( 'NONE', *, *, #25683, .F. ) ;
#27959=DIRECTION ( 'NONE',  ( 0.000000000000000000, 0.000000000000000000, 1.000000000000000000 ) ) ;
#27964=DIRECTION ( 'NONE',  ( 0.000000000000000000, 0.000000000000000000, 1.000000000000000000 ) ) ;
#27965=ORIENTED_EDGE ( 'NONE', *, *, #19183, .F. ) ;
#27976=CARTESIAN_POINT ( 'NONE',  ( 58.75000000000003553, -1.470078920827915470, 1.470078920827824209 ) ) ;
#27978=CIRCLE ( 'NONE', #9774, 0.1499999999999999667 ) ;
#27981=ADVANCED_FACE ( 'NONE', ( #24069 ), #12656, .F. ) ;
#27992=CARTESIAN_POINT ( 'NONE',  ( 58.74999999305994436, 1.683452862813316742, 0.9423072185569032477 ) ) ;
#27993=ORIENTED_EDGE ( 'NONE', *, *, #25304, .F. ) ;
#27999=ORIENTED_EDGE ( 'NONE', *, *, #10907, .F. ) ;
#28003=CARTESIAN_POINT ( 'NONE',  ( 50.25000000000003553, -1.499837071478530071, 1.323060376181713016 ) ) ;
#28012=VERTEX_POINT ( 'NONE', #13727 ) ;
#28024=LINE ( 'NONE', #30550, #3885 ) ;
#28028=DIRECTION ( 'NONE',  ( 0.000000000000000000, 0.000000000000000000, 1.000000000000000000 ) ) ;
#28032=EDGE_LOOP ( 'NONE', ( #822, #14119, #1660, #401 ) ) ;
#28042=ORIENTED_EDGE ( 'NONE', *, *, #16973, .F. ) ;
#28044=EDGE_CURVE ( 'NONE', #29648, #31291, #20738, .T. ) ;
#28050=EDGE_CURVE ( 'NONE', #2387, #27521, #23135, .T. ) ;
#28052=VERTEX_POINT ( 'NONE', #9000 ) ;
#28055=DIRECTION ( 'NONE',  ( 0.000000000000000000, 0.000000000000000000, 1.000000000000000000 ) ) ;
#28056=DIRECTION ( 'NONE',  ( 1.000000000000000000, 1.047444401652940007E-14, 0.000000000000000000 ) ) ;
#28062=FILL_AREA_STYLE_COLOUR ( '', #27122 ) ;
#28064=CARTESIAN_POINT ( 'NONE',  ( 58.75000000000002842, -1.039502773796971091, 1.800471618824829756 ) ) ;
#28067=AXIS2_PLACEMENT_3D ( 'NONE', #10916, #3787, #23283 ) ;
#28068=DIRECTION ( 'NONE',  ( 0.000000000000000000, 0.000000000000000000, 1.000000000000000000 ) ) ;
#28069=ORIENTED_EDGE ( 'NONE', *, *, #20283, .F. ) ;
#28073=DIRECTION ( 'NONE',  ( 0.000000000000000000, 0.000000000000000000, 1.000000000000000000 ) ) ;
#28079=VECTOR ( 'NONE', #806, 1000.000000000000000 ) ;
#28080=CARTESIAN_POINT ( 'NONE',  ( 58.65000000000001990, 6.143261415694495821E-13, 3.111507638930570854E-58 ) ) ;
#28084=CARTESIAN_POINT ( 'NONE',  ( 51.31757909864145972, 1.004435980686513963, -1.391945786376508343 ) ) ;
#28095=AXIS2_PLACEMENT_3D ( 'NONE', #9470, #7088, #6611 ) ;
#28100=EDGE_CURVE ( 'NONE', #27455, #14166, #21116, .T. ) ;
#28105=AXIS2_PLACEMENT_3D ( 'NONE', #4083, #28467, #13723 ) ;
#28112=CIRCLE ( 'NONE', #20041, 2.000000000000000000 ) ;
#28115=CARTESIAN_POINT ( 'NONE',  ( 61.25000000000002132, 6.415596960124259844E-13, 3.111507638930570854E-58 ) ) ;
#28124=LINE ( 'NONE', #25287, #5811 ) ;
#28128=ORIENTED_EDGE ( 'NONE', *, *, #5393, .F. ) ;
#28129=CYLINDRICAL_SURFACE ( 'NONE', #19145, 0.1500000000000001887 ) ;
#28131=EDGE_CURVE ( 'NONE', #27840, #16066, #10985, .T. ) ;
#28132=CARTESIAN_POINT ( 'NONE',  ( 61.09423418604154676, -0.6373668173473425735, 1.895722432253304168 ) ) ;
#28134=DIRECTION ( 'NONE',  ( 0.000000000000000000, 0.000000000000000000, 1.000000000000000000 ) ) ;
#28136=CARTESIAN_POINT ( 'NONE',  ( 51.17950113889409636, -0.9670426259150803894, -1.523577707254206715 ) ) ;
#28140=AXIS2_PLACEMENT_3D ( 'NONE', #17521, #1050, #10381 ) ;
#28147=EDGE_CURVE ( 'NONE', #23567, #21339, #11210, .T. ) ;
#28149=AXIS2_PLACEMENT_3D ( 'NONE', #14335, #1998, #13846 ) ;
#28153=CARTESIAN_POINT ( 'NONE',  ( 58.65000045311410304, 1.580645149931350080, 1.008695754911069331 ) ) ;
#28154=VECTOR ( 'NONE', #21558, 1000.000000000000000 ) ;
#28156=CARTESIAN_POINT ( 'NONE',  ( 58.65000000000002700, -0.5811678240976775323, -1.782657835994575724 ) ) ;
#28158=DIRECTION ( 'NONE',  ( 0.000000000000000000, 0.000000000000000000, 1.000000000000000000 ) ) ;
#28168=ADVANCED_FACE ( 'NONE', ( #21843 ), #28938, .F. ) ;
#28171=EDGE_CURVE ( 'NONE', #12544, #29950, #10495, .T. ) ;
#28172=CARTESIAN_POINT ( 'NONE',  ( 58.75000000000000711, 0.8897917884447026360, -1.791164585742097914 ) ) ;
#28174=B_SPLINE_CURVE_WITH_KNOTS ( 'NONE', 3,
 ( #2741, #17311, #5263, #22233 ),
 .UNSPECIFIED., .F., .F.,
 ( 4, 4 ),
 ( 0.0001159639600966503627, 0.0002000540139215557138 ),
 .UNSPECIFIED. ) ;
#28189=AXIS2_PLACEMENT_3D ( 'NONE', #28294, #2156, #6751 ) ;
#28201=CARTESIAN_POINT ( 'NONE',  ( 58.75000000000000711, 1.106298139390812452, -1.666164585742097914 ) ) ;
#28203=CARTESIAN_POINT ( 'NONE',  ( 58.73379417893117704, 1.830385781110580590, 0.4072049916502743505 ) ) ;
#28206=VERTEX_POINT ( 'NONE', #31313 ) ;
#28214=EDGE_CURVE ( 'NONE', #21983, #28408, #25646, .T. ) ;
#28216=ORIENTED_EDGE ( 'NONE', *, *, #19183, .T. ) ;
#28218=DIRECTION ( 'NONE',  ( -1.387778780781445676E-14, 1.000000000000000000, 0.000000000000000000 ) ) ;
#28222=ORIENTED_EDGE ( 'NONE', *, *, #12565, .F. ) ;
#28234=SURFACE_STYLE_USAGE ( .BOTH. , #30763 ) ;
#28236=EDGE_CURVE ( 'NONE', #23320, #27840, #12011, .T. ) ;
#28238=CARTESIAN_POINT ( 'NONE',  ( 58.65266784251146959, -1.589569034372440459, -0.9945725797246820488 ) ) ;
#28251=CARTESIAN_POINT ( 'NONE',  ( 50.59602332238209499, 0.1408342061609077767, 0.7375000000000033751 ) ) ;
#28253=ORIENTED_EDGE ( 'NONE', *, *, #6511, .T. ) ;
#28254=CARTESIAN_POINT ( 'NONE',  ( 58.75000000000003553, -1.760622601995820657, 0.8948927608039445314 ) ) ;
#28266=CARTESIAN_POINT ( 'NONE',  ( 61.25000000000002842, -0.4999999999993586797, -1.807104036850122109 ) ) ;
#28267=CARTESIAN_POINT ( 'NONE',  ( 58.66118217212500952, 1.337770226786352046, 1.313877211063982253 ) ) ;
#28268=CARTESIAN_POINT ( 'NONE',  ( 61.25000000000000711, 1.323060376180939413, 1.499837071478648420 ) ) ;
#28269=CARTESIAN_POINT ( 'NONE',  ( 58.75000000000002132, -0.5811678240974700316, 1.782657835994650775 ) ) ;
#28270=CARTESIAN_POINT ( 'NONE',  ( 58.66107449606948876, -1.802323084877160086, -0.5180360531255027157 ) ) ;
#28271=EDGE_CURVE ( 'NONE', #8618, #67, #19100, .T. ) ;
#28272=COLOUR_RGB ( '', 0.08235294, 0.09019608, 0.10196078) ;
#28277=DIRECTION ( 'NONE',  ( 9.329605248950888974E-15, -1.000000000000000000, 0.000000000000000000 ) ) ;
#28278=CARTESIAN_POINT ( 'NONE',  ( 51.32030452908213647, -1.012971576473159718, 1.577980961882171185 ) ) ;
#28282=DIRECTION ( 'NONE',  ( 1.000000000000000000, 1.047444401652940007E-14, 0.000000000000000000 ) ) ;
#28294=CARTESIAN_POINT ( 'NONE',  ( 58.75000000000000711, 1.470078920827434965, 1.470078920828533420 ) ) ;
#28302=B_SPLINE_CURVE_WITH_KNOTS ( 'NONE', 3,
 ( #30960, #9275, #17288, #346, #6894, #16563 ),
 .UNSPECIFIED., .F., .F.,
 ( 4, 2, 4 ),
 ( 0.000000000000000000, 0.0001000270069599285065, 0.0002000540139198570130 ),
 .UNSPECIFIED. ) ;
#28303=FACE_OUTER_BOUND ( 'NONE', #26522, .T. ) ;
#28322=CARTESIAN_POINT ( 'NONE',  ( 58.66118217212510189, 1.632243256843118884, 0.9228675180760285146 ) ) ;
#28326=CARTESIAN_POINT ( 'NONE',  ( 58.65266784251147669, -1.372094080475589228, 1.277991457600579528 ) ) ;
#28329=CARTESIAN_POINT ( 'NONE',  ( 58.75000000000000711, 1.666164585742715420, 1.106298139391201030 ) ) ;
#28345=CARTESIAN_POINT ( 'NONE',  ( 58.65000000000003411, -1.571497941946114363, -1.022750809560766694 ) ) ;
#28347=CIRCLE ( 'NONE', #1048, 0.1499999999999999667 ) ;
#28350=CARTESIAN_POINT ( 'NONE',  ( 58.75000000000000711, 1.895722432253174938, -0.6373668173460090847 ) ) ;
#28356=CARTESIAN_POINT ( 'NONE',  ( 61.19881854997409221, -0.7436933986905437388, -1.660788881864677435 ) ) ;
#28361=FACE_OUTER_BOUND ( 'NONE', #23070, .T. ) ;
#28368=CARTESIAN_POINT ( 'NONE',  ( 58.70362814788219907, 0.5000000000006148415, 1.816403611747777980 ) ) ;
#28371=CARTESIAN_POINT ( 'NONE',  ( 58.74154451056408988, 1.872697749444274029, 0.09314201707211816617 ) ) ;
#28372=ORIENTED_EDGE ( 'NONE', *, *, #27636, .F. ) ;
#28376=ADVANCED_FACE ( 'NONE', ( #15708 ), #8108, .F. ) ;
#28381=CARTESIAN_POINT ( 'NONE',  ( 50.25000000000000711, 0.8897917884446137071, -1.791164585742097914 ) ) ;
#28385=DIRECTION ( 'NONE',  ( 1.000000000000000000, 1.047444401652940007E-14, 0.000000000000000000 ) ) ;
#28388=EDGE_CURVE ( 'NONE', #4931, #17369, #23156, .T. ) ;
#28389=SURFACE_STYLE_FILL_AREA ( #23656 ) ;
#28390=CARTESIAN_POINT ( 'NONE',  ( 51.18410987668590195, -1.003361152472067586, -1.282358977530923871 ) ) ;
#28392=CARTESIAN_POINT ( 'NONE',  ( 58.65844932252336008, -1.607045716458009865, -0.9660788770022267213 ) ) ;
#28396=EDGE_LOOP ( 'NONE', ( #11737, #954, #2223, #26360, #26201, #1551 ) ) ;
#28397=CARTESIAN_POINT ( 'NONE',  ( 51.31943556899496173, -1.088761256243092612, -1.206353010735627729 ) ) ;
#28401=VERTEX_POINT ( 'NONE', #1276 ) ;
#28402=DIRECTION ( 'NONE',  ( 1.000000000000000000, 1.047444401652940007E-14, 0.000000000000000000 ) ) ;
#28405=VERTEX_POINT ( 'NONE', #17924 ) ;
#28408=VERTEX_POINT ( 'NONE', #22694 ) ;
#28409=CARTESIAN_POINT ( 'NONE',  ( 58.65844932252308297, -1.640171707772328347, 0.9087029769947272406 ) ) ;
#28412=VERTEX_POINT ( 'NONE', #3661 ) ;
#28417=ORIENTED_EDGE ( 'NONE', *, *, #19908, .T. ) ;
#28419=DIRECTION ( 'NONE',  ( 1.000000000000000000, 1.047444401652940007E-14, 0.000000000000000000 ) ) ;
#28429=CARTESIAN_POINT ( 'NONE',  ( 58.66122797211809115, -0.9517229765811608955, 1.615588400946835534 ) ) ;
#28433=LINE ( 'NONE', #7066, #2412 ) ;
#28434=DIRECTION ( 'NONE',  ( 1.000000000000000000, 1.047444401652940007E-14, 0.000000000000000000 ) ) ;
#28440=AXIS2_PLACEMENT_3D ( 'NONE', #11656, #26370, #4671 ) ;
#28442=DIRECTION ( 'NONE',  ( 0.000000000000000000, 0.000000000000000000, 1.000000000000000000 ) ) ;
#28444=EDGE_LOOP ( 'NONE', ( #16922, #6958, #21481, #10606 ) ) ;
#28455=CARTESIAN_POINT ( 'NONE',  ( 58.74999999305993725, 1.856692759305444529, -0.5240691109005866100 ) ) ;
#28456=EDGE_CURVE ( 'NONE', #25278, #14364, #1877, .T. ) ;
#28458=CARTESIAN_POINT ( 'NONE',  ( 51.12687253673779253, 0.9194130538826112975, -1.491219977510798378 ) ) ;
#28467=DIRECTION ( 'NONE',  ( 8.860386339788720432E-15, -0.8459051693633012903, -0.5333333333333335480 ) ) ;
#28469=FACE_OUTER_BOUND ( 'NONE', #21458, .T. ) ;
#28470=CARTESIAN_POINT ( 'NONE',  ( 58.75000000000002132, 6.153735859711025284E-13, 3.111507638930570854E-58 ) ) ;
#28477=CARTESIAN_POINT ( 'NONE',  ( 50.50000000000002132, 5.291762632692320630E-13, 3.111507638930570854E-58 ) ) ;
#28480=EDGE_LOOP ( 'NONE', ( #29760, #19430, #14120, #23168 ) ) ;
#28481=CARTESIAN_POINT ( 'NONE',  ( 61.25000000000001421, 1.039502773797226221, -1.800471618823823450 ) ) ;
#28491=EDGE_CURVE ( 'NONE', #9827, #6367, #21897, .T. ) ;
#28495=ORIENTED_EDGE ( 'NONE', *, *, #16679, .F. ) ;
#28498=CARTESIAN_POINT ( 'NONE',  ( 58.75000000000002132, 6.153735859711025284E-13, 3.111507638930570854E-58 ) ) ;
#28502=CARTESIAN_POINT ( 'NONE',  ( 51.64333574538936489, -0.8318165372340007302, 1.569663068107119974 ) ) ;
#28503=CARTESIAN_POINT ( 'NONE',  ( 58.72419296898095098, -1.799118770101062026, -0.5284032650186377689 ) ) ;
#28505=CIRCLE ( 'NONE', #19862, 2.000000000000000000 ) ;
#28509=ORIENTED_EDGE ( 'NONE', *, *, #12165, .F. ) ;
#28510=DIRECTION ( 'NONE',  ( 1.000000000000000000, 1.047444401652940007E-14, 0.000000000000000000 ) ) ;
#28511=DIRECTION ( 'NONE',  ( 0.000000000000000000, 0.000000000000000000, 1.000000000000000000 ) ) ;
#28514=CARTESIAN_POINT ( 'NONE',  ( 51.31572262954152563, 1.002608958138273554, -1.584424273060082378 ) ) ;
#28516=VERTEX_POINT ( 'NONE', #18718 ) ;
#28520=CARTESIAN_POINT ( 'NONE',  ( 58.71354657862811166, 0.5000000000006149525, 1.821913688936171116 ) ) ;
#28522=CARTESIAN_POINT ( 'NONE',  ( 58.74999999305994436, 1.929066554548210410, -0.02566444196698207739 ) ) ;
#28524=EDGE_CURVE ( 'NONE', #19651, #21736, #26141, .T. ) ;
#28534=VECTOR ( 'NONE', #12293, 1000.000000000000000 ) ;
#28535=CARTESIAN_POINT ( 'NONE',  ( 61.25000000000001421, 1.000000000000641709, 1.586072192556190252 ) ) ;
#28536=ADVANCED_FACE ( 'NONE', ( #28361 ), #2894, .F. ) ;
#28552=DIRECTION ( 'NONE',  ( 1.000000000000000000, 1.047444401652940007E-14, 0.000000000000000000 ) ) ;
#28555=CARTESIAN_POINT ( 'NONE',  ( 60.89332643996548455, 0.5000000000006328271, -1.718465855720773483 ) ) ;
#28561=CARTESIAN_POINT ( 'NONE',  ( 58.73371041428940487, -1.662559130997790513, 0.8671977075801986512 ) ) ;
#28564=ORIENTED_EDGE ( 'NONE', *, *, #27876, .F. ) ;
#28572=VERTEX_POINT ( 'NONE', #26773 ) ;
#28573=FACE_OUTER_BOUND ( 'NONE', #23318, .T. ) ;
#28577=CARTESIAN_POINT ( 'NONE',  ( 61.25000000000003553, -0.9999999999993586242, -1.546164609606622831 ) ) ;
#28584=CARTESIAN_POINT ( 'NONE',  ( 58.73371041428940487, -1.006219588947987686, 1.582294810367148363 ) ) ;
#28589=EDGE_CURVE ( 'NONE', #24526, #24661, #8478, .T. ) ;
#28598=DIRECTION ( 'NONE',  ( 0.000000000000000000, 0.000000000000000000, 1.000000000000000000 ) ) ;
#28614=DIRECTION ( 'NONE',  ( 1.000000000000000000, 1.047444401652940007E-14, 0.000000000000000000 ) ) ;
#28625=DIRECTION ( 'NONE',  ( 1.000000000000000000, 1.047444401652940007E-14, 0.000000000000000000 ) ) ;
#28627=B_SPLINE_CURVE_WITH_KNOTS ( 'NONE', 3,
 ( #4521, #14173, #9438, #28752, #7065, #21647, #16728, #31276, #10813, #12870, #2924, #22554, #12566 ),
 .UNSPECIFIED., .F., .F.,
 ( 4, 3, 3, 3, 4 ),
 ( 0.000000000000000000, 3.429247765842821492E-05, 6.861252194980687496E-05, 0.0001025118211733554781, 0.0001105094600589149093 ),
 .UNSPECIFIED. ) ;
#28629=DIRECTION ( 'NONE',  ( 0.000000000000000000, 0.000000000000000000, 1.000000000000000000 ) ) ;
#28637=EDGE_CURVE ( 'NONE', #14166, #12730, #5076, .T. ) ;
#28639=CARTESIAN_POINT ( 'NONE',  ( 58.75000000000001421, 1.022750809562429142, -1.571497941946046417 ) ) ;
#28647=CARTESIAN_POINT ( 'NONE',  ( 58.65000000000003411, -1.253243060178072188, 1.394635017527513510 ) ) ;
#28650=DIRECTION ( 'NONE',  ( 0.000000000000000000, 0.000000000000000000, 1.000000000000000000 ) ) ;
#28652=AXIS2_PLACEMENT_3D ( 'NONE', #21800, #19105, #14645 ) ;
#28658=CIRCLE ( 'NONE', #26614, 0.1500000000000000777 ) ;
#28660=ORIENTED_EDGE ( 'NONE', *, *, #29021, .F. ) ;
#28667=CIRCLE ( 'NONE', #27639, 2.000000000000000000 ) ;
#28679=CIRCLE ( 'NONE', #21095, 1.625000000000000222 ) ;
#28686=ORIENTED_EDGE ( 'NONE', *, *, #14110, .T. ) ;
#28699=AXIS2_PLACEMENT_3D ( 'NONE', #16613, #4406, #23263 ) ;
#28700=ORIENTED_EDGE ( 'NONE', *, *, #3638, .F. ) ;
#28708=DIRECTION ( 'NONE',  ( 0.000000000000000000, 0.000000000000000000, -1.000000000000000000 ) ) ;
#28712=AXIS2_PLACEMENT_3D ( 'NONE', #11553, #18364, #23585 ) ;
#28714=CARTESIAN_POINT ( 'NONE',  ( 51.23644008536124517, -1.080112125195908490, -1.214076932077872817 ) ) ;
#28717=ORIENTED_EDGE ( 'NONE', *, *, #11304, .T. ) ;
#28719=CARTESIAN_POINT ( 'NONE',  ( 61.00000000000003553, -0.9999999999993611777, 1.586072192556190252 ) ) ;
#28720=CARTESIAN_POINT ( 'NONE',  ( 61.09423418604154676, -0.6373668173473425735, 1.895722432253304168 ) ) ;
#28734=ORIENTED_EDGE ( 'NONE', *, *, #20532, .T. ) ;
#28743=( BOUNDED_CURVE ( )  B_SPLINE_CURVE ( 3, ( #13902, #18536, #26115, #9515 ),
 .UNSPECIFIED., .F., .T. ) 
 B_SPLINE_CURVE_WITH_KNOTS ( ( 4, 4 ),
 ( 5.439460278842602747, 5.455963239578336399 ),
 .UNSPECIFIED. ) 
 CURVE ( )  GEOMETRIC_REPRESENTATION_ITEM ( )  RATIONAL_B_SPLINE_CURVE ( ( 1.000000000000000000, 0.9999773044860189586, 0.9999773044860189586, 1.000000000000000000 ) ) 
 REPRESENTATION_ITEM ( '' )  );
#28745=B_SPLINE_CURVE_WITH_KNOTS ( 'NONE', 3,
 ( #23411, #8669, #27848, #30846, #9315, #25457 ),
 .UNSPECIFIED., .F., .F.,
 ( 4, 2, 4 ),
 ( 0.000000000000000000, 0.0001939776071359000566, 0.0003879552142718001133 ),
 .UNSPECIFIED. ) ;
#28746=ORIENTED_EDGE ( 'NONE', *, *, #29707, .T. ) ;
#28750=CARTESIAN_POINT ( 'NONE',  ( 58.75000000000000711, -0.5811678240976559939, -1.782657835994590156 ) ) ;
#28752=CARTESIAN_POINT ( 'NONE',  ( 58.72973946705038628, -0.4999999999993850475, 1.835413506854427501 ) ) ;
#28760=CARTESIAN_POINT ( 'NONE',  ( 58.74487987613195372, 0.5000000000003640421, -1.852860917432736620 ) ) ;
#28764=FACE_OUTER_BOUND ( 'NONE', #25968, .T. ) ;
#28767=VERTEX_POINT ( 'NONE', #2021 ) ;
#28773=ORIENTED_EDGE ( 'NONE', *, *, #18901, .F. ) ;
#28794=ORIENTED_EDGE ( 'NONE', *, *, #12620, .T. ) ;
#28798=CARTESIAN_POINT ( 'NONE',  ( 58.72200624034153549, 0.9564954546397702595, -1.612834625125357135 ) ) ;
#28802=DIRECTION ( 'NONE',  ( 2.150099724758698120E-15, 0.05332224631949595423, -0.9985773570672645816 ) ) ;
#28806=DIRECTION ( 'NONE',  ( 0.000000000000000000, 0.000000000000000000, 1.000000000000000000 ) ) ;
#28810=CARTESIAN_POINT ( 'NONE',  ( 61.25000000000001421, 0.9885922787763641306, 1.658880815146376753 ) ) ;
#28813=CARTESIAN_POINT ( 'NONE',  ( 50.55258015808398397, 5.293720379222080095E-13, -1.177580158083963546 ) ) ;
#28817=ORIENTED_EDGE ( 'NONE', *, *, #10252, .T. ) ;
#28822=DIRECTION ( 'NONE',  ( 1.000000000000000000, 1.047444401652940007E-14, 0.000000000000000000 ) ) ;
#28823=LINE ( 'NONE', #14394, #10965 ) ;
#28832=ORIENTED_EDGE ( 'NONE', *, *, #20337, .F. ) ;
#28833=CARTESIAN_POINT ( 'NONE',  ( 58.75000000694010538, -1.869674713775759223, 0.4751516942898563745 ) ) ;
#28844=VERTEX_POINT ( 'NONE', #25924 ) ;
#28845=CARTESIAN_POINT ( 'NONE',  ( 58.73371041428907091, 1.873417296529001908, 0.08026432063284159868 ) ) ;
#28850=ORIENTED_EDGE ( 'NONE', *, *, #4375, .T. ) ;
#28852=VERTEX_POINT ( 'NONE', #19143 ) ;
#28853=CIRCLE ( 'NONE', #4572, 2.000000000000000000 ) ;
#28863=FACE_OUTER_BOUND ( 'NONE', #13174, .T. ) ;
#28867=PLANE ( 'NONE',  #22590 ) ;
#28876=CIRCLE ( 'NONE', #12667, 2.000000000000000000 ) ;
#28877=ORIENTED_EDGE ( 'NONE', *, *, #10323, .F. ) ;
#28884=CARTESIAN_POINT ( 'NONE',  ( 51.01608411450971658, 0.7569233679480915633, 1.030722644926825859 ) ) ;
#28886=ORIENTED_EDGE ( 'NONE', *, *, #6324, .T. ) ;
#28887=DIRECTION ( 'NONE',  ( 1.000000000000000000, 1.047444401652940007E-14, 0.000000000000000000 ) ) ;
#28888=CARTESIAN_POINT ( 'NONE',  ( 51.36308620441100459, -1.097739233405182979, 1.198394850649636245 ) ) ;
#28891=CIRCLE ( 'NONE', #29896, 0.1500000000000002720 ) ;
#28892=EDGE_CURVE ( 'NONE', #2387, #23636, #19128, .T. ) ;
#28894=CARTESIAN_POINT ( 'NONE',  ( 50.59602332238209499, -0.1408342061598471806, -0.8215393206232035617 ) ) ;
#28899=CARTESIAN_POINT ( 'NONE',  ( 58.74999981404334903, -0.9032433253524316807, 1.734728236458898287 ) ) ;
#28900=CARTESIAN_POINT ( 'NONE',  ( 51.40674769956036272, 0.9873535814804794697, 1.422142864483640912 ) ) ;
#28901=DIRECTION ( 'NONE',  ( 1.000000000000000000, 1.047444401652940007E-14, 0.000000000000000000 ) ) ;
#28902=EDGE_CURVE ( 'NONE', #29235, #15307, #12516, .T. ) ;
#28903=CARTESIAN_POINT ( 'NONE',  ( 61.25000000000004263, -1.470078920827180724, -1.470078920827526892 ) ) ;
#28911=DIRECTION ( 'NONE',  ( 1.000000000000000000, 1.047444401652940007E-14, 0.000000000000000000 ) ) ;
#28913=ORIENTED_EDGE ( 'NONE', *, *, #27593, .F. ) ;
#28924=CARTESIAN_POINT ( 'NONE',  ( 51.13989201884550795, 0.9305404255935276758, -1.499649012356545796 ) ) ;
#28935=ORIENTED_EDGE ( 'NONE', *, *, #17708, .F. ) ;
#28938=CYLINDRICAL_SURFACE ( 'NONE', #30192, 0.1500000000000001887 ) ;
#28943=DIRECTION ( 'NONE',  ( 9.408669700213139918E-15, -1.000000000000000000, 0.000000000000000000 ) ) ;
#28946=VERTEX_POINT ( 'NONE', #17522 ) ;
#28947=CARTESIAN_POINT ( 'NONE',  ( 50.59602332238209499, 0.1408342061609077767, -1.125000000000000222 ) ) ;
#28948=CARTESIAN_POINT ( 'NONE',  ( 50.59602332238209499, 0.1408342061609076379, -0.8215393206232032286 ) ) ;
#28949=CYLINDRICAL_SURFACE ( 'NONE', #16076, 2.000000000000000000 ) ;
#28956=ADVANCED_FACE ( 'NONE', ( #5311 ), #10233, .F. ) ;
#28959=EDGE_CURVE ( 'NONE', #24355, #26303, #24797, .T. ) ;
#28964=FACE_OUTER_BOUND ( 'NONE', #16431, .T. ) ;
#28967=B_SPLINE_CURVE_WITH_KNOTS ( 'NONE', 3,
 ( #31189, #19475, #17112, #29423 ),
 .UNSPECIFIED., .F., .F.,
 ( 4, 4 ),
 ( 0.000000000000000000, 0.0003113238203258932740 ),
 .UNSPECIFIED. ) ;
#28971=CARTESIAN_POINT ( 'NONE',  ( 58.65000000000000568, 1.253243060177670287, 1.394635017528978782 ) ) ;
#28976=DIRECTION ( 'NONE',  ( 1.000000000000000000, 1.047444401652940007E-14, 0.000000000000000000 ) ) ;
#28978=AXIS2_PLACEMENT_3D ( 'NONE', #14325, #29217, #7531 ) ;
#28982=EDGE_CURVE ( 'NONE', #23193, #207, #22939, .T. ) ;
#28989=DIRECTION ( 'NONE',  ( 1.000000000000000000, 1.047444401652940007E-14, 0.000000000000000000 ) ) ;
#28990=B_SPLINE_CURVE_WITH_KNOTS ( 'NONE', 3,
 ( #20316, #15074, #7640, #15549 ),
 .UNSPECIFIED., .F., .F.,
 ( 4, 4 ),
 ( 0.000000000000000000, 0.0002183616642542151958 ),
 .UNSPECIFIED. ) ;
#28991=CARTESIAN_POINT ( 'NONE',  ( 51.14630318392405428, 0.9364487020640391846, 1.503522130792586342 ) ) ;
#28994=ORIENTED_EDGE ( 'NONE', *, *, #16643, .T. ) ;
#28996=FACE_OUTER_BOUND ( 'NONE', #25037, .T. ) ;
#29000=ADVANCED_FACE ( 'NONE', ( #22295 ), #20550, .T. ) ;
#29004=DIRECTION ( 'NONE',  ( 0.000000000000000000, 0.000000000000000000, 1.000000000000000000 ) ) ;
#29005=AXIS2_PLACEMENT_3D ( 'NONE', #30256, #18245, #25969 ) ;
#29006=CIRCLE ( 'NONE', #31014, 0.1500000000000001887 ) ;
#29007=DIRECTION ( 'NONE',  ( 1.000000000000000000, 1.047444401652940007E-14, 0.000000000000000000 ) ) ;
#29008=DIRECTION ( 'NONE',  ( 2.463111065593883491E-12, 0.2069455031824437852, -0.9783524716136640098 ) ) ;
#29010=PLANE ( 'NONE',  #4888 ) ;
#29013=CARTESIAN_POINT ( 'NONE',  ( 58.75000000000004263, -2.079005547593188119, 1.932245437381540134E-15 ) ) ;
#29021=EDGE_CURVE ( 'NONE', #12582, #26840, #10861, .T. ) ;
#29023=FACE_OUTER_BOUND ( 'NONE', #24206, .T. ) ;
#29024=EDGE_CURVE ( 'NONE', #28408, #16052, #21162, .T. ) ;
#29030=ORIENTED_EDGE ( 'NONE', *, *, #27308, .T. ) ;
#29044=CARTESIAN_POINT ( 'NONE',  ( 58.73371041428920591, -0.8671977075792437484, -1.662559130998595203 ) ) ;
#29049=CYLINDRICAL_SURFACE ( 'NONE', #245, 0.2500000000000000000 ) ;
#29052=CARTESIAN_POINT ( 'NONE',  ( 51.44193764627932808, 0.9752197701250188144, 1.304631266258923006 ) ) ;
#29059=CARTESIAN_POINT ( 'NONE',  ( 58.70142274306336105, 0.5000000000006148415, -1.816042500834985196 ) ) ;
#29060=ORIENTED_EDGE ( 'NONE', *, *, #3676, .F. ) ;
#29061=EDGE_CURVE ( 'NONE', #29835, #23193, #11453, .T. ) ;
#29064=FACE_OUTER_BOUND ( 'NONE', #19833, .T. ) ;
#29065=CARTESIAN_POINT ( 'NONE',  ( 50.25000000000000000, 2.008165151418512373, 0.5380862305919300592 ) ) ;
#29067=EDGE_LOOP ( 'NONE', ( #29983, #4033, #27161, #21309, #14275, #13175 ) ) ;
#29068=AXIS2_PLACEMENT_3D ( 'NONE', #23696, #16565, #23845 ) ;
#29069=CARTESIAN_POINT ( 'NONE',  ( 61.00000000000001421, 0.8666666666673054076, -1.374595900215364930 ) ) ;
#29074=ORIENTED_EDGE ( 'NONE', *, *, #23966, .F. ) ;
#29080=AXIS2_PLACEMENT_3D ( 'NONE', #30266, #16335, #7006 ) ;
#29086=CARTESIAN_POINT ( 'NONE',  ( 58.75000000000002842, -0.8948927608030052827, -1.760622601996601366 ) ) ;
#29090=CARTESIAN_POINT ( 'NONE',  ( 61.16862972101695561, -0.7079877303042131365, 1.871978752394868550 ) ) ;
#29097=ORIENTED_EDGE ( 'NONE', *, *, #10728, .T. ) ;
#29104=CARTESIAN_POINT ( 'NONE',  ( 52.20711756518982583, 0.7500000000005468959, -1.996089927833914146 ) ) ;
#29114=CIRCLE ( 'NONE', #4829, 0.2500000000000000000 ) ;
#29119=ORIENTED_EDGE ( 'NONE', *, *, #28982, .T. ) ;
#29139=EDGE_CURVE ( 'NONE', #8649, #22245, #28667, .T. ) ;
#29143=CARTESIAN_POINT ( 'NONE',  ( 51.18284667156842715, -0.9660006958939171273, -1.457928575331213894 ) ) ;
#29148=LINE ( 'NONE', #17133, #15527 ) ;
#29149=VERTEX_POINT ( 'NONE', #18595 ) ;
#29150=FACE_OUTER_BOUND ( 'NONE', #4201, .T. ) ;
#29153=CARTESIAN_POINT ( 'NONE',  ( 58.74160516400037579, -1.390091577294200631, -1.258299259017775062 ) ) ;
#29156=VERTEX_POINT ( 'NONE', #1058 ) ;
#29159=AXIS2_PLACEMENT_3D ( 'NONE', #5540, #29295, #3158 ) ;
#29166=EDGE_CURVE ( 'NONE', #26655, #15962, #11768, .T. ) ;
#29169=AXIS2_PLACEMENT_3D ( 'NONE', #25382, #1015, #3685 ) ;
#29173=DIRECTION ( 'NONE',  ( 1.000000000000000000, 1.047444401652940007E-14, 0.000000000000000000 ) ) ;
#29176=EDGE_CURVE ( 'NONE', #14207, #15114, #27137, .T. ) ;
#29177=LINE ( 'NONE', #24119, #783 ) ;
#29178=EDGE_CURVE ( 'NONE', #23320, #19132, #414, .T. ) ;
#29182=DIRECTION ( 'NONE',  ( 1.000000000000000000, 1.047444401652940007E-14, 0.000000000000000000 ) ) ;
#29194=CARTESIAN_POINT ( 'NONE',  ( 58.65000000000000568, 1.320082690053779650, 1.469015551797190788 ) ) ;
#29200=AXIS2_PLACEMENT_3D ( 'NONE', #2092, #2417, #7172 ) ;
#29207=EDGE_CURVE ( 'NONE', #7818, #19129, #26485, .T. ) ;
#29211=EDGE_CURVE ( 'NONE', #8262, #27197, #29234, .T. ) ;
#29213=DIRECTION ( 'NONE',  ( 0.000000000000000000, 0.000000000000000000, 1.000000000000000000 ) ) ;
#29214=FACE_OUTER_BOUND ( 'NONE', #10651, .T. ) ;
#29217=DIRECTION ( 'NONE',  ( 2.456447210758503401E-12, 0.9507508458638417315, -0.3099561728522108872 ) ) ;
#29220=VERTEX_POINT ( 'NONE', #21607 ) ;
#29226=AXIS2_PLACEMENT_3D ( 'NONE', #2574, #493, #10011 ) ;
#29233=( BOUNDED_CURVE ( )  B_SPLINE_CURVE ( 3, ( #14604, #17150, #21911, #24269 ),
 .UNSPECIFIED., .F., .T. ) 
 B_SPLINE_CURVE_WITH_KNOTS ( ( 4, 4 ),
 ( 1.982313172862383732, 2.241731514487931509 ),
 .UNSPECIFIED. ) 
 CURVE ( )  GEOMETRIC_REPRESENTATION_ITEM ( )  RATIONAL_B_SPLINE_CURVE ( ( 1.000000000000000000, 0.9943997021150918769, 0.9943997021150918769, 1.000000000000000000 ) ) 
 REPRESENTATION_ITEM ( '' )  );
#29234=CIRCLE ( 'NONE', #1926, 0.1500000000000000777 ) ;
#29235=VERTEX_POINT ( 'NONE', #26335 ) ;
#29238=CARTESIAN_POINT ( 'NONE',  ( 52.20711756518984714, -0.7499999999994533262, 1.718465885608438937 ) ) ;
#29246=CARTESIAN_POINT ( 'NONE',  ( 50.50000000000002132, 5.291762632692320630E-13, -1.996089927833914146 ) ) ;
#29252=CARTESIAN_POINT ( 'NONE',  ( 61.25000000000002132, 6.415596960124259844E-13, 3.111507638930570854E-58 ) ) ;
#29260=CARTESIAN_POINT ( 'NONE',  ( 52.06628335902944826, 0.5434431642986583544, -1.996089927833914146 ) ) ;
#29268=CARTESIAN_POINT ( 'NONE',  ( 58.65000000000003411, -1.671477153793625714, -0.8495817349401489915 ) ) ;
#29270=ORIENTED_EDGE ( 'NONE', *, *, #27474, .F. ) ;
#29273=CARTESIAN_POINT ( 'NONE',  ( 58.75000000000000711, 1.469015551796267305, 1.320082690054878549 ) ) ;
#29291=EDGE_CURVE ( 'NONE', #18608, #5258, #28990, .T. ) ;
#29292=CARTESIAN_POINT ( 'NONE',  ( 58.66122797211814088, -1.815363284467121252, 0.4694237433642899360 ) ) ;
#29294=DIRECTION ( 'NONE',  ( 0.000000000000000000, 0.000000000000000000, 1.000000000000000000 ) ) ;
#29295=DIRECTION ( 'NONE',  ( 1.000000000000000000, 1.047444401652940007E-14, 0.000000000000000000 ) ) ;
#29298=VERTEX_POINT ( 'NONE', #25201 ) ;
#29309=EDGE_LOOP ( 'NONE', ( #11818, #19463, #18999, #25832, #3155 ) ) ;
#29321=DIRECTION ( 'NONE',  ( 1.000000000000000000, 1.047444401652940007E-14, 0.000000000000000000 ) ) ;
#29323=CARTESIAN_POINT ( 'NONE',  ( 58.75000000000002132, 6.153735859711025284E-13, 3.111507638930570854E-58 ) ) ;
#29325=EDGE_LOOP ( 'NONE', ( #20248, #2942, #22117, #14801 ) ) ;
#29337=ADVANCED_FACE ( 'NONE', ( #30556 ), #7218, .F. ) ;
#29346=FACE_OUTER_BOUND ( 'NONE', #21111, .T. ) ;
#29350=CARTESIAN_POINT ( 'NONE',  ( 52.06628335902944826, 0.5434431642986596867, -1.718465885608439603 ) ) ;
#29353=DIRECTION ( 'NONE',  ( 1.000000000000000000, 1.047444401652940007E-14, 0.000000000000000000 ) ) ;
#29358=DIRECTION ( 'NONE',  ( 1.000000000000000000, 1.047444401652940007E-14, 0.000000000000000000 ) ) ;
#29360=CARTESIAN_POINT ( 'NONE',  ( 58.64999999999999858, 1.872332544501737361, 0.09997921184905503300 ) ) ;
#29376=LINE ( 'NONE', #10071, #12519 ) ;
#29387=DIRECTION ( 'NONE',  ( 0.000000000000000000, 0.000000000000000000, 1.000000000000000000 ) ) ;
#29392=ORIENTED_EDGE ( 'NONE', *, *, #21227, .F. ) ;
#29395=DIRECTION ( 'NONE',  ( 1.000000000000000000, 1.047444401652940007E-14, 0.000000000000000000 ) ) ;
#29399=ORIENTED_EDGE ( 'NONE', *, *, #8366, .F. ) ;
#29408=CARTESIAN_POINT ( 'NONE',  ( 58.75000000000000711, 1.323060376181323550, 1.499837071479058981 ) ) ;
#29409=AXIS2_PLACEMENT_3D ( 'NONE', #20191, #5449, #13033 ) ;
#29413=CARTESIAN_POINT ( 'NONE',  ( 52.20711756518984714, -0.6499999999994534594, -1.489337100860648189 ) ) ;
#29417=LINE ( 'NONE', #22634, #18006 ) ;
#29422=EDGE_CURVE ( 'NONE', #1939, #27496, #14998, .T. ) ;
#29423=CARTESIAN_POINT ( 'NONE',  ( 61.09423418604048095, 0.6373668173476213505, -1.895722432252298084 ) ) ;
#29430=DIRECTION ( 'NONE',  ( 0.000000000000000000, 0.000000000000000000, 1.000000000000000000 ) ) ;
#29432=CARTESIAN_POINT ( 'NONE',  ( 60.81555826527925035, 0.6500000000006364020, 1.489337100860648633 ) ) ;
#29440=CARTESIAN_POINT ( 'NONE',  ( 51.78364358464218498, 0.9002346248705929144, 1.360127766454912068 ) ) ;
#29449=EDGE_CURVE ( 'NONE', #25335, #8618, #26994, .T. ) ;
#29469=ORIENTED_EDGE ( 'NONE', *, *, #3676, .T. ) ;
#29475=ORIENTED_EDGE ( 'NONE', *, *, #10252, .F. ) ;
#29483=CARTESIAN_POINT ( 'NONE',  ( 58.75000000000002132, 6.153735859711025284E-13, 3.111507638930570854E-58 ) ) ;
#29495=DIRECTION ( 'NONE',  ( 0.000000000000000000, 0.000000000000000000, 1.000000000000000000 ) ) ;
#29502=EDGE_LOOP ( 'NONE', ( #8218, #22119, #23819, #11639 ) ) ;
#29505=ORIENTED_EDGE ( 'NONE', *, *, #23316, .T. ) ;
#29513=ORIENTED_EDGE ( 'NONE', *, *, #11983, .F. ) ;
#29522=EDGE_CURVE ( 'NONE', #8786, #24661, #20127, .T. ) ;
#29527=CARTESIAN_POINT ( 'NONE',  ( 58.75000000000000711, 1.457351493771914086, 1.320164791810606975 ) ) ;
#29529=DIRECTION ( 'NONE',  ( 1.000000000000000000, 1.047444401652940007E-14, 0.000000000000000000 ) ) ;
#29530=DIRECTION ( 'NONE',  ( 1.000000000000000000, 1.047444401652940007E-14, -0.000000000000000000 ) ) ;
#29534=CARTESIAN_POINT ( 'NONE',  ( 51.13858604272873976, -1.070913481528389166, 1.222302725805714640 ) ) ;
#29535=EDGE_CURVE ( 'NONE', #1037, #27064, #23107, .T. ) ;
#29539=CARTESIAN_POINT ( 'NONE',  ( 58.65000000000001990, 6.143261415694495821E-13, 3.111507638930570854E-58 ) ) ;
#29540=CARTESIAN_POINT ( 'NONE',  ( 51.47729133425627168, -0.9526829978892299433, -1.321356857233840110 ) ) ;
#29546=DIRECTION ( 'NONE',  ( 0.000000000000000000, 0.000000000000000000, 1.000000000000000000 ) ) ;
#29547=CIRCLE ( 'NONE', #7811, 0.1500000000000003830 ) ;
#29550=DIRECTION ( 'NONE',  ( 0.000000000000000000, 0.000000000000000000, -1.000000000000000000 ) ) ;
#29553=CARTESIAN_POINT ( 'NONE',  ( 60.89136863770560382, -0.4999999999993600119, -1.718465794862841678 ) ) ;
#29566=CARTESIAN_POINT ( 'NONE',  ( 51.78364358464229866, -0.9002346248695359821, -1.360127766454889642 ) ) ;
#29567=AXIS2_PLACEMENT_3D ( 'NONE', #21798, #29358, #15261 ) ;
#29568=ORIENTED_EDGE ( 'NONE', *, *, #28491, .T. ) ;
#29575=CIRCLE ( 'NONE', #12898, 2.000000000000000000 ) ;
#29581=EDGE_LOOP ( 'NONE', ( #20647, #16261, #10610, #21664 ) ) ;
#29589=VERTEX_POINT ( 'NONE', #13123 ) ;
#29590=CARTESIAN_POINT ( 'NONE',  ( 60.75000000000001421, 0.5000000000006363798, -1.718465885608440047 ) ) ;
#29592=CARTESIAN_POINT ( 'NONE',  ( 51.98914612709258876, 0.7788013043309388594, 1.433123603079402786 ) ) ;
#29593=ORIENTED_EDGE ( 'NONE', *, *, #22347, .F. ) ;
#29600=CARTESIAN_POINT ( 'NONE',  ( 58.65838214097827574, -1.349359547237690693, -1.301971553119712688 ) ) ;
#29608=EDGE_CURVE ( 'NONE', #4841, #20392, #16021, .T. ) ;
#29611=EDGE_CURVE ( 'NONE', #20775, #7673, #9973, .T. ) ;
#29612=AXIS2_PLACEMENT_3D ( 'NONE', #11394, #14086, #4265 ) ;
#29614=CARTESIAN_POINT ( 'NONE',  ( 51.85262340636812439, 0.6891204047495628204, 1.750401715244590095 ) ) ;
#29617=CARTESIAN_POINT ( 'NONE',  ( 58.75000000000000711, 1.800471618824943221, -1.039502773795712987 ) ) ;
#29619=VECTOR ( 'NONE', #17647, 1000.000000000000000 ) ;
#29623=AXIS2_PLACEMENT_3D ( 'NONE', #17768, #15542, #15699 ) ;
#29628=LINE ( 'NONE', #511, #10084 ) ;
#29629=DIRECTION ( 'NONE',  ( -0.5633368246415186853, 0.8262273428075416204, 0.000000000000000000 ) ) ;
#29633=ADVANCED_FACE ( 'NONE', ( #6020 ), #2127, .F. ) ;
#29634=VECTOR ( 'NONE', #21578, 1000.000000000000000 ) ;
#29636=CARTESIAN_POINT ( 'NONE',  ( 51.16541527693603797, 0.9540616519818778674, -1.477274982328775854 ) ) ;
#29642=FILL_AREA_STYLE ('',( #13021 ) ) ;
#29646=AXIS2_PLACEMENT_3D ( 'NONE', #29323, #29173, #5247 ) ;
#29648=VERTEX_POINT ( 'NONE', #23740 ) ;
#29649=CARTESIAN_POINT ( 'NONE',  ( 61.25000000000003553, -0.9999999999993586242, 1.586072192556190252 ) ) ;
#29655=CIRCLE ( 'NONE', #27649, 1.875000000000001776 ) ;
#29657=FACE_OUTER_BOUND ( 'NONE', #7820, .T. ) ;
#29658=LINE ( 'NONE', #15255, #29619 ) ;
#29659=FACE_OUTER_BOUND ( 'NONE', #2231, .T. ) ;
#29671=ORIENTED_EDGE ( 'NONE', *, *, #21938, .T. ) ;
#29672=CARTESIAN_POINT ( 'NONE',  ( 52.15659655364830627, 0.5000000000005454526, 1.807104036850122331 ) ) ;
#29674=AXIS2_PLACEMENT_3D ( 'NONE', #20769, #1121, #13283 ) ;
#29680=FACE_OUTER_BOUND ( 'NONE', #9700, .T. ) ;
#29685=ORIENTED_EDGE ( 'NONE', *, *, #935, .F. ) ;
#29693=AXIS2_PLACEMENT_3D ( 'NONE', #10865, #30341, #10715 ) ;
#29706=EDGE_CURVE ( 'NONE', #11180, #28767, #3909, .T. ) ;
#29707=EDGE_CURVE ( 'NONE', #6274, #17902, #21642, .T. ) ;
#29711=AXIS2_PLACEMENT_3D ( 'NONE', #8901, #18130, #1018 ) ;
#29713=VECTOR ( 'NONE', #19313, 1000.000000000000000 ) ;
#29731=VERTEX_POINT ( 'NONE', #136 ) ;
#29735=CARTESIAN_POINT ( 'NONE',  ( 58.66118217212530794, 1.615348343402911446, -0.9521303665439364572 ) ) ;
#29739=DIRECTION ( 'NONE',  ( 0.000000000000000000, -1.000000000000000000, 0.000000000000000000 ) ) ;
#29744=EDGE_CURVE ( 'NONE', #9733, #27521, #4900, .T. ) ;
#29747=DIRECTION ( 'NONE',  ( 1.000000000000000000, 1.047444401652940007E-14, 0.000000000000000000 ) ) ;
#29750=CARTESIAN_POINT ( 'NONE',  ( 51.59739104186226655, 1.165722629542050193, -1.468576096419531352 ) ) ;
#29752=ORIENTED_EDGE ( 'NONE', *, *, #10979, .F. ) ;
#29754=ORIENTED_EDGE ( 'NONE', *, *, #26976, .T. ) ;
#29759=VECTOR ( 'NONE', #28511, 1000.000000000000000 ) ;
#29760=ORIENTED_EDGE ( 'NONE', *, *, #27412, .T. ) ;
#29768=EDGE_CURVE ( 'NONE', #10001, #2526, #4404, .T. ) ;
#29770=CARTESIAN_POINT ( 'NONE',  ( 58.74999981196286569, -1.321459237640645767, -1.441661833134718407 ) ) ;
#29782=CARTESIAN_POINT ( 'NONE',  ( 58.75000000000004263, -1.932246131436200942, -0.4087173687850521042 ) ) ;
#29786=CARTESIAN_POINT ( 'NONE',  ( 58.66107449606992219, 1.819875603894975491, -0.4525291603547138553 ) ) ;
#29797=CARTESIAN_POINT ( 'NONE',  ( 50.55258015808398397, 5.293720379222080095E-13, -1.177580158083963546 ) ) ;
#29803=EDGE_CURVE ( 'NONE', #17369, #91, #8446, .T. ) ;
#29805=CARTESIAN_POINT ( 'NONE',  ( 58.66133336607637716, 1.607522887372764941, -0.9657121834148668649 ) ) ;
#29812=ORIENTED_EDGE ( 'NONE', *, *, #10793, .F. ) ;
#29817=AXIS2_PLACEMENT_3D ( 'NONE', #9257, #3708, #1335 ) ;
#29828=VECTOR ( 'NONE', #11037, 1000.000000000000000 ) ;
#29830=CARTESIAN_POINT ( 'NONE',  ( 58.74999999305994436, 1.345908541130588221, -1.382203543031251813 ) ) ;
#29832=ORIENTED_EDGE ( 'NONE', *, *, #12025, .F. ) ;
#29834=CIRCLE ( 'NONE', #19288, 2.000000000000000000 ) ;
#29835=VERTEX_POINT ( 'NONE', #7714 ) ;
#29850=DIRECTION ( 'NONE',  ( 0.000000000000000000, 0.000000000000000000, -1.000000000000000000 ) ) ;
#29851=EDGE_LOOP ( 'NONE', ( #7367, #21232, #13380, #30596 ) ) ;
#29857=EDGE_CURVE ( 'NONE', #15552, #10800, #18039, .T. ) ;
#29860=CARTESIAN_POINT ( 'NONE',  ( 61.00000000000002132, 6.389410850082937196E-13, 3.111507638930570854E-58 ) ) ;
#29865=FACE_OUTER_BOUND ( 'NONE', #6876, .T. ) ;
#29866=ORIENTED_EDGE ( 'NONE', *, *, #5040, .T. ) ;
#29867=B_SPLINE_CURVE_WITH_KNOTS ( 'NONE', 3,
 ( #18077, #23290, #11233, #20909 ),
 .UNSPECIFIED., .F., .F.,
 ( 4, 4 ),
 ( 5.935267624065755708E-05, 0.0002061672048306634642 ),
 .UNSPECIFIED. ) ;
#29869=DIRECTION ( 'NONE',  ( 0.000000000000000000, 0.000000000000000000, 1.000000000000000000 ) ) ;
#29874=CARTESIAN_POINT ( 'NONE',  ( 58.65000000000001990, 6.143261415694495821E-13, 3.111507638930570854E-58 ) ) ;
#29875=DIRECTION ( 'NONE',  ( 1.000000000000000000, 1.047444401652940007E-14, 0.000000000000000000 ) ) ;
#29877=FACE_OUTER_BOUND ( 'NONE', #16098, .T. ) ;
#29878=LINE ( 'NONE', #22616, #29828 ) ;
#29882=ADVANCED_FACE ( 'NONE', ( #29877 ), #5170, .T. ) ;
#29889=CARTESIAN_POINT ( 'NONE',  ( 50.75360625943720549, -0.3719558471739982108, 1.344678919698702568 ) ) ;
#29891=CARTESIAN_POINT ( 'NONE',  ( 58.75000018803716983, 1.701355787207877501, -0.9251739982193851741 ) ) ;
#29895=VERTEX_POINT ( 'NONE', #16104 ) ;
#29896=AXIS2_PLACEMENT_3D ( 'NONE', #12923, #18179, #29546 ) ;
#29903=CARTESIAN_POINT ( 'NONE',  ( 58.65000000000004121, -1.872332544500628915, 0.09997921184680889917 ) ) ;
#29904=ORIENTED_EDGE ( 'NONE', *, *, #16997, .F. ) ;
#29905=AXIS2_PLACEMENT_3D ( 'NONE', #11644, #21322, #30952 ) ;
#29907=EDGE_LOOP ( 'NONE', ( #21002, #5477, #2117, #30608 ) ) ;
#29914=AXIS2_PLACEMENT_3D ( 'NONE', #3922, #23252, #30203 ) ;
#29925=CARTESIAN_POINT ( 'NONE',  ( 58.72204580543404262, -1.341784641881615725, -1.309860786662260024 ) ) ;
#29926=( BOUNDED_SURFACE ( )  B_SPLINE_SURFACE ( 3, 2, ( 
 ( #3608, #3750, #10261 ),
 ( #3464, #20409, #5669 ),
 ( #755, #25444, #19932 ),
 ( #8349, #25296, #30199 ),
 ( #5827, #10417, #29735 ),
 ( #8048, #5515, #7878 ),
 ( #29891, #8202, #17718 ),
 ( #8514, #1216, #15484 ),
 ( #18024, #13243, #13099 ),
 ( #27360, #24968, #27676 ) ),
 .UNSPECIFIED., .F., .F., .F. ) 
 B_SPLINE_SURFACE_WITH_KNOTS ( ( 4, 2, 2, 2, 4 ),
 ( 3, 3 ),
 ( 0.0001706658715691184651, 0.0002229276920778214721, 0.0002751895125865245063, 0.0003274513330952275405, 0.0003797131536039305747 ),
 ( 0.000000000000000000, 1.000000000000000000 ),
 .UNSPECIFIED. ) 
 GEOMETRIC_REPRESENTATION_ITEM ( )  RATIONAL_B_SPLINE_SURFACE ( (
 ( 1.000000000000000000, 0.7071067811865455743, 1.000000000000000000),
 ( 1.000000000000000000, 0.7375607040701674944, 1.000000000000000000),
 ( 1.000000000000000000, 0.7730431127431096616, 1.000000000000000000),
 ( 1.000000000000000000, 0.8321012486992810375, 1.000000000000000000),
 ( 1.000000000000000000, 0.8541932017417851464, 1.000000000000000000),
 ( 1.000000000000000000, 0.8545723906072691944, 1.000000000000000000),
 ( 1.000000000000000000, 0.8327032135053918926, 1.000000000000000000),
 ( 1.000000000000000000, 0.7734559727069735269, 1.000000000000000000),
 ( 1.000000000000000000, 0.7377766653994330959, 1.000000000000000000),
 ( 1.000000000000000000, 0.7071067811865439090, 1.000000000000000000) ) ) 
 REPRESENTATION_ITEM ( '' )  SURFACE ( )  );
#29927=EDGE_LOOP ( 'NONE', ( #28794, #17456, #24243, #5949, #29568, #25074, #11584, #27058, #1401, #2849, #26202, #28686, #21052, #23983, #5156, #12585, #26093, #11214, #5287, #15177, #26035, #14680, #26904, #26387, #30050, #7648, #19787, #17363, #382, #17976, #8153, #14767 ) ) ;
#29936=CARTESIAN_POINT ( 'NONE',  ( 58.66122797211827589, -1.806862593128205630, -0.5011487553405924444 ) ) ;
#29937=ADVANCED_FACE ( 'NONE', ( #18481 ), #22775, .T. ) ;
#29942=EDGE_LOOP ( 'NONE', ( #25676, #25207, #25838, #29074 ) ) ;
#29943=CARTESIAN_POINT ( 'NONE',  ( 50.25000000000003553, -1.323060376181892872, 1.499837071478349326 ) ) ;
#29944=ADVANCED_FACE ( 'NONE', ( #8337 ), #22917, .T. ) ;
#29950=VERTEX_POINT ( 'NONE', #6132 ) ;
#29955=CARTESIAN_POINT ( 'NONE',  ( 51.18805119203790355, 0.9696852903241819366, -1.451974857136960395 ) ) ;
#29960=VERTEX_POINT ( 'NONE', #30486 ) ;
#29965=CARTESIAN_POINT ( 'NONE',  ( 61.25000000000000711, 1.470078920828157498, -1.320078920826817992 ) ) ;
#29969=CARTESIAN_POINT ( 'NONE',  ( 60.75000000000001421, 0.5000000000006363798, -1.546164609606622831 ) ) ;
#29973=ADVANCED_FACE ( 'NONE', ( #28764 ), #11508, .T. ) ;
#29977=CARTESIAN_POINT ( 'NONE',  ( 58.75000000000003553, -1.760622601995821102, 0.8948927608039443093 ) ) ;
#29981=VERTEX_POINT ( 'NONE', #6598 ) ;
#29983=ORIENTED_EDGE ( 'NONE', *, *, #28388, .T. ) ;
#29984=ORIENTED_EDGE ( 'NONE', *, *, #6230, .F. ) ;
#29991=VERTEX_POINT ( 'NONE', #23535 ) ;
#29992=CARTESIAN_POINT ( 'NONE',  ( 61.00000000000001421, 0.8666666666673055186, 1.374595900215364930 ) ) ;
#29996=FACE_OUTER_BOUND ( 'NONE', #5815, .T. ) ;
#30003=CARTESIAN_POINT ( 'NONE',  ( 58.66120520918118331, -0.4851952615757724185, 1.811135157337471879 ) ) ;
#30004=DIRECTION ( 'NONE',  ( 4.730068669893459805E-15, -0.4531102586349080030, -0.8914544820235112965 ) ) ;
#30010=B_SPLINE_CURVE_WITH_KNOTS ( 'NONE', 3,
 ( #25744, #18633, #25894, #13834, #19732, #17490, #26518, #398, #14649, #90, #21950, #17192, #22104 ),
 .UNSPECIFIED., .F., .F.,
 ( 4, 3, 3, 3, 4 ),
 ( 0.000000000000000000, 4.994367907428545029E-05, 9.982969917211881056E-05, 0.0001505119896697729815, 0.0001857353029103987188 ),
 .UNSPECIFIED. ) ;
#30013=CARTESIAN_POINT ( 'NONE',  ( 51.19148447764912646, -0.9872860527319672341, -1.295557643792433433 ) ) ;
#30019=DIRECTION ( 'NONE',  ( 0.000000000000000000, 0.000000000000000000, 1.000000000000000000 ) ) ;
#30028=DIRECTION ( 'NONE',  ( 0.000000000000000000, 1.000000000000000000, 0.000000000000000000 ) ) ;
#30034=CARTESIAN_POINT ( 'NONE',  ( 58.75000000000002132, 6.153735859711025284E-13, 3.111507638930570854E-58 ) ) ;
#30046=EDGE_CURVE ( 'NONE', #19199, #27197, #30686, .T. ) ;
#30048=FACE_OUTER_BOUND ( 'NONE', #6401, .T. ) ;
#30050=ORIENTED_EDGE ( 'NONE', *, *, #8366, .T. ) ;
#30054=DIRECTION ( 'NONE',  ( 1.000000000000000000, 1.047444401652940007E-14, 0.000000000000000000 ) ) ;
#30060=ADVANCED_FACE ( 'NONE', ( #11973 ), #6745, .T. ) ;
#30067=AXIS2_PLACEMENT_3D ( 'NONE', #26212, #9436, #18630 ) ;
#30070=VECTOR ( 'NONE', #27786, 1000.000000000000000 ) ;
#30075=CARTESIAN_POINT ( 'NONE',  ( 51.23644008536121675, 1.080112125196981410, -1.214076932077873039 ) ) ;
#30079=CARTESIAN_POINT ( 'NONE',  ( 58.75000018595672913, -1.883137918659851806, -0.4528999722754138424 ) ) ;
#30080=B_SPLINE_CURVE_WITH_KNOTS ( 'NONE', 3,
 ( #2277, #28888, #11941, #2450 ),
 .UNSPECIFIED., .F., .F.,
 ( 4, 4 ),
 ( 0.000000000000000000, 0.0003845111068534253374 ),
 .UNSPECIFIED. ) ;
#30083=CARTESIAN_POINT ( 'NONE',  ( 58.75000000000003553, -1.470078920827193825, -1.320078920827526758 ) ) ;
#30087=VECTOR ( 'NONE', #6510, 1000.000000000000114 ) ;
#30091=DIRECTION ( 'NONE',  ( 0.000000000000000000, 0.000000000000000000, 1.000000000000000000 ) ) ;
#30096=ADVANCED_FACE ( 'NONE', ( #18952 ), #21342, .F. ) ;
#30100=ORIENTED_EDGE ( 'NONE', *, *, #25537, .T. ) ;
#30101=DIRECTION ( 'NONE',  ( 0.7071067811865549002, -0.7071067811865402453, 8.659560562354930393E-17 ) ) ;
#30102=CARTESIAN_POINT ( 'NONE',  ( 51.59739104186227365, 1.010292945603182169, -1.272765950230260401 ) ) ;
#30108=EDGE_CURVE ( 'NONE', #15114, #4338, #15529, .T. ) ;
#30113=CARTESIAN_POINT ( 'NONE',  ( 61.16289782575175593, 0.6851579758935786302, 1.477831714898440341 ) ) ;
#30120=AXIS2_PLACEMENT_3D ( 'NONE', #21773, #4490, #31252 ) ;
#30123=ADVANCED_FACE ( 'NONE', ( #26379 ), #7222, .F. ) ;
#30128=CARTESIAN_POINT ( 'NONE',  ( 58.75000000694006275, 1.381609951798780767, -1.346330794793079155 ) ) ;
#30130=CARTESIAN_POINT ( 'NONE',  ( 50.59602332238209499, -0.1408342061598474304, 1.125000000000000888 ) ) ;
#30134=CARTESIAN_POINT ( 'NONE',  ( 58.65000000000003411, -0.9947034709615889536, 1.589751505945788956 ) ) ;
#30137=EDGE_LOOP ( 'NONE', ( #19875, #16495, #1932, #7956 ) ) ;
#30139=FACE_OUTER_BOUND ( 'NONE', #30223, .T. ) ;
#30143=TOROIDAL_SURFACE ( 'NONE', #28652, 1.975000000000001865, 0.1000000000000000056 ) ;
#30144=ORIENTED_EDGE ( 'NONE', *, *, #13783, .T. ) ;
#30146=EDGE_LOOP ( 'NONE', ( #25869, #22639, #17060, #12331 ) ) ;
#30149=CARTESIAN_POINT ( 'NONE',  ( 51.50435016707358926, 0.9265794315412880788, -1.339215852266871565 ) ) ;
#30150=VERTEX_POINT ( 'NONE', #14799 ) ;
#30164=CARTESIAN_POINT ( 'NONE',  ( 58.65838214097819048, 1.349359547238225376, 1.301971553120433001 ) ) ;
#30166=CARTESIAN_POINT ( 'NONE',  ( 58.65000000000001279, 0.5811678240991626776, -1.782657835994492457 ) ) ;
#30169=CARTESIAN_POINT ( 'NONE',  ( 51.14630318392396902, -0.9364487020628400327, 1.503522130792752209 ) ) ;
#30172=AXIS2_PLACEMENT_3D ( 'NONE', #15062, #5098, #22209 ) ;
#30175=AXIS2_PLACEMENT_3D ( 'NONE', #23014, #17951, #27293 ) ;
#30176=CARTESIAN_POINT ( 'NONE',  ( 51.38214458811558671, -1.084857585945107505, 1.209959298770751923 ) ) ;
#30185=CARTESIAN_POINT ( 'NONE',  ( 60.88854248453768747, -0.6773709096934548146, 1.477839832418263333 ) ) ;
#30192=AXIS2_PLACEMENT_3D ( 'NONE', #17083, #7707, #14361 ) ;
#30198=ADVANCED_FACE ( 'NONE', ( #29064 ), #12418, .T. ) ;
#30199=CARTESIAN_POINT ( 'NONE',  ( 58.65838214097848180, 1.606847897768966860, -0.9664062014978758164 ) ) ;
#30200=EDGE_CURVE ( 'NONE', #21439, #10001, #24154, .T. ) ;
#30203=DIRECTION ( 'NONE',  ( 0.000000000000000000, 0.000000000000000000, -1.000000000000000000 ) ) ;
#30207=CARTESIAN_POINT ( 'NONE',  ( 51.69060524974067050, -0.7995873297236903987, 1.427997211815761780 ) ) ;
#30218=CARTESIAN_POINT ( 'NONE',  ( 58.65000045311414567, -1.873226731663665712, -0.08323357347563117847 ) ) ;
#30222=CARTESIAN_POINT ( 'NONE',  ( 58.75000000000000711, 1.652350234724653477, 1.065927491745260358 ) ) ;
#30223=EDGE_LOOP ( 'NONE', ( #20974, #366, #12802, #17585 ) ) ;
#30225=CARTESIAN_POINT ( 'NONE',  ( 58.75000000000000711, 0.8948927608039201065, -1.760622601996761682 ) ) ;
#30234=DIRECTION ( 'NONE',  ( 1.000000000000000000, 1.047444401652940007E-14, 0.000000000000000000 ) ) ;
#30235=AXIS2_PLACEMENT_3D ( 'NONE', #925, #445, #10577 ) ;
#30237=B_SPLINE_CURVE_WITH_KNOTS ( 'NONE', 3,
 ( #29360, #10200, #17330, #232, #12409, #22400 ),
 .UNSPECIFIED., .F., .F.,
 ( 4, 2, 4 ),
 ( 0.000000000000000000, 0.0001000270069609034211, 0.0002000540139218068422 ),
 .UNSPECIFIED. ) ;
#30244=DIRECTION ( 'NONE',  ( 0.000000000000000000, 0.000000000000000000, 1.000000000000000000 ) ) ;
#30249=CARTESIAN_POINT ( 'NONE',  ( 50.25000000000003553, -1.470078920828004732, 1.470078920827824209 ) ) ;
#30254=CARTESIAN_POINT ( 'NONE',  ( 51.25000000000001421, 5.368152558471320595E-13, 3.111507638930570854E-58 ) ) ;
#30256=CARTESIAN_POINT ( 'NONE',  ( 58.65000000000001990, 6.143261415694495821E-13, 3.111507638930570854E-58 ) ) ;
#30259=CARTESIAN_POINT ( 'NONE',  ( 58.65000000000004121, -0.9941784314380475163, -1.590093208332685082 ) ) ;
#30262=ADVANCED_FACE ( 'NONE', ( #17053 ), #24459, .T. ) ;
#30263=FACE_OUTER_BOUND ( 'NONE', #27674, .T. ) ;
#30266=CARTESIAN_POINT ( 'NONE',  ( 58.75000000000003553, -1.470078920827206925, -1.470078920827526892 ) ) ;
#30269=CARTESIAN_POINT ( 'NONE',  ( 51.24551381660813831, -1.093420264358021532, -1.202138525661323731 ) ) ;
#30276=ORIENTED_EDGE ( 'NONE', *, *, #9715, .T. ) ;
#30277=AXIS2_PLACEMENT_3D ( 'NONE', #25068, #26408, #3403 ) ;
#30279=CARTESIAN_POINT ( 'NONE',  ( 60.75000000000001421, 0.5000000000006363798, 1.718465885608440047 ) ) ;
#30281=CARTESIAN_POINT ( 'NONE',  ( 50.50000000000002132, 5.291762632692320630E-13, -1.996089927833914146 ) ) ;
#30289=CARTESIAN_POINT ( 'NONE',  ( 61.25000000000000000, 1.800471618824969422, -1.039502773795712987 ) ) ;
#30304=ORIENTED_EDGE ( 'NONE', *, *, #20530, .T. ) ;
#30307=CARTESIAN_POINT ( 'NONE',  ( 58.73379417893125520, -1.582215608938960072, 1.006340787080793220 ) ) ;
#30308=EDGE_CURVE ( 'NONE', #23733, #22781, #2920, .T. ) ;
#30318=CARTESIAN_POINT ( 'NONE',  ( 51.23018762252620917, -0.9889900474263613184, 1.419502710324607841 ) ) ;
#30320=CARTESIAN_POINT ( 'NONE',  ( 58.66122797211841799, 1.314214529126963793, 1.337438849765042681 ) ) ;
#30321=TOROIDAL_SURFACE ( 'NONE', #4546, 1.975000000000001865, 0.1000000000000000056 ) ;
#30322=CARTESIAN_POINT ( 'NONE',  ( 51.49472959044965137, 1.070956530528825557, 1.224612562803249594 ) ) ;
#30323=AXIS2_PLACEMENT_3D ( 'NONE', #13281, #20449, #1722 ) ;
#30325=CARTESIAN_POINT ( 'NONE',  ( 58.75000000000000711, 1.470078920827434965, 1.470078920828533420 ) ) ;
#30328=CARTESIAN_POINT ( 'NONE',  ( 61.25000000000003553, -0.9999999999993586242, -1.655766640118113031 ) ) ;
#30341=DIRECTION ( 'NONE',  ( 1.000000000000000000, 1.047444401652940007E-14, 0.000000000000000000 ) ) ;
#30347=FACE_OUTER_BOUND ( 'NONE', #9507, .T. ) ;
#30350=EDGE_CURVE ( 'NONE', #20749, #7153, #1395, .T. ) ;
#30354=CARTESIAN_POINT ( 'NONE',  ( 58.65263613458538572, 1.792763816755340356, -0.5494533739919623683 ) ) ;
#30355=TOROIDAL_SURFACE ( 'NONE', #16727, 1.975000000000001865, 0.1000000000000000056 ) ;
#30363=EDGE_CURVE ( 'NONE', #4089, #28405, #389, .T. ) ;
#30365=CARTESIAN_POINT ( 'NONE',  ( 58.66122797211820483, -1.875002085569718258, -0.01642207461113097053 ) ) ;
#30367=CARTESIAN_POINT ( 'NONE',  ( 58.75000000000000711, 1.800471618824943221, -1.039502773795712987 ) ) ;
#30368=EDGE_CURVE ( 'NONE', #16027, #19841, #19125, .T. ) ;
#30381=LINE ( 'NONE', #28003, #11987 ) ;
#30385=DIRECTION ( 'NONE',  ( 0.000000000000000000, 0.000000000000000000, 1.000000000000000000 ) ) ;
#30391=DIRECTION ( 'NONE',  ( 0.000000000000000000, 0.000000000000000000, -1.000000000000000000 ) ) ;
#30392=CARTESIAN_POINT ( 'NONE',  ( 61.25000000000000000, 1.960427193528887280, -0.3958853607737569114 ) ) ;
#30395=CARTESIAN_POINT ( 'NONE',  ( 58.75000000000002132, 6.153735859711025284E-13, 3.111507638930570854E-58 ) ) ;
#30398=CARTESIAN_POINT ( 'NONE',  ( 50.25000000000000000, 1.499837071477871042, 1.323060376182421782 ) ) ;
#30405=CARTESIAN_POINT ( 'NONE',  ( 58.75000000000000000, 1.877732920581272946, 0.6121634413844393441 ) ) ;
#30411=( BOUNDED_CURVE ( )  B_SPLINE_CURVE ( 3, ( #11700, #9500, #4714, #12018 ),
 .UNSPECIFIED., .F., .T. ) 
 B_SPLINE_CURVE_WITH_KNOTS ( ( 4, 4 ),
 ( 4.094114376165666869, 4.828985806059314712 ),
 .UNSPECIFIED. ) 
 CURVE ( )  GEOMETRIC_REPRESENTATION_ITEM ( )  RATIONAL_B_SPLINE_CURVE ( ( 1.000000000000000000, 0.9555010429016489448, 0.9555010429016489448, 1.000000000000000000 ) ) 
 REPRESENTATION_ITEM ( '' )  );
#30412=EDGE_LOOP ( 'NONE', ( #26697, #5222 ) ) ;
#30415=CARTESIAN_POINT ( 'NONE',  ( 58.66107449606996482, 1.640741681271480124, -0.9081280691409446826 ) ) ;
#30425=B_SPLINE_CURVE_WITH_KNOTS ( 'NONE', 3,
 ( #19661, #21570, #29143, #19805, #16663, #26455, #2224, #173, #9541, #9994 ),
 .UNSPECIFIED., .F., .F.,
 ( 4, 2, 2, 2, 4 ),
 ( 2.528772284819897467E-18, 9.757673230185597056E-05, 0.0001951534646037094746, 0.0002927301969055630328, 0.0003903069292074165639 ),
 .UNSPECIFIED. ) ;
#30428=CARTESIAN_POINT ( 'NONE',  ( 58.73307976133189356, 0.5681412931396376820, -1.786904874454019465 ) ) ;
#30429=CARTESIAN_POINT ( 'NONE',  ( 52.20711756518984714, -0.7499999999994533262, -1.718465885608440935 ) ) ;
#30442=CARTESIAN_POINT ( 'NONE',  ( 58.75000000000002132, 6.153735859711025284E-13, 3.111507638930570854E-58 ) ) ;
#30443=CARTESIAN_POINT ( 'NONE',  ( 58.66133336607565241, -0.9092995659213525261, 1.640092727267363770 ) ) ;
#30446=CARTESIAN_POINT ( 'NONE',  ( 58.75000000000002132, 6.153735859711025284E-13, 3.111507638930570854E-58 ) ) ;
#30453=CARTESIAN_POINT ( 'NONE',  ( 51.19148447764911225, 0.9872860527330414859, -1.295557643792421443 ) ) ;
#30454=EDGE_CURVE ( 'NONE', #5258, #25335, #7423, .T. ) ;
#30463=LINE ( 'NONE', #3877, #30618 ) ;
#30467=CARTESIAN_POINT ( 'NONE',  ( 58.64999999999999858, 1.253243060177670287, 1.394635017528978782 ) ) ;
#30473=CYLINDRICAL_SURFACE ( 'NONE', #6433, 0.2500000000000000000 ) ;
#30474=ADVANCED_FACE ( 'NONE', ( #26420 ), #28949, .T. ) ;
#30475=CARTESIAN_POINT ( 'NONE',  ( 51.45655683570191741, -0.9591657938390834026, 1.611094652690528095 ) ) ;
#30479=EDGE_CURVE ( 'NONE', #22240, #2603, #12514, .T. ) ;
#30486=CARTESIAN_POINT ( 'NONE',  ( 61.25000000000003553, -1.039502773796089796, -1.650471618824325359 ) ) ;
#30490=LINE ( 'NONE', #24465, #15056 ) ;
#30498=CARTESIAN_POINT ( 'NONE',  ( 58.74999981196283017, 1.909245389982500818, -0.4235863532939667664 ) ) ;
#30503=ADVANCED_FACE ( 'NONE', ( #14698 ), #4419, .T. ) ;
#30504=CARTESIAN_POINT ( 'NONE',  ( 60.99941465888825576, -0.5621240721069680202, -1.858165151418244010 ) ) ;
#30508=EDGE_CURVE ( 'NONE', #24848, #1900, #27104, .T. ) ;
#30510=EDGE_CURVE ( 'NONE', #15123, #9856, #14373, .T. ) ;
#30512=DIRECTION ( 'NONE',  ( -0.5633368246415004776, -0.8262273428075539439, 0.000000000000000000 ) ) ;
#30518=AXIS2_PLACEMENT_3D ( 'NONE', #18476, #28282, #6128 ) ;
#30520=CARTESIAN_POINT ( 'NONE',  ( 58.74154451056426751, -1.390058629627632936, 1.258335925860512461 ) ) ;
#30523=DIRECTION ( 'NONE',  ( 1.000000000000000000, 1.047444401652940007E-14, 0.000000000000000000 ) ) ;
#30527=ORIENTED_EDGE ( 'NONE', *, *, #3320, .T. ) ;
#30541=DIRECTION ( 'NONE',  ( 0.000000000000000000, 0.000000000000000000, 1.000000000000000000 ) ) ;
#30550=CARTESIAN_POINT ( 'NONE',  ( 52.06628335902946247, -0.5434431642975677823, -1.996089927833914146 ) ) ;
#30551=CARTESIAN_POINT ( 'NONE',  ( 60.97408713704744088, -0.7545809820792435119, 1.439897579195098309 ) ) ;
#30556=FACE_OUTER_BOUND ( 'NONE', #19008, .T. ) ;
#30566=VERTEX_POINT ( 'NONE', #29268 ) ;
#30577=EDGE_CURVE ( 'NONE', #4452, #1083, #6976, .T. ) ;
#30587=( LENGTH_UNIT ( ) NAMED_UNIT ( * ) SI_UNIT ( .MILLI., .METRE. ) );
#30590=EDGE_CURVE ( 'NONE', #6559, #20284, #17109, .T. ) ;
#30591=FACE_OUTER_BOUND ( 'NONE', #13990, .T. ) ;
#30592=( BOUNDED_SURFACE ( )  B_SPLINE_SURFACE ( 3, 2, ( 
 ( #6417, #25729, #4037 ),
 ( #29566, #13356, #23049 ),
 ( #22167, #1341, #456 ),
 ( #24677, #11014, #606 ) ),
 .UNSPECIFIED., .F., .F., .F. ) 
 B_SPLINE_SURFACE_WITH_KNOTS ( ( 4, 4 ),
 ( 3, 3 ),
 ( 4.041453792691655167, 4.300872134317203610 ),
 ( 0.000000000000000000, 1.000000000000000000 ),
 .UNSPECIFIED. ) 
 GEOMETRIC_REPRESENTATION_ITEM ( )  RATIONAL_B_SPLINE_SURFACE ( (
 ( 1.000000000000000000, 0.8699658093904940603, 1.000000000000000000),
 ( 1.000000000000000000, 0.8538860448759170163, 1.000000000000000000),
 ( 1.000000000000000000, 0.8356979842195467745, 1.000000000000000000),
 ( 1.000000000000000000, 0.8156258140602883344, 1.000000000000000000) ) ) 
 REPRESENTATION_ITEM ( '' )  SURFACE ( )  );
#30596=ORIENTED_EDGE ( 'NONE', *, *, #14517, .F. ) ;
#30606=AXIS2_PLACEMENT_3D ( 'NONE', #14715, #5361, #10124 ) ;
#30608=ORIENTED_EDGE ( 'NONE', *, *, #30577, .F. ) ;
#30610=CARTESIAN_POINT ( 'NONE',  ( 58.75000000000003553, -1.652371589363308413, 1.066009655020056845 ) ) ;
#30616=ORIENTED_EDGE ( 'NONE', *, *, #26286, .F. ) ;
#30618=VECTOR ( 'NONE', #1503, 1000.000000000000000 ) ;
#30629=CARTESIAN_POINT ( 'NONE',  ( 58.65000000000003411, -1.793030239489117994, -0.5493518053820871661 ) ) ;
#30636=CYLINDRICAL_SURFACE ( 'NONE', #28440, 2.000000000000000000 ) ;
#30639=VERTEX_POINT ( 'NONE', #16264 ) ;
#30647=VECTOR ( 'NONE', #8321, 1000.000000000000000 ) ;
#30664=PLANE ( 'NONE',  #13852 ) ;
#30671=ADVANCED_FACE ( 'NONE', ( #1531 ), #27830, .T. ) ;
#30675=CIRCLE ( 'NONE', #17049, 0.1000000000000001721 ) ;
#30683=AXIS2_PLACEMENT_3D ( 'NONE', #5082, #8083, #12659 ) ;
#30685=CARTESIAN_POINT ( 'NONE',  ( 51.24551381660811700, 1.093420264359095784, 1.202138525661322843 ) ) ;
#30686=CIRCLE ( 'NONE', #3394, 2.000000000000000000 ) ;
#30688=DIRECTION ( 'NONE',  ( 1.000000000000000000, 1.047444401652940007E-14, 0.000000000000000000 ) ) ;
#30691=AXIS2_PLACEMENT_3D ( 'NONE', #20849, #16847, #15917 ) ;
#30692=ORIENTED_EDGE ( 'NONE', *, *, #7359, .F. ) ;
#30701=CIRCLE ( 'NONE', #28189, 0.1500000000000001887 ) ;
#30702=CARTESIAN_POINT ( 'NONE',  ( 50.59602332238209499, -0.1408342061598471806, -0.8215393206232035617 ) ) ;
#30704=CARTESIAN_POINT ( 'NONE',  ( 58.65838214097809100, 0.9664062014978274107, 1.606847897768749700 ) ) ;
#30706=EDGE_LOOP ( 'NONE', ( #8292, #20922, #11483, #2775 ) ) ;
#30710=ADVANCED_FACE ( 'NONE', ( #30347 ), #28129, .F. ) ;
#30722=CARTESIAN_POINT ( 'NONE',  ( 51.21021026411726496, 1.041641720705850149, -1.248302399389048079 ) ) ;
#30737=CARTESIAN_POINT ( 'NONE',  ( 61.25000000000001421, 1.000000000000641709, -1.863080903343375061 ) ) ;
#30740=ORIENTED_EDGE ( 'NONE', *, *, #11447, .T. ) ;
#30749=CARTESIAN_POINT ( 'NONE',  ( 58.74160516400051790, 1.872695119589735668, -0.09319124196165359808 ) ) ;
#30758=DIRECTION ( 'NONE',  ( 0.000000000000000000, 0.000000000000000000, 1.000000000000000000 ) ) ;
#30759=CARTESIAN_POINT ( 'NONE',  ( 51.36308620441100459, -1.097739233405183201, -1.198394850649635801 ) ) ;
#30763=SURFACE_SIDE_STYLE ('',( #28389 ) ) ;
#30771=CARTESIAN_POINT ( 'NONE',  ( 51.02976068049119363, -1.019450805964126516, -1.268081568884226407 ) ) ;
#30776=ORIENTED_EDGE ( 'NONE', *, *, #7473, .F. ) ;
#30784=CARTESIAN_POINT ( 'NONE',  ( 51.36283714269074352, 1.001673184508090397, -1.284520656909115877 ) ) ;
#30789=DIRECTION ( 'NONE',  ( 1.000000000000000000, 1.047444401652940007E-14, 0.000000000000000000 ) ) ;
#30795=CARTESIAN_POINT ( 'NONE',  ( 52.20711756518982583, 0.7500000000005468959, 1.718465885608440491 ) ) ;
#30797=VERTEX_POINT ( 'NONE', #4541 ) ;
#30803=CARTESIAN_POINT ( 'NONE',  ( 58.75000000694009117, -0.9860766835994869695, 1.658042653848745607 ) ) ;
#30807=TOROIDAL_SURFACE ( 'NONE', #8069, 1.975000000000001865, 0.1000000000000000056 ) ;
#30808=CARTESIAN_POINT ( 'NONE',  ( 52.06628335902944826, 0.5434431642986571331, -1.794517909405660694 ) ) ;
#30811=ORIENTED_EDGE ( 'NONE', *, *, #2225, .T. ) ;
#30815=EDGE_CURVE ( 'NONE', #26954, #22739, #16492, .T. ) ;
#30818=DIRECTION ( 'NONE',  ( 1.000000000000000000, 1.047444401652940007E-14, 0.000000000000000000 ) ) ;
#30820=VERTEX_POINT ( 'NONE', #11672 ) ;
#30828=EDGE_LOOP ( 'NONE', ( #27929, #5770, #29475, #24012, #25315, #13710 ) ) ;
#30834=AXIS2_PLACEMENT_3D ( 'NONE', #19514, #5095, #24405 ) ;
#30840=DIRECTION ( 'NONE',  ( 0.000000000000000000, 0.000000000000000000, 1.000000000000000000 ) ) ;
#30844=ORIENTED_EDGE ( 'NONE', *, *, #11831, .T. ) ;
#30846=CARTESIAN_POINT ( 'NONE',  ( 60.88048385701372212, -0.6732112958808652570, -1.479676701994273369 ) ) ;
#30848=CARTESIAN_POINT ( 'NONE',  ( 50.59602332238209499, -0.1408342061598474304, -0.7375000000000029310 ) ) ;
#30851=CARTESIAN_POINT ( 'NONE',  ( 58.74160516400055343, 1.668397168087972116, 0.8556415768457033000 ) ) ;
#30856=DIRECTION ( 'NONE',  ( 1.000000000000000000, 1.047444401652940007E-14, 0.000000000000000000 ) ) ;
#30857=ORIENTED_EDGE ( 'NONE', *, *, #29803, .T. ) ;
#30863=CARTESIAN_POINT ( 'NONE',  ( 58.65266784251151932, 0.8793208749734084950, 1.656109637136073731 ) ) ;
#30871=ORIENTED_EDGE ( 'NONE', *, *, #17004, .T. ) ;
#30873=DIRECTION ( 'NONE',  ( 0.000000000000000000, 0.000000000000000000, 1.000000000000000000 ) ) ;
#30876=B_SPLINE_CURVE_WITH_KNOTS ( 'NONE', 3,
 ( #9180, #9329, #6789, #16777, #26106, #28647 ),
 .UNSPECIFIED., .F., .F.,
 ( 4, 2, 4 ),
 ( 0.000000000000000000, 0.0001000270069598443860, 0.0002000540139196887719 ),
 .UNSPECIFIED. ) ;
#30877=DIRECTION ( 'NONE',  ( 0.000000000000000000, 0.000000000000000000, 1.000000000000000000 ) ) ;
#30890=ADVANCED_FACE ( 'NONE', ( #29996 ), #8926, .T. ) ;
#30900=VERTEX_POINT ( 'NONE', #23207 ) ;
#30904=CARTESIAN_POINT ( 'NONE',  ( 58.75000000000000000, 1.964000600391587081, -0.09700564724573840225 ) ) ;
#30905=VERTEX_POINT ( 'NONE', #27626 ) ;
#30906=EDGE_CURVE ( 'NONE', #779, #6477, #17617, .T. ) ;
#30909=ORIENTED_EDGE ( 'NONE', *, *, #13665, .T. ) ;
#30914=CARTESIAN_POINT ( 'NONE',  ( 51.23644008536124517, -1.080112125195908490, -1.214076932077872817 ) ) ;
#30924=CARTESIAN_POINT ( 'NONE',  ( 50.59602332238209499, -0.1408342061598474859, 1.212874140286674285 ) ) ;
#30928=DIRECTION ( 'NONE',  ( -1.000000000000000000, -1.018631342913014973E-14, -0.000000000000000000 ) ) ;
#30929=DIRECTION ( 'NONE',  ( 0.000000000000000000, 0.000000000000000000, 1.000000000000000000 ) ) ;
#30931=CARTESIAN_POINT ( 'NONE',  ( 61.25000000000001421, 1.000000000000641709, 1.655766640118845112 ) ) ;
#30935=DIRECTION ( 'NONE',  ( 0.000000000000000000, 0.000000000000000000, 1.000000000000000000 ) ) ;
#30941=CARTESIAN_POINT ( 'NONE',  ( 58.75000000000003553, -1.671477153793476722, 0.8495817349404574115 ) ) ;
#30948=ORIENTED_EDGE ( 'NONE', *, *, #21596, .F. ) ;
#30952=DIRECTION ( 'NONE',  ( 0.000000000000000000, 0.8381322357048210936, -0.5454670984325618033 ) ) ;
#30954=DIRECTION ( 'NONE',  ( 0.000000000000000000, 0.000000000000000000, 1.000000000000000000 ) ) ;
#30960=CARTESIAN_POINT ( 'NONE',  ( 58.65000000000004121, -1.834410884275050169, 0.3880228184668811364 ) ) ;
#30962=CARTESIAN_POINT ( 'NONE',  ( 58.65844932252307586, -0.9660788770021814242, 1.607045716458280538 ) ) ;
#30971=CARTESIAN_POINT ( 'NONE',  ( 50.25000000000000711, 1.039502773797110979, -1.800471618823823450 ) ) ;
#30977=ORIENTED_EDGE ( 'NONE', *, *, #30046, .T. ) ;
#30982=CARTESIAN_POINT ( 'NONE',  ( 58.75000000694005564, 1.869674713775927755, -0.4751516942887533124 ) ) ;
#30987=ADVANCED_FACE ( 'NONE', ( #26198 ), #16097, .F. ) ;
#30994=EDGE_LOOP ( 'NONE', ( #8068, #10070, #14050, #28877 ) ) ;
#31003=CARTESIAN_POINT ( 'NONE',  ( 58.65000000000001990, 6.143261415694495821E-13, 3.111507638930570854E-58 ) ) ;
#31004=ORIENTED_EDGE ( 'NONE', *, *, #15859, .T. ) ;
#31008=CARTESIAN_POINT ( 'NONE',  ( 58.65000045311411014, 0.8645309767539767209, 1.663878723407761884 ) ) ;
#31012=DIRECTION ( 'NONE',  ( 1.000000000000000000, 1.047444401652940007E-14, 0.000000000000000000 ) ) ;
#31014=AXIS2_PLACEMENT_3D ( 'NONE', #18091, #27734, #28028 ) ;
#31017=CARTESIAN_POINT ( 'NONE',  ( 52.20711756518983293, 0.6500000000005468070, -1.489337100860647967 ) ) ;
#31022=CARTESIAN_POINT ( 'NONE',  ( 61.24343480274154672, 0.9192405086487059895, -1.710822371301342404 ) ) ;
#31028=CIRCLE ( 'NONE', #14842, 0.1500000000000001887 ) ;
#31031=CARTESIAN_POINT ( 'NONE',  ( 58.75000000000002132, 6.153735859711025284E-13, 3.111507638930570854E-58 ) ) ;
#31034=EDGE_CURVE ( 'NONE', #7404, #24526, #9261, .T. ) ;
#31036=LINE ( 'NONE', #18867, #29759 ) ;
#31039=DIRECTION ( 'NONE',  ( -9.329605248950888974E-15, 1.000000000000000000, 0.000000000000000000 ) ) ;
#31040=ORIENTED_EDGE ( 'NONE', *, *, #22798, .F. ) ;
#31045=CARTESIAN_POINT ( 'NONE',  ( 58.73097752866945598, 0.5000000000006151746, 1.835761897403992648 ) ) ;
#31048=ORIENTED_EDGE ( 'NONE', *, *, #28637, .T. ) ;
#31050=CARTESIAN_POINT ( 'NONE',  ( 58.75000000000003553, -1.469015551795635588, -1.320082690053874686 ) ) ;
#31063=( BOUNDED_SURFACE ( )  B_SPLINE_SURFACE ( 3, 2, ( 
 ( #9115, #28750, #6895 ),
 ( #9435, #23516, #16724 ),
 ( #19102, #21173, #6584 ),
 ( #7063, #26041, #16243 ) ),
 .UNSPECIFIED., .F., .F., .F. ) 
 B_SPLINE_SURFACE_WITH_KNOTS ( ( 4, 4 ),
 ( 3, 3 ),
 ( 0.0001706658715693129167, 0.0002755376070454402431 ),
 ( 0.000000000000000000, 1.000000000000000000 ),
 .UNSPECIFIED. ) 
 GEOMETRIC_REPRESENTATION_ITEM ( )  RATIONAL_B_SPLINE_SURFACE ( (
 ( 1.000000000000000000, 0.7071067811866784680, 1.000000000000000000),
 ( 1.000000000000000000, 0.7664791242987701869, 1.000000000000000000),
 ( 1.000000000000000000, 0.8546216002064864758, 1.000000000000000000),
 ( 1.000000000000000000, 0.8543839179689260988, 1.000000000000000000) ) ) 
 REPRESENTATION_ITEM ( '' )  SURFACE ( )  );
#31072=EDGE_LOOP ( 'NONE', ( #9298, #23460, #20556, #1421 ) ) ;
#31078=AXIS2_PLACEMENT_3D ( 'NONE', #19842, #7787, #1594 ) ;
#31079=DIRECTION ( 'NONE',  ( 0.000000000000000000, 0.3099561728525589976, -0.9507508458637281556 ) ) ;
#31092=VECTOR ( 'NONE', #29495, 1000.000000000000000 ) ;
#31099=DIRECTION ( 'NONE',  ( 1.000000000000000000, 1.047444401652940007E-14, 0.000000000000000000 ) ) ;
#31101=CARTESIAN_POINT ( 'NONE',  ( 58.66054497608116947, -0.4999999999856035160, 1.807104036853935503 ) ) ;
#31110=CARTESIAN_POINT ( 'NONE',  ( 51.13858604272871133, 1.070913481529462086, 1.222302725805713308 ) ) ;
#31118=EDGE_LOOP ( 'NONE', ( #8861, #4062, #18074, #4070 ) ) ;
#31138=CYLINDRICAL_SURFACE ( 'NONE', #5164, 0.1500000000000001887 ) ;
#31139=PLANE ( 'NONE',  #28095 ) ;
#31150=AXIS2_PLACEMENT_3D ( 'NONE', #15079, #20166, #22228 ) ;
#31152=ORIENTED_EDGE ( 'NONE', *, *, #21434, .T. ) ;
#31161=CARTESIAN_POINT ( 'NONE',  ( 58.72204580543390762, 0.9179489429356690877, -1.635081356933328456 ) ) ;
#31163=ORIENTED_EDGE ( 'NONE', *, *, #3561, .F. ) ;
#31166=VERTEX_POINT ( 'NONE', #22383 ) ;
#31172=CARTESIAN_POINT ( 'NONE',  ( 58.66122797211838247, 0.9232791089889081926, 1.632010475558724583 ) ) ;
#31178=VECTOR ( 'NONE', #543, 1000.000000000000000 ) ;
#31181=VECTOR ( 'NONE', #2880, 1000.000000000000000 ) ;
#31182=CARTESIAN_POINT ( 'NONE',  ( 51.59739104186229497, -1.165722629540969058, 1.468576096419531574 ) ) ;
#31184=TOROIDAL_SURFACE ( 'NONE', #5888, 1.975000000000001865, 0.1000000000000000056 ) ;
#31185=DIRECTION ( 'NONE',  ( -7.001079612237637714E-15, 0.6683962987619627150, -0.7438053426813424629 ) ) ;
#31187=EDGE_CURVE ( 'NONE', #23886, #20434, #24787, .T. ) ;
#31189=CARTESIAN_POINT ( 'NONE',  ( 61.23770293222991512, 0.8897917884447287262, -1.791164585742097914 ) ) ;
#31195=AXIS2_PLACEMENT_3D ( 'NONE', #17117, #27049, #22176 ) ;
#31221=CARTESIAN_POINT ( 'NONE',  ( 58.72200624034156391, 1.875003484781901930, 0.02193204975976815671 ) ) ;
#31225=CARTESIAN_POINT ( 'NONE',  ( 52.20711756518983293, 0.6500000000005468070, 1.489337100860647967 ) ) ;
#31237=CARTESIAN_POINT ( 'NONE',  ( 61.25000000000003553, -1.039502773796076474, -1.800471618824325493 ) ) ;
#31238=AXIS2_PLACEMENT_3D ( 'NONE', #595, #12625, #14699 ) ;
#31239=AXIS2_PLACEMENT_3D ( 'NONE', #21383, #24211, #11852 ) ;
#31243=VERTEX_POINT ( 'NONE', #10657 ) ;
#31252=DIRECTION ( 'NONE',  ( 0.000000000000000000, 0.3099561728515298764, 0.9507508458640635540 ) ) ;
#31253=EDGE_CURVE ( 'NONE', #30900, #29298, #21181, .T. ) ;
#31257=VERTEX_POINT ( 'NONE', #23173 ) ;
#31263=CARTESIAN_POINT ( 'NONE',  ( 58.65000000000004121, -1.872332544500605822, -0.09997921184723339294 ) ) ;
#31269=CARTESIAN_POINT ( 'NONE',  ( 52.10742184747380179, -0.5153941949037030845, -1.803012124260139126 ) ) ;
#31271=CARTESIAN_POINT ( 'NONE',  ( 58.72419296898078755, -0.8985315506022777399, -1.645806614394816458 ) ) ;
#31276=CARTESIAN_POINT ( 'NONE',  ( 58.69114869172535265, -0.4999999999993854916, 1.811349421029608608 ) ) ;
#31286=CARTESIAN_POINT ( 'NONE',  ( 58.75000000000000711, 1.960427193528805123, -0.3958853607737420899 ) ) ;
#31291=VERTEX_POINT ( 'NONE', #17795 ) ;
#31293=ORIENTED_EDGE ( 'NONE', *, *, #14355, .F. ) ;
#31307=DIRECTION ( 'NONE',  ( 0.000000000000000000, 0.000000000000000000, 1.000000000000000000 ) ) ;
#31311=ORIENTED_EDGE ( 'NONE', *, *, #21596, .T. ) ;
#31313=CARTESIAN_POINT ( 'NONE',  ( 51.12687253673779253, 0.9194130538826106314, 1.491219977510798156 ) ) ;
#31314=ORIENTED_EDGE ( 'NONE', *, *, #19429, .T. ) ;
#31320=CARTESIAN_POINT ( 'NONE',  ( 58.66122797211883011, 0.9517229765820151011, -1.615588400947058911 ) ) ;
ENDSEC;
END-ISO-10303-21;
